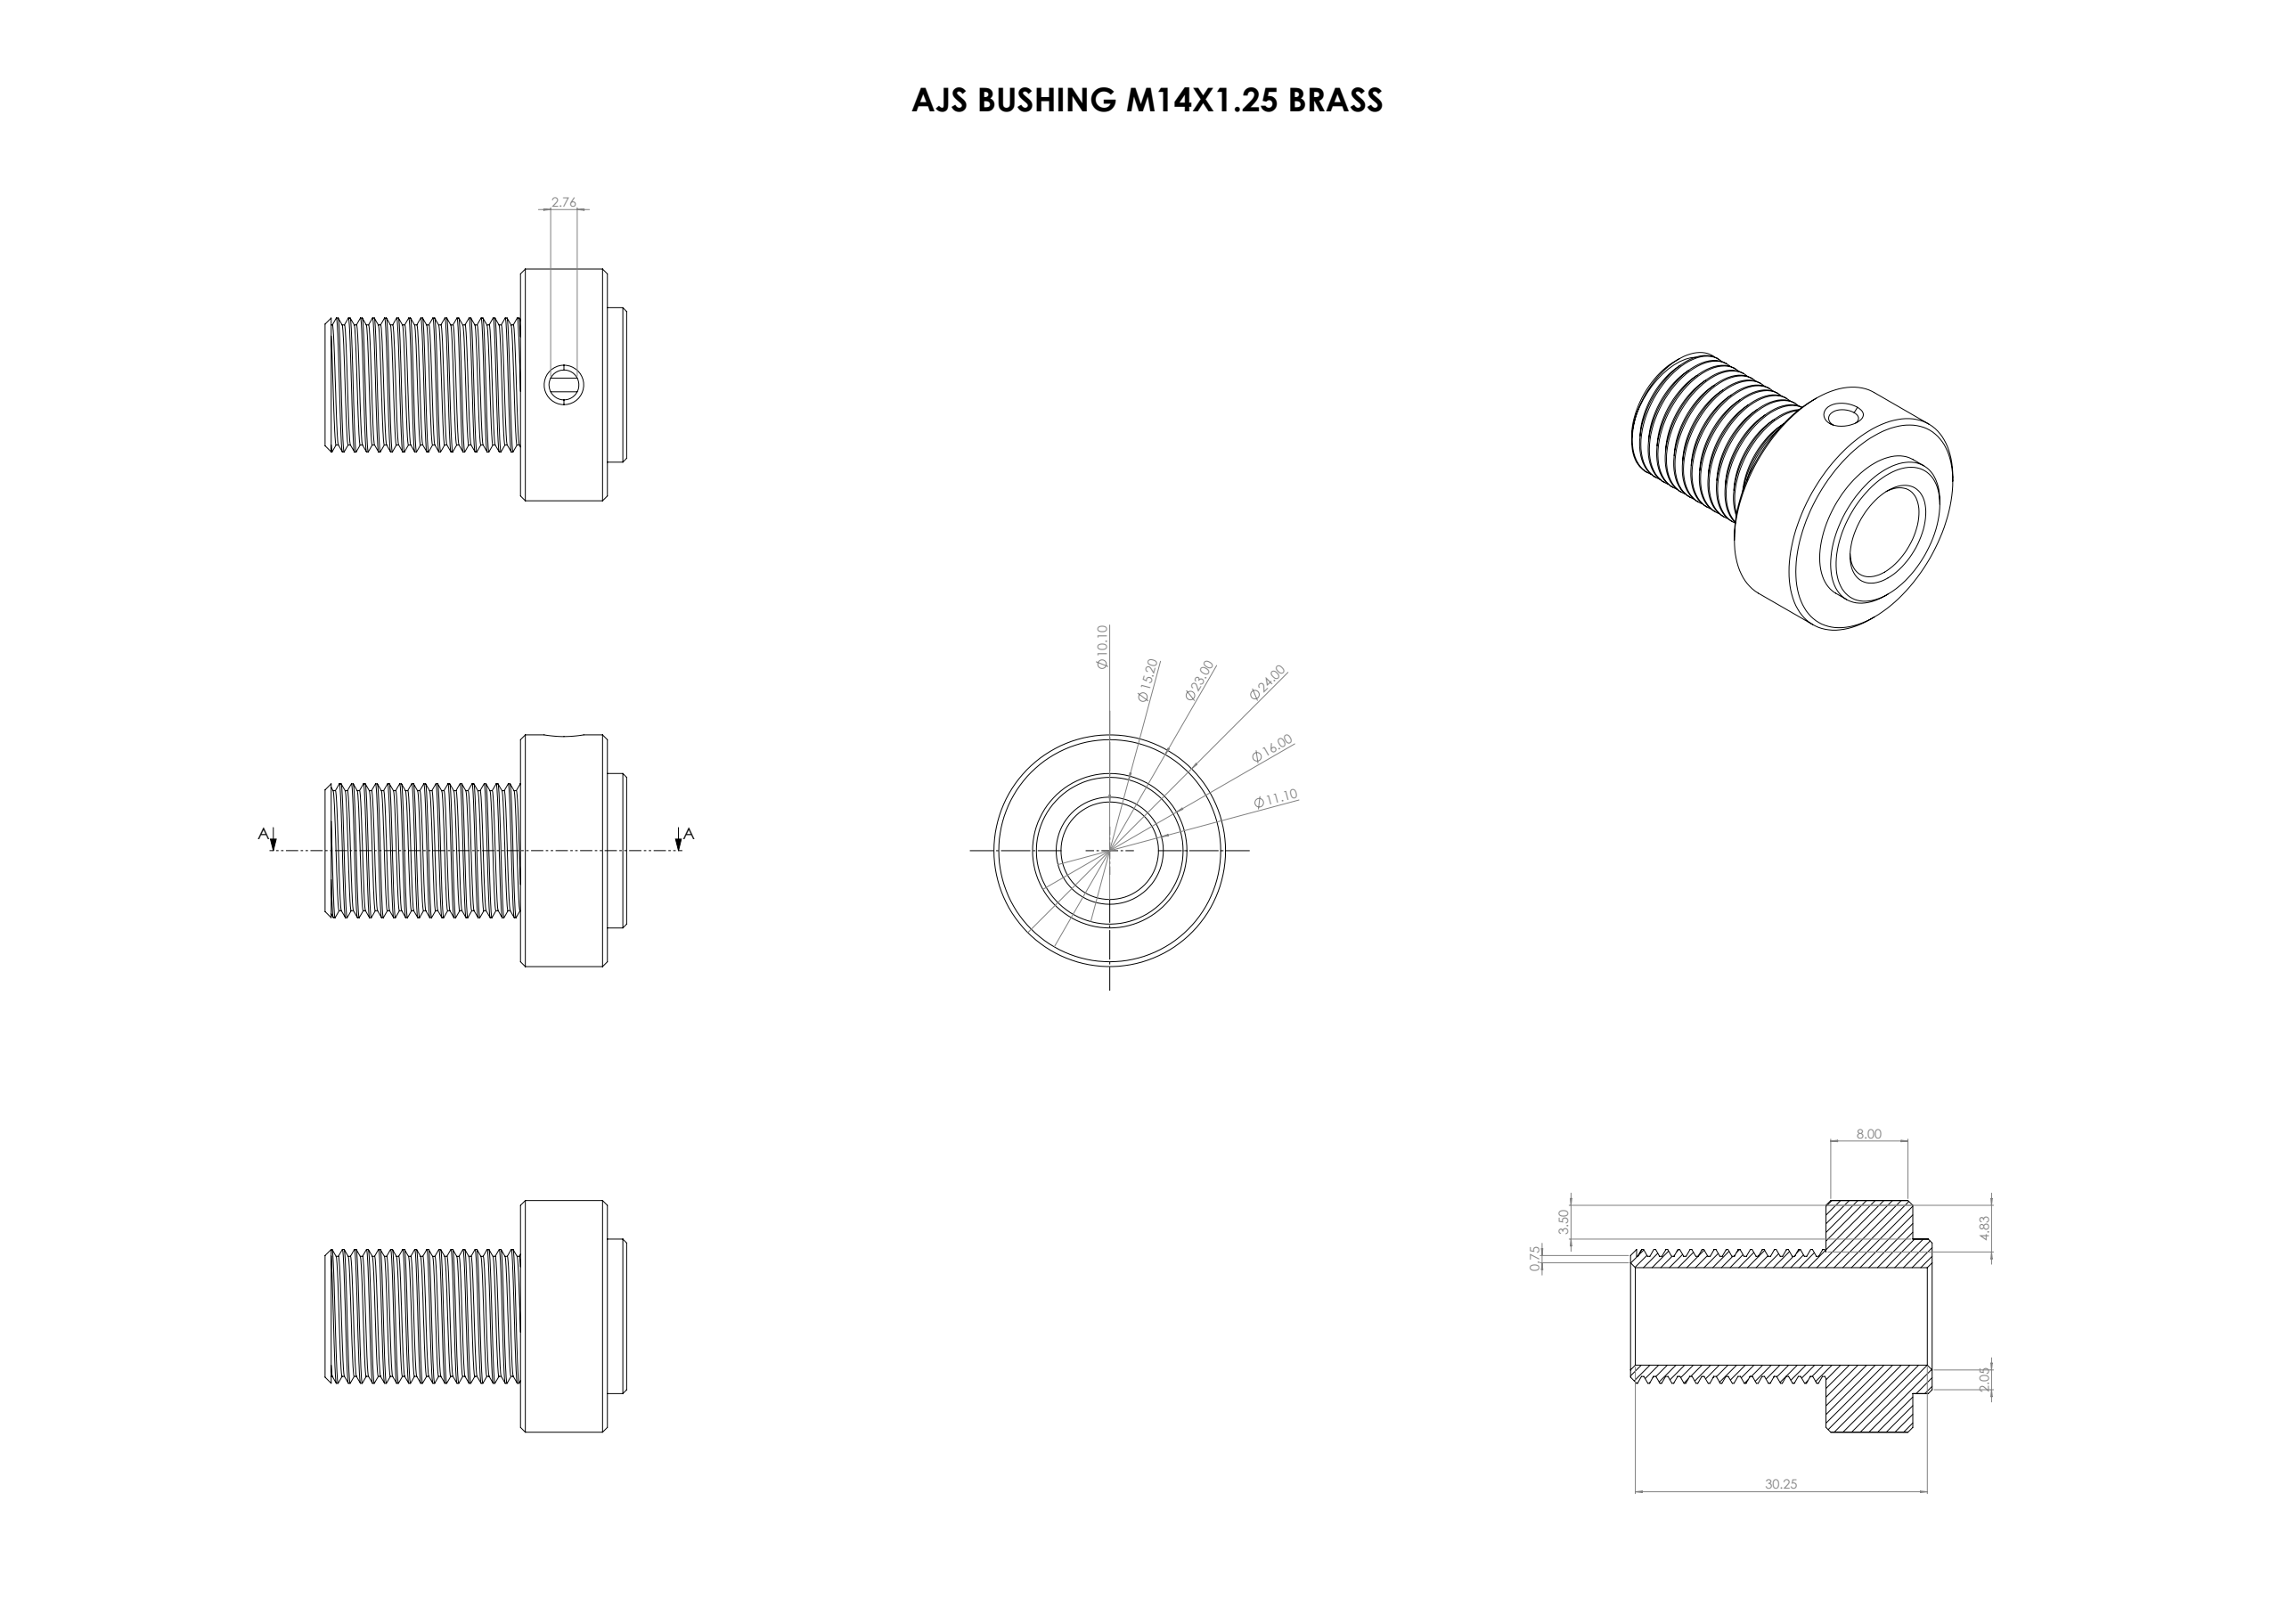
ISO-10303-21;
HEADER;
/* Generated by software containing ST-Developer
 * from STEP Tools, Inc. (www.steptools.com) 
 */

FILE_DESCRIPTION(
/* description */ (''),
/* implementation_level */ '2;1');

FILE_NAME(
/* name */ '07_AJS_Bushing_M14x1.25_Brass.step',
/* time_stamp */ '2026-10-21T01:56:51-07:00',
/* author */ (''),
/* organization */ (''),
/* preprocessor_version */ 'ST-DEVELOPER v20.2',
/* originating_system */ 'Autodesk Translation Framework v15.15.0.0',
/* authorisation */ '');

FILE_SCHEMA (('AUTOMOTIVE_DESIGN { 1 0 10303 214 3 1 1 }'));
ENDSEC;

DATA;
#10=MECHANICAL_DESIGN_GEOMETRIC_PRESENTATION_REPRESENTATION('',(#285),#82384);
#247=SHAPE_REPRESENTATION_RELATIONSHIP('SRR','None',#82481,#266);
#266=ADVANCED_BREP_SHAPE_REPRESENTATION('',(#304),#82380);
#285=STYLED_ITEM('',(#82645),#304);
#304=MANIFOLD_SOLID_BREP('Body1',#30676);
#426=B_SPLINE_SURFACE_WITH_KNOTS('',3,3,((#68020,#68021,#68022,#68023,#68024,
#68025,#68026,#68027,#68028,#68029,#68030,#68031,#68032,#68033,#68034,#68035,
#68036,#68037,#68038,#68039,#68040,#68041,#68042,#68043,#68044,#68045,#68046),
(#68047,#68048,#68049,#68050,#68051,#68052,#68053,#68054,#68055,#68056,
#68057,#68058,#68059,#68060,#68061,#68062,#68063,#68064,#68065,#68066,#68067,
#68068,#68069,#68070,#68071,#68072,#68073),(#68074,#68075,#68076,#68077,
#68078,#68079,#68080,#68081,#68082,#68083,#68084,#68085,#68086,#68087,#68088,
#68089,#68090,#68091,#68092,#68093,#68094,#68095,#68096,#68097,#68098,#68099,
#68100),(#68101,#68102,#68103,#68104,#68105,#68106,#68107,#68108,#68109,
#68110,#68111,#68112,#68113,#68114,#68115,#68116,#68117,#68118,#68119,#68120,
#68121,#68122,#68123,#68124,#68125,#68126,#68127)),.UNSPECIFIED.,.F.,.T.,
 .F.,(4,4),(4,1,2,1,1,1,2,2,2,1,1,1,1,1,1,1,1,1,1,1,4),(0.,1.),(0.,0.0584568917522064,
0.116913783504413,0.175370117903373,0.233826452302333,0.263054619501813,
0.350739121100252,0.409196012852459,0.467652904604665,0.526109517680248,
0.569951977486936,0.584566130755832,0.672251050369206,0.686865203638102,
0.69417228027255,0.701479356906998,0.774550123251477,0.818392583058164,
0.847620889595956,0.876849196133747,0.93530580920933),.UNSPECIFIED.);
#427=B_SPLINE_SURFACE_WITH_KNOTS('',3,3,((#68199,#68200,#68201,#68202,#68203,
#68204,#68205,#68206,#68207,#68208,#68209,#68210,#68211,#68212,#68213,#68214,
#68215,#68216,#68217,#68218,#68219,#68220,#68221,#68222,#68223,#68224,#68225,
#68226,#68227,#68228,#68229,#68230,#68231,#68232,#68233,#68234,#68235,#68236,
#68237,#68238,#68239,#68240,#68241,#68242,#68243,#68244,#68245,#68246,#68247,
#68248,#68249,#68250,#68251,#68252,#68253,#68254,#68255,#68256,#68257,#68258,
#68259,#68260,#68261,#68262,#68263,#68264,#68265,#68266,#68267,#68268,#68269,
#68270,#68271,#68272,#68273,#68274,#68275,#68276,#68277,#68278,#68279,#68280,
#68281,#68282,#68283,#68284,#68285,#68286,#68287,#68288,#68289,#68290,#68291,
#68292,#68293,#68294,#68295,#68296,#68297,#68298,#68299,#68300,#68301,#68302,
#68303,#68304,#68305,#68306,#68307,#68308,#68309,#68310,#68311,#68312,#68313,
#68314,#68315,#68316,#68317,#68318,#68319,#68320,#68321,#68322,#68323,#68324,
#68325,#68326,#68327,#68328,#68329,#68330,#68331,#68332,#68333,#68334,#68335,
#68336,#68337,#68338,#68339,#68340,#68341,#68342,#68343,#68344,#68345,#68346,
#68347,#68348,#68349,#68350,#68351,#68352,#68353,#68354,#68355,#68356,#68357,
#68358,#68359,#68360,#68361,#68362,#68363,#68364,#68365,#68366,#68367,#68368,
#68369,#68370,#68371,#68372,#68373,#68374,#68375,#68376,#68377,#68378,#68379,
#68380,#68381,#68382,#68383,#68384,#68385,#68386,#68387,#68388,#68389,#68390,
#68391,#68392,#68393,#68394,#68395,#68396,#68397,#68398,#68399,#68400,#68401,
#68402,#68403),(#68404,#68405,#68406,#68407,#68408,#68409,#68410,#68411,
#68412,#68413,#68414,#68415,#68416,#68417,#68418,#68419,#68420,#68421,#68422,
#68423,#68424,#68425,#68426,#68427,#68428,#68429,#68430,#68431,#68432,#68433,
#68434,#68435,#68436,#68437,#68438,#68439,#68440,#68441,#68442,#68443,#68444,
#68445,#68446,#68447,#68448,#68449,#68450,#68451,#68452,#68453,#68454,#68455,
#68456,#68457,#68458,#68459,#68460,#68461,#68462,#68463,#68464,#68465,#68466,
#68467,#68468,#68469,#68470,#68471,#68472,#68473,#68474,#68475,#68476,#68477,
#68478,#68479,#68480,#68481,#68482,#68483,#68484,#68485,#68486,#68487,#68488,
#68489,#68490,#68491,#68492,#68493,#68494,#68495,#68496,#68497,#68498,#68499,
#68500,#68501,#68502,#68503,#68504,#68505,#68506,#68507,#68508,#68509,#68510,
#68511,#68512,#68513,#68514,#68515,#68516,#68517,#68518,#68519,#68520,#68521,
#68522,#68523,#68524,#68525,#68526,#68527,#68528,#68529,#68530,#68531,#68532,
#68533,#68534,#68535,#68536,#68537,#68538,#68539,#68540,#68541,#68542,#68543,
#68544,#68545,#68546,#68547,#68548,#68549,#68550,#68551,#68552,#68553,#68554,
#68555,#68556,#68557,#68558,#68559,#68560,#68561,#68562,#68563,#68564,#68565,
#68566,#68567,#68568,#68569,#68570,#68571,#68572,#68573,#68574,#68575,#68576,
#68577,#68578,#68579,#68580,#68581,#68582,#68583,#68584,#68585,#68586,#68587,
#68588,#68589,#68590,#68591,#68592,#68593,#68594,#68595,#68596,#68597,#68598,
#68599,#68600,#68601,#68602,#68603,#68604,#68605,#68606,#68607,#68608),
(#68609,#68610,#68611,#68612,#68613,#68614,#68615,#68616,#68617,#68618,
#68619,#68620,#68621,#68622,#68623,#68624,#68625,#68626,#68627,#68628,#68629,
#68630,#68631,#68632,#68633,#68634,#68635,#68636,#68637,#68638,#68639,#68640,
#68641,#68642,#68643,#68644,#68645,#68646,#68647,#68648,#68649,#68650,#68651,
#68652,#68653,#68654,#68655,#68656,#68657,#68658,#68659,#68660,#68661,#68662,
#68663,#68664,#68665,#68666,#68667,#68668,#68669,#68670,#68671,#68672,#68673,
#68674,#68675,#68676,#68677,#68678,#68679,#68680,#68681,#68682,#68683,#68684,
#68685,#68686,#68687,#68688,#68689,#68690,#68691,#68692,#68693,#68694,#68695,
#68696,#68697,#68698,#68699,#68700,#68701,#68702,#68703,#68704,#68705,#68706,
#68707,#68708,#68709,#68710,#68711,#68712,#68713,#68714,#68715,#68716,#68717,
#68718,#68719,#68720,#68721,#68722,#68723,#68724,#68725,#68726,#68727,#68728,
#68729,#68730,#68731,#68732,#68733,#68734,#68735,#68736,#68737,#68738,#68739,
#68740,#68741,#68742,#68743,#68744,#68745,#68746,#68747,#68748,#68749,#68750,
#68751,#68752,#68753,#68754,#68755,#68756,#68757,#68758,#68759,#68760,#68761,
#68762,#68763,#68764,#68765,#68766,#68767,#68768,#68769,#68770,#68771,#68772,
#68773,#68774,#68775,#68776,#68777,#68778,#68779,#68780,#68781,#68782,#68783,
#68784,#68785,#68786,#68787,#68788,#68789,#68790,#68791,#68792,#68793,#68794,
#68795,#68796,#68797,#68798,#68799,#68800,#68801,#68802,#68803,#68804,#68805,
#68806,#68807,#68808,#68809,#68810,#68811,#68812,#68813),(#68814,#68815,
#68816,#68817,#68818,#68819,#68820,#68821,#68822,#68823,#68824,#68825,#68826,
#68827,#68828,#68829,#68830,#68831,#68832,#68833,#68834,#68835,#68836,#68837,
#68838,#68839,#68840,#68841,#68842,#68843,#68844,#68845,#68846,#68847,#68848,
#68849,#68850,#68851,#68852,#68853,#68854,#68855,#68856,#68857,#68858,#68859,
#68860,#68861,#68862,#68863,#68864,#68865,#68866,#68867,#68868,#68869,#68870,
#68871,#68872,#68873,#68874,#68875,#68876,#68877,#68878,#68879,#68880,#68881,
#68882,#68883,#68884,#68885,#68886,#68887,#68888,#68889,#68890,#68891,#68892,
#68893,#68894,#68895,#68896,#68897,#68898,#68899,#68900,#68901,#68902,#68903,
#68904,#68905,#68906,#68907,#68908,#68909,#68910,#68911,#68912,#68913,#68914,
#68915,#68916,#68917,#68918,#68919,#68920,#68921,#68922,#68923,#68924,#68925,
#68926,#68927,#68928,#68929,#68930,#68931,#68932,#68933,#68934,#68935,#68936,
#68937,#68938,#68939,#68940,#68941,#68942,#68943,#68944,#68945,#68946,#68947,
#68948,#68949,#68950,#68951,#68952,#68953,#68954,#68955,#68956,#68957,#68958,
#68959,#68960,#68961,#68962,#68963,#68964,#68965,#68966,#68967,#68968,#68969,
#68970,#68971,#68972,#68973,#68974,#68975,#68976,#68977,#68978,#68979,#68980,
#68981,#68982,#68983,#68984,#68985,#68986,#68987,#68988,#68989,#68990,#68991,
#68992,#68993,#68994,#68995,#68996,#68997,#68998,#68999,#69000,#69001,#69002,
#69003,#69004,#69005,#69006,#69007,#69008,#69009,#69010,#69011,#69012,#69013,
#69014,#69015,#69016,#69017,#69018)),.UNSPECIFIED.,.F.,.F.,.F.,(4,4),(4,
1,1,1,1,1,1,1,1,1,1,1,1,1,1,1,1,1,1,1,1,1,1,1,1,1,1,1,1,1,1,1,1,1,1,1,1,
1,1,1,1,1,1,1,1,1,1,1,1,1,1,1,1,1,1,1,1,1,1,1,1,1,1,1,1,1,1,1,1,1,1,1,1,
1,1,1,1,1,1,1,1,1,1,1,1,1,1,1,1,1,1,1,1,1,1,1,1,1,1,1,1,1,1,1,1,1,1,1,1,
1,1,1,1,1,1,1,1,1,1,1,1,1,1,1,1,1,1,1,1,1,1,1,1,1,1,1,1,1,1,1,1,1,1,1,1,
1,1,1,1,1,1,1,1,1,1,1,1,1,1,1,1,1,1,1,1,1,1,1,1,1,1,1,1,1,1,1,1,1,1,1,1,
1,1,1,1,1,1,1,1,1,1,1,1,1,1,1,1,1,1,1,1,1,4),(0.,0.0824167509268191),(8.30472057736738,
8.80312233880653,9.30152410024569,9.79992586168484,10.298327623124,10.7967293845631,
11.2951311460023,11.7935329074415,12.2919346688806,12.7903364303198,13.2887381917589,
13.7871399531981,14.2855417146372,14.7839434760764,15.2823452375155,15.7807469989547,
16.2791487603938,16.777550521833,17.2759522832721,17.7743540447113,18.2727558061505,
18.7711575675896,19.2695593290288,19.7679610904679,20.2663628519071,20.7647646133462,
21.2631663747854,21.7615681362245,22.2599698976637,22.7583716591028,23.256773420542,
23.7551751819811,24.2535769434203,24.7519787048595,25.2503804662986,25.7487822277378,
26.2471839891769,26.7455857506161,27.2439875120552,27.7423892734944,28.2407910349335,
28.7391927963727,29.2375945578118,29.735996319251,30.2343980806901,30.7327998421293,
31.2312016035684,31.7296033650076,32.2280051264468,32.7264068878859,33.2248086493251,
33.7232104107642,34.2216121722034,34.7200139336425,35.2184156950817,35.7168174565208,
36.21521921796,36.7136209793991,37.2120227408383,37.7104245022774,38.2088262637166,
38.7072280251558,39.2056297865949,39.7040315480341,40.2024333094732,40.7008350709124,
41.1992368323515,41.6976385937907,42.1960403552298,42.694442116669,43.1928438781081,
43.6912456395473,44.1896474009864,44.6880491624256,45.1864509238648,45.6848526853039,
46.1832544467431,46.6816562081822,47.1800579696214,47.6784597310605,48.1768614924997,
48.6752632539388,49.173665015378,49.6720667768171,50.1704685382563,50.6688702996954,
51.1672720611346,51.6656738225738,52.1640755840129,52.6624773454521,53.1608791068912,
53.6592808683304,54.1576826297695,54.6560843912087,55.1544861526478,55.652887914087,
56.1512896755261,56.6496914369653,57.1480931984044,57.6464949598436,58.1448967212827,
58.6432984827219,59.1417002441611,59.6401020056002,60.1385037670394,60.6369055284785,
61.1353072899177,61.6337090513568,62.132110812796,62.6305125742351,63.1289143356743,
63.6273160971134,64.1257178585526,64.6241196199917,65.1225213814309,65.6209231428701,
66.1193249043092,66.6177266657484,67.1161284271875,67.6145301886267,68.1129319500658,
68.611333711505,69.1097354729441,69.6081372343833,70.1065389958224,70.6049407572616,
71.1033425187007,71.6017442801399,72.1001460415791,72.5985478030182,73.0969495644573,
73.5953513258965,74.0937530873357,74.5921548487748,75.090556610214,75.5889583716531,
76.0873601330923,76.5857618945314,77.0841636559706,77.5825654174097,78.0809671788489,
78.579368940288,79.0777707017272,79.5761724631663,80.0745742246055,80.5729759860447,
81.0713777474838,81.569779508923,82.0681812703621,82.5665830318013,83.0649847932404,
83.5633865546796,84.0617883161187,84.5601900775579,85.058591838997,85.5569936004362,
86.0553953618753,86.5537971233145,87.0521988847537,87.5506006461928,88.049002407632,
88.5474041690711,89.0458059305103,89.5442076919494,90.0426094533886,90.5410112148277,
91.0394129762669,91.537814737706,92.0362164991452,92.5346182605844,93.0330200220235,
93.5314217834626,94.0298235449018,94.528225306341,95.0266270677801,95.5250288292193,
96.0234305906584,96.5218323520976,97.0202341135367,97.5186358749759,98.017037636415,
98.5154393978542,99.0138411592933,99.5122429207325,100.010644682172,100.509046443611,
101.00744820505,101.505849966489,102.004251727928,102.502653489367,103.001055250807,
103.499457012246,103.997858773685,104.496260535124,104.994662296563,105.493064058002,
105.991465819441,106.489867580881,106.98826934232,107.486671103759,107.985072865198,
108.483474626637,108.981876388076),.UNSPECIFIED.);
#428=B_SPLINE_SURFACE_WITH_KNOTS('',3,3,((#69418,#69419,#69420,#69421,#69422,
#69423,#69424,#69425,#69426,#69427,#69428,#69429,#69430,#69431,#69432,#69433,
#69434,#69435,#69436,#69437,#69438,#69439,#69440,#69441,#69442,#69443,#69444,
#69445,#69446,#69447,#69448,#69449,#69450,#69451,#69452,#69453,#69454,#69455,
#69456,#69457,#69458,#69459,#69460,#69461,#69462,#69463,#69464,#69465,#69466,
#69467,#69468,#69469,#69470,#69471,#69472,#69473,#69474,#69475,#69476,#69477,
#69478,#69479,#69480,#69481,#69482,#69483,#69484,#69485,#69486,#69487,#69488,
#69489,#69490,#69491,#69492,#69493,#69494,#69495,#69496,#69497,#69498,#69499,
#69500,#69501,#69502,#69503,#69504,#69505,#69506,#69507,#69508,#69509,#69510,
#69511,#69512,#69513,#69514,#69515,#69516,#69517,#69518,#69519,#69520,#69521,
#69522,#69523,#69524,#69525,#69526,#69527,#69528,#69529,#69530,#69531,#69532,
#69533,#69534,#69535,#69536,#69537,#69538,#69539,#69540,#69541,#69542,#69543,
#69544,#69545,#69546,#69547,#69548,#69549,#69550,#69551,#69552,#69553,#69554,
#69555,#69556,#69557,#69558,#69559,#69560,#69561,#69562,#69563,#69564,#69565,
#69566,#69567,#69568,#69569,#69570,#69571,#69572,#69573,#69574,#69575,#69576,
#69577,#69578,#69579,#69580,#69581,#69582,#69583,#69584,#69585,#69586,#69587,
#69588,#69589,#69590,#69591,#69592,#69593,#69594,#69595,#69596,#69597,#69598,
#69599,#69600,#69601,#69602,#69603,#69604,#69605,#69606,#69607,#69608,#69609,
#69610,#69611,#69612,#69613,#69614,#69615,#69616,#69617,#69618,#69619,#69620,
#69621,#69622),(#69623,#69624,#69625,#69626,#69627,#69628,#69629,#69630,
#69631,#69632,#69633,#69634,#69635,#69636,#69637,#69638,#69639,#69640,#69641,
#69642,#69643,#69644,#69645,#69646,#69647,#69648,#69649,#69650,#69651,#69652,
#69653,#69654,#69655,#69656,#69657,#69658,#69659,#69660,#69661,#69662,#69663,
#69664,#69665,#69666,#69667,#69668,#69669,#69670,#69671,#69672,#69673,#69674,
#69675,#69676,#69677,#69678,#69679,#69680,#69681,#69682,#69683,#69684,#69685,
#69686,#69687,#69688,#69689,#69690,#69691,#69692,#69693,#69694,#69695,#69696,
#69697,#69698,#69699,#69700,#69701,#69702,#69703,#69704,#69705,#69706,#69707,
#69708,#69709,#69710,#69711,#69712,#69713,#69714,#69715,#69716,#69717,#69718,
#69719,#69720,#69721,#69722,#69723,#69724,#69725,#69726,#69727,#69728,#69729,
#69730,#69731,#69732,#69733,#69734,#69735,#69736,#69737,#69738,#69739,#69740,
#69741,#69742,#69743,#69744,#69745,#69746,#69747,#69748,#69749,#69750,#69751,
#69752,#69753,#69754,#69755,#69756,#69757,#69758,#69759,#69760,#69761,#69762,
#69763,#69764,#69765,#69766,#69767,#69768,#69769,#69770,#69771,#69772,#69773,
#69774,#69775,#69776,#69777,#69778,#69779,#69780,#69781,#69782,#69783,#69784,
#69785,#69786,#69787,#69788,#69789,#69790,#69791,#69792,#69793,#69794,#69795,
#69796,#69797,#69798,#69799,#69800,#69801,#69802,#69803,#69804,#69805,#69806,
#69807,#69808,#69809,#69810,#69811,#69812,#69813,#69814,#69815,#69816,#69817,
#69818,#69819,#69820,#69821,#69822,#69823,#69824,#69825,#69826,#69827),
(#69828,#69829,#69830,#69831,#69832,#69833,#69834,#69835,#69836,#69837,
#69838,#69839,#69840,#69841,#69842,#69843,#69844,#69845,#69846,#69847,#69848,
#69849,#69850,#69851,#69852,#69853,#69854,#69855,#69856,#69857,#69858,#69859,
#69860,#69861,#69862,#69863,#69864,#69865,#69866,#69867,#69868,#69869,#69870,
#69871,#69872,#69873,#69874,#69875,#69876,#69877,#69878,#69879,#69880,#69881,
#69882,#69883,#69884,#69885,#69886,#69887,#69888,#69889,#69890,#69891,#69892,
#69893,#69894,#69895,#69896,#69897,#69898,#69899,#69900,#69901,#69902,#69903,
#69904,#69905,#69906,#69907,#69908,#69909,#69910,#69911,#69912,#69913,#69914,
#69915,#69916,#69917,#69918,#69919,#69920,#69921,#69922,#69923,#69924,#69925,
#69926,#69927,#69928,#69929,#69930,#69931,#69932,#69933,#69934,#69935,#69936,
#69937,#69938,#69939,#69940,#69941,#69942,#69943,#69944,#69945,#69946,#69947,
#69948,#69949,#69950,#69951,#69952,#69953,#69954,#69955,#69956,#69957,#69958,
#69959,#69960,#69961,#69962,#69963,#69964,#69965,#69966,#69967,#69968,#69969,
#69970,#69971,#69972,#69973,#69974,#69975,#69976,#69977,#69978,#69979,#69980,
#69981,#69982,#69983,#69984,#69985,#69986,#69987,#69988,#69989,#69990,#69991,
#69992,#69993,#69994,#69995,#69996,#69997,#69998,#69999,#70000,#70001,#70002,
#70003,#70004,#70005,#70006,#70007,#70008,#70009,#70010,#70011,#70012,#70013,
#70014,#70015,#70016,#70017,#70018,#70019,#70020,#70021,#70022,#70023,#70024,
#70025,#70026,#70027,#70028,#70029,#70030,#70031,#70032),(#70033,#70034,
#70035,#70036,#70037,#70038,#70039,#70040,#70041,#70042,#70043,#70044,#70045,
#70046,#70047,#70048,#70049,#70050,#70051,#70052,#70053,#70054,#70055,#70056,
#70057,#70058,#70059,#70060,#70061,#70062,#70063,#70064,#70065,#70066,#70067,
#70068,#70069,#70070,#70071,#70072,#70073,#70074,#70075,#70076,#70077,#70078,
#70079,#70080,#70081,#70082,#70083,#70084,#70085,#70086,#70087,#70088,#70089,
#70090,#70091,#70092,#70093,#70094,#70095,#70096,#70097,#70098,#70099,#70100,
#70101,#70102,#70103,#70104,#70105,#70106,#70107,#70108,#70109,#70110,#70111,
#70112,#70113,#70114,#70115,#70116,#70117,#70118,#70119,#70120,#70121,#70122,
#70123,#70124,#70125,#70126,#70127,#70128,#70129,#70130,#70131,#70132,#70133,
#70134,#70135,#70136,#70137,#70138,#70139,#70140,#70141,#70142,#70143,#70144,
#70145,#70146,#70147,#70148,#70149,#70150,#70151,#70152,#70153,#70154,#70155,
#70156,#70157,#70158,#70159,#70160,#70161,#70162,#70163,#70164,#70165,#70166,
#70167,#70168,#70169,#70170,#70171,#70172,#70173,#70174,#70175,#70176,#70177,
#70178,#70179,#70180,#70181,#70182,#70183,#70184,#70185,#70186,#70187,#70188,
#70189,#70190,#70191,#70192,#70193,#70194,#70195,#70196,#70197,#70198,#70199,
#70200,#70201,#70202,#70203,#70204,#70205,#70206,#70207,#70208,#70209,#70210,
#70211,#70212,#70213,#70214,#70215,#70216,#70217,#70218,#70219,#70220,#70221,
#70222,#70223,#70224,#70225,#70226,#70227,#70228,#70229,#70230,#70231,#70232,
#70233,#70234,#70235,#70236,#70237)),.UNSPECIFIED.,.F.,.F.,.F.,(4,4),(4,
1,1,1,1,1,1,1,1,1,1,1,1,1,1,1,1,1,1,1,1,1,1,1,1,1,1,1,1,1,1,1,1,1,1,1,1,
1,1,1,1,1,1,1,1,1,1,1,1,1,1,1,1,1,1,1,1,1,1,1,1,1,1,1,1,1,1,1,1,1,1,1,1,
1,1,1,1,1,1,1,1,1,1,1,1,1,1,1,1,1,1,1,1,1,1,1,1,1,1,1,1,1,1,1,1,1,1,1,1,
1,1,1,1,1,1,1,1,1,1,1,1,1,1,1,1,1,1,1,1,1,1,1,1,1,1,1,1,1,1,1,1,1,1,1,1,
1,1,1,1,1,1,1,1,1,1,1,1,1,1,1,1,1,1,1,1,1,1,1,1,1,1,1,1,1,1,1,1,1,1,1,1,
1,1,1,1,1,1,1,1,1,1,1,1,1,1,1,1,1,1,1,1,1,4),(0.,0.0824167509268191),(11.6150691238055,
12.1134708852447,12.6118726466838,13.110274408123,13.6086761695621,14.1070779310013,
14.6054796924404,15.1038814538796,15.6022832153187,16.1006849767579,16.5990867381971,
17.0974884996362,17.5958902610754,18.0942920225145,18.5926937839537,19.0910955453928,
19.589497306832,20.0878990682711,20.5863008297103,21.0847025911494,21.5831043525886,
22.0815061140277,22.5799078754669,23.0783096369061,23.5767113983452,24.0751131597844,
24.5735149212235,25.0719166826627,25.5703184441018,26.068720205541,26.5671219669801,
27.0655237284193,27.5639254898584,28.0623272512976,28.5607290127367,29.0591307741759,
29.5575325356151,30.0559342970542,30.5543360584934,31.0527378199325,31.5511395813717,
32.0495413428108,32.54794310425,33.0463448656891,33.5447466271283,34.0431483885674,
34.5415501500066,35.0399519114457,35.5383536728849,36.036755434324,36.5351571957632,
37.0335589572024,37.5319607186415,38.0303624800807,38.5287642415198,39.027166002959,
39.5255677643981,40.0239695258373,40.5223712872764,41.0207730487156,41.5191748101547,
42.0175765715939,42.515978333033,43.0143800944722,43.5127818559113,44.0111836173505,
44.5095853787897,45.0079871402288,45.506388901668,46.0047906631071,46.5031924245463,
47.0015941859854,47.4999959474246,47.9983977088637,48.4967994703029,48.995201231742,
49.4936029931812,49.9920047546203,50.4904065160595,50.9888082774987,51.4872100389378,
51.985611800377,52.4840135618161,52.9824153232553,53.4808170846944,53.9792188461336,
54.4776206075727,54.9760223690119,55.474424130451,55.9728258918902,56.4712276533293,
56.9696294147685,57.4680311762077,57.9664329376468,58.464834699086,58.9632364605251,
59.4616382219643,59.9600399834034,60.4584417448426,60.9568435062817,61.4552452677209,
61.95364702916,62.4520487905992,62.9504505520383,63.4488523134775,63.9472540749166,
64.4456558363558,64.944057597795,65.4424593592341,65.9408611206733,66.4392628821124,
66.9376646435516,67.4360664049907,67.9344681664299,68.432869927869,68.9312716893082,
69.4296734507473,69.9280752121865,70.4264769736257,70.9248787350648,71.4232804965039,
71.9216822579431,72.4200840193823,72.9184857808214,73.4168875422606,73.9152893036997,
74.4136910651389,74.912092826578,75.4104945880172,75.9088963494563,76.4072981108955,
76.9056998723347,77.4041016337738,77.902503395213,78.4009051566521,78.8993069180913,
79.3977086795304,79.8961104409696,80.3945122024087,80.8929139638479,81.391315725287,
81.8897174867262,82.3881192481653,82.8865210096045,83.3849227710436,83.8833245324828,
84.381726293922,84.8801280553611,85.3785298168003,85.8769315782394,86.3753333396786,
86.8737351011177,87.3721368625569,87.870538623996,88.3689403854352,88.8673421468743,
89.3657439083135,89.8641456697526,90.3625474311918,90.860949192631,91.3593509540701,
91.8577527155093,92.3561544769484,92.8545562383876,93.3529579998267,93.8513597612659,
94.349761522705,94.8481632841442,95.3465650455833,95.8449668070225,96.3433685684616,
96.8417703299008,97.34017209134,97.8385738527791,98.3369756142182,98.8353773756574,
99.3337791370966,99.8321808985357,100.330582659975,100.828984421414,101.327386182853,
101.825787944292,102.324189705731,102.822591467171,103.32099322861,103.819394990049,
104.317796751488,104.816198512927,105.314600274366,105.813002035806,106.311403797245,
106.809805558684,107.308207320123,107.806609081562,108.305010843001,108.80341260444,
109.30181436588,109.800216127319,110.298617888758,110.797019650197,111.295421411636,
111.793823173075,112.292224934515),.UNSPECIFIED.);
#812=CYLINDRICAL_SURFACE('',#32908,6.933);
#813=CYLINDRICAL_SURFACE('',#32910,6.933);
#814=CYLINDRICAL_SURFACE('',#32911,6.933);
#815=CYLINDRICAL_SURFACE('',#32912,6.933);
#816=CYLINDRICAL_SURFACE('',#32913,6.933);
#817=CYLINDRICAL_SURFACE('',#32914,6.933);
#818=CYLINDRICAL_SURFACE('',#32915,6.933);
#819=CYLINDRICAL_SURFACE('',#32916,6.933);
#820=CYLINDRICAL_SURFACE('',#32917,6.933);
#821=CYLINDRICAL_SURFACE('',#32918,6.933);
#822=CYLINDRICAL_SURFACE('',#32919,6.933);
#823=CYLINDRICAL_SURFACE('',#32920,6.933);
#824=CYLINDRICAL_SURFACE('',#32921,6.933);
#825=CYLINDRICAL_SURFACE('',#32922,6.933);
#826=CYLINDRICAL_SURFACE('',#32923,6.933);
#827=CYLINDRICAL_SURFACE('',#32924,6.933);
#828=CYLINDRICAL_SURFACE('',#32925,6.21925);
#829=CYLINDRICAL_SURFACE('',#32927,6.21925);
#830=CYLINDRICAL_SURFACE('',#32929,6.21925);
#831=CYLINDRICAL_SURFACE('',#32930,6.21925);
#832=CYLINDRICAL_SURFACE('',#32931,6.21925);
#833=CYLINDRICAL_SURFACE('',#32932,6.21925);
#834=CYLINDRICAL_SURFACE('',#32933,6.21925);
#835=CYLINDRICAL_SURFACE('',#32934,6.21925);
#836=CYLINDRICAL_SURFACE('',#32935,6.21925);
#837=CYLINDRICAL_SURFACE('',#32936,6.21925);
#838=CYLINDRICAL_SURFACE('',#32937,6.21925);
#839=CYLINDRICAL_SURFACE('',#32938,6.21925);
#840=CYLINDRICAL_SURFACE('',#32939,6.21925);
#841=CYLINDRICAL_SURFACE('',#32940,6.21925);
#842=CYLINDRICAL_SURFACE('',#32941,6.21925);
#843=CYLINDRICAL_SURFACE('',#32942,6.21925);
#844=CYLINDRICAL_SURFACE('',#32947,5.05);
#845=CYLINDRICAL_SURFACE('',#32956,1.55);
#846=CYLINDRICAL_SURFACE('',#32959,12.);
#847=CYLINDRICAL_SURFACE('',#32966,6.21925);
#848=CYLINDRICAL_SURFACE('',#32970,6.933);
#849=CYLINDRICAL_SURFACE('',#32979,8.);
#1742=CIRCLE('',#32909,6.933);
#1743=CIRCLE('',#32926,6.21925);
#1744=CIRCLE('',#32928,6.21925);
#1745=CIRCLE('',#32944,5.55);
#1746=CIRCLE('',#32945,5.05);
#1747=CIRCLE('',#32946,5.05);
#1748=CIRCLE('',#32948,5.05);
#1749=CIRCLE('',#32949,5.05);
#1750=CIRCLE('',#32951,6.3);
#1751=CIRCLE('',#32953,5.55);
#1752=CIRCLE('',#32955,7.6);
#1753=CIRCLE('',#32957,1.55);
#1754=CIRCLE('',#32958,1.55);
#1755=CIRCLE('',#32960,12.);
#1756=CIRCLE('',#32961,12.);
#1757=CIRCLE('',#32963,6.933);
#1758=CIRCLE('',#32964,6.933);
#1759=CIRCLE('',#32965,6.21925);
#1760=CIRCLE('',#32971,6.933);
#1761=CIRCLE('',#32973,11.5);
#1762=CIRCLE('',#32976,11.5);
#1763=CIRCLE('',#32978,8.);
#1764=CIRCLE('',#32980,8.);
#2055=CONICAL_SURFACE('',#32943,5.3,0.785398163397448);
#2056=CONICAL_SURFACE('',#32952,5.3,0.785398163397448);
#2057=CONICAL_SURFACE('',#32969,6.65,0.785398163397447);
#2058=CONICAL_SURFACE('',#32974,11.75,0.785398163397448);
#2059=CONICAL_SURFACE('',#32975,11.75,0.785398163397448);
#2060=CONICAL_SURFACE('',#32981,7.8,0.785398163397451);
#2835=B_SPLINE_CURVE_WITH_KNOTS('',3,(#66057,#66058,#66059,#66060,#66061,
#66062,#66063,#66064,#66065,#66066,#66067,#66068,#66069,#66070,#66071,#66072),
 .UNSPECIFIED.,.F.,.F.,(4,3,3,3,3,4),(-4.09289414414337,-3.98721409151323,
-3.48881233007407,-2.99041056863492,-2.49200880719577,-2.07135887395549),
 .UNSPECIFIED.);
#2836=B_SPLINE_CURVE_WITH_KNOTS('',3,(#66075,#66076,#66077,#66078,#66079,
#66080,#66081,#66082,#66083,#66084),.UNSPECIFIED.,.F.,.F.,(4,3,3,4),(0.,
0.498401761439146,0.996803522878299,1.12005738340184),.UNSPECIFIED.);
#2837=B_SPLINE_CURVE_WITH_KNOTS('',3,(#66089,#66090,#66091,#66092,#66093,
#66094,#66095,#66096,#66097,#66098,#66099,#66100,#66101,#66102,#66103,#66104,
#66105,#66106,#66107,#66108,#66109,#66110,#66111,#66112,#66113,#66114,#66115,
#66116,#66117,#66118,#66119,#66120,#66121,#66122,#66123,#66124,#66125,#66126,
#66127,#66128),.UNSPECIFIED.,.F.,.F.,(4,3,3,3,3,3,3,3,3,3,3,3,3,4),(-10.376079451323,
-9.96803522878307,-9.46963346734392,-8.97123170590477,-8.47282994446562,
-7.97442818302646,-7.47602642158731,-6.97762466014815,-6.479222898709,-5.98082113726984,
-5.48241937583069,-4.98401761439154,-4.48561585295238,-4.09289414414337),
 .UNSPECIFIED.);
#2838=B_SPLINE_CURVE_WITH_KNOTS('',3,(#66129,#66130,#66131,#66132,#66133,
#66134,#66135,#66136,#66137,#66138,#66139,#66140,#66141,#66142,#66143,#66144,
#66145,#66146,#66147,#66148,#66149,#66150,#66151,#66152,#66153,#66154,#66155,
#66156,#66157,#66158,#66159,#66160,#66161,#66162,#66163,#66164,#66165,#66166,
#66167,#66168),.UNSPECIFIED.,.F.,.F.,(4,3,3,3,3,3,3,3,3,3,3,3,3,4),(1.12005738340184,
1.49520528431745,1.99360704575661,2.49200880719576,2.99041056863492,3.48881233007407,
3.98721409151323,4.48561585295238,4.98401761439154,5.48241937583069,5.98082113726985,
6.479222898709,6.97762466014816,7.40324269058142),.UNSPECIFIED.);
#2839=B_SPLINE_CURVE_WITH_KNOTS('',3,(#66173,#66174,#66175,#66176,#66177,
#66178,#66179,#66180,#66181,#66182,#66183,#66184,#66185,#66186,#66187,#66188,
#66189,#66190,#66191,#66192,#66193,#66194,#66195,#66196,#66197,#66198,#66199,
#66200,#66201,#66202,#66203,#66204,#66205,#66206,#66207,#66208,#66209,#66210,
#66211,#66212,#66213,#66214,#66215),.UNSPECIFIED.,.F.,.F.,(4,3,3,3,3,3,
3,3,3,3,3,3,3,3,4),(-16.6592647585025,-16.4472581274921,-15.9488563660529,
-15.4504546046138,-14.9520528431746,-14.4536510817355,-13.9552493202963,
-13.4568475588571,-12.958445797418,-12.4600440359788,-11.9616422745397,
-11.4632405131005,-10.9648387516614,-10.4664369902222,-10.376079451323),
 .UNSPECIFIED.);
#2840=B_SPLINE_CURVE_WITH_KNOTS('',3,(#66216,#66217,#66218,#66219,#66220,
#66221,#66222,#66223,#66224,#66225,#66226,#66227,#66228,#66229,#66230,#66231,
#66232,#66233,#66234,#66235,#66236,#66237,#66238,#66239,#66240,#66241,#66242,
#66243,#66244,#66245,#66246,#66247,#66248,#66249,#66250,#66251,#66252,#66253,
#66254,#66255,#66256,#66257,#66258),.UNSPECIFIED.,.F.,.F.,(4,3,3,3,3,3,
3,3,3,3,3,3,3,3,4),(7.40324269058142,7.47602642158731,7.97442818302646,
8.47282994446562,8.97123170590477,9.46963346734393,9.96803522878308,10.4664369902222,
10.9648387516614,11.4632405131005,11.9616422745397,12.4600440359788,12.958445797418,
13.4568475588571,13.686427997761),.UNSPECIFIED.);
#2841=B_SPLINE_CURVE_WITH_KNOTS('',3,(#66263,#66264,#66265,#66266,#66267,
#66268,#66269,#66270,#66271,#66272,#66273,#66274,#66275,#66276,#66277,#66278,
#66279,#66280,#66281,#66282,#66283,#66284,#66285,#66286,#66287,#66288,#66289,
#66290,#66291,#66292,#66293,#66294,#66295,#66296,#66297,#66298,#66299,#66300,
#66301,#66302,#66303,#66304,#66305),.UNSPECIFIED.,.F.,.F.,(4,3,3,3,3,3,
3,3,3,3,3,3,3,3,4),(-22.9424500656821,-22.9264810262011,-22.4280792647619,
-21.9296775033228,-21.4312757418836,-20.9328739804445,-20.4344722190053,
-19.9360704575661,-19.437668696127,-18.9392669346878,-18.4408651732487,
-17.9424634118095,-17.4440616503704,-16.9456598889312,-16.6592647585025),
 .UNSPECIFIED.);
#2842=B_SPLINE_CURVE_WITH_KNOTS('',3,(#66306,#66307,#66308,#66309,#66310,
#66311,#66312,#66313,#66314,#66315,#66316,#66317,#66318,#66319,#66320,#66321,
#66322,#66323,#66324,#66325,#66326,#66327,#66328,#66329,#66330,#66331,#66332,
#66333,#66334,#66335,#66336,#66337,#66338,#66339,#66340,#66341,#66342,#66343,
#66344,#66345,#66346,#66347,#66348),.UNSPECIFIED.,.F.,.F.,(4,3,3,3,3,3,
3,3,3,3,3,3,3,3,4),(13.686427997761,13.9552493202963,14.4536510817355,14.9520528431746,
15.4504546046138,15.9488563660529,16.4472581274921,16.9456598889312,17.4440616503704,
17.9424634118095,18.4408651732487,18.9392669346878,19.437668696127,19.9360704575661,
19.9696133049406),.UNSPECIFIED.);
#2843=B_SPLINE_CURVE_WITH_KNOTS('',3,(#66353,#66354,#66355,#66356,#66357,
#66358,#66359,#66360,#66361,#66362,#66363,#66364,#66365,#66366,#66367,#66368,
#66369,#66370,#66371,#66372,#66373,#66374,#66375,#66376,#66377,#66378,#66379,
#66380,#66381,#66382,#66383,#66384,#66385,#66386,#66387,#66388,#66389,#66390,
#66391,#66392),.UNSPECIFIED.,.F.,.F.,(4,3,3,3,3,3,3,3,3,3,3,3,3,4),(-29.2256353728617,
-28.9073021634709,-28.4089004020318,-27.9104986405926,-27.4120968791534,
-26.9136951177143,-26.4152933562751,-25.916891594836,-25.4184898333968,
-24.9200880719577,-24.4216863105185,-23.9232845490794,-23.4248827876402,
-22.9424500656821),.UNSPECIFIED.);
#2844=B_SPLINE_CURVE_WITH_KNOTS('',3,(#66393,#66394,#66395,#66396,#66397,
#66398,#66399,#66400,#66401,#66402,#66403,#66404,#66405,#66406,#66407,#66408,
#66409,#66410,#66411,#66412,#66413,#66414,#66415,#66416,#66417,#66418,#66419,
#66420,#66421,#66422,#66423,#66424,#66425,#66426,#66427,#66428,#66429,#66430,
#66431,#66432),.UNSPECIFIED.,.F.,.F.,(4,3,3,3,3,3,3,3,3,3,3,3,3,4),(19.9696133049406,
20.4344722190053,20.9328739804445,21.4312757418836,21.9296775033228,22.4280792647619,
22.9264810262011,23.4248827876402,23.9232845490794,24.4216863105185,24.9200880719577,
25.4184898333968,25.916891594836,26.2527986121202),.UNSPECIFIED.);
#2845=B_SPLINE_CURVE_WITH_KNOTS('',3,(#66437,#66438,#66439,#66440,#66441,
#66442,#66443,#66444,#66445,#66446,#66447,#66448,#66449,#66450,#66451,#66452,
#66453,#66454,#66455,#66456,#66457,#66458,#66459,#66460,#66461,#66462,#66463,
#66464,#66465,#66466,#66467,#66468,#66469,#66470,#66471,#66472,#66473,#66474,
#66475,#66476,#66477,#66478,#66479),.UNSPECIFIED.,.F.,.F.,(4,3,3,3,3,3,
3,3,3,3,3,3,3,3,4),(-35.5088206800413,-35.3865250621799,-34.8881233007408,
-34.3897215393016,-33.8913197778624,-33.3929180164233,-32.8945162549841,
-32.396114493545,-31.8977127321058,-31.3993109706667,-30.9009092092275,
-30.4025074477884,-29.9041056863492,-29.4057039249101,-29.2256353728617),
 .UNSPECIFIED.);
#2846=B_SPLINE_CURVE_WITH_KNOTS('',3,(#66480,#66481,#66482,#66483,#66484,
#66485,#66486,#66487,#66488,#66489,#66490,#66491,#66492,#66493,#66494,#66495,
#66496,#66497,#66498,#66499,#66500,#66501,#66502,#66503,#66504,#66505,#66506,
#66507,#66508,#66509,#66510,#66511,#66512,#66513,#66514,#66515,#66516,#66517,
#66518,#66519,#66520,#66521,#66522),.UNSPECIFIED.,.F.,.F.,(4,3,3,3,3,3,
3,3,3,3,3,3,3,3,4),(26.2527986121202,26.4152933562751,26.9136951177143,
27.4120968791534,27.9104986405926,28.4089004020318,28.9073021634709,29.4057039249101,
29.9041056863492,30.4025074477884,30.9009092092275,31.3993109706667,31.8977127321058,
32.396114493545,32.5359839192998),.UNSPECIFIED.);
#2847=B_SPLINE_CURVE_WITH_KNOTS('',3,(#66527,#66528,#66529,#66530,#66531,
#66532,#66533,#66534,#66535,#66536,#66537,#66538,#66539,#66540,#66541,#66542,
#66543,#66544,#66545,#66546,#66547,#66548,#66549,#66550,#66551,#66552,#66553,
#66554,#66555,#66556,#66557,#66558,#66559,#66560,#66561,#66562,#66563,#66564,
#66565,#66566),.UNSPECIFIED.,.F.,.F.,(4,3,3,3,3,3,3,3,3,3,3,3,3,4),(-41.7920059872209,
-41.3673461994497,-40.8689444380106,-40.3705426765714,-39.8721409151323,
-39.3737391536931,-38.875337392254,-38.3769356308148,-37.8785338693757,
-37.3801321079365,-36.8817303464974,-36.3833285850582,-35.8849268236191,
-35.5088206800413),.UNSPECIFIED.);
#2848=B_SPLINE_CURVE_WITH_KNOTS('',3,(#66567,#66568,#66569,#66570,#66571,
#66572,#66573,#66574,#66575,#66576,#66577,#66578,#66579,#66580,#66581,#66582,
#66583,#66584,#66585,#66586,#66587,#66588,#66589,#66590,#66591,#66592,#66593,
#66594,#66595,#66596,#66597,#66598,#66599,#66600,#66601,#66602,#66603,#66604,
#66605,#66606),.UNSPECIFIED.,.F.,.F.,(4,3,3,3,3,3,3,3,3,3,3,3,3,4),(32.5359839192998,
32.8945162549841,33.3929180164233,33.8913197778625,34.3897215393016,34.8881233007408,
35.3865250621799,35.8849268236191,36.3833285850582,36.8817303464974,37.3801321079365,
37.8785338693757,38.3769356308148,38.8191692264794),.UNSPECIFIED.);
#2849=B_SPLINE_CURVE_WITH_KNOTS('',3,(#66611,#66612,#66613,#66614,#66615,
#66616,#66617,#66618,#66619,#66620,#66621,#66622,#66623,#66624,#66625,#66626,
#66627,#66628,#66629,#66630,#66631,#66632,#66633,#66634,#66635,#66636,#66637,
#66638,#66639,#66640,#66641,#66642,#66643,#66644,#66645,#66646,#66647,#66648,
#66649,#66650,#66651,#66652,#66653),.UNSPECIFIED.,.F.,.F.,(4,3,3,3,3,3,
3,3,3,3,3,3,3,3,4),(-48.0751912944005,-47.8465690981587,-47.3481673367196,
-46.8497655752804,-46.3513638138413,-45.8529620524021,-45.354560290963,
-44.8561585295238,-44.3577567680847,-43.8593550066455,-43.3609532452064,
-42.8625514837672,-42.3641497223281,-41.8657479608889,-41.7920059872209),
 .UNSPECIFIED.);
#2850=B_SPLINE_CURVE_WITH_KNOTS('',3,(#66654,#66655,#66656,#66657,#66658,
#66659,#66660,#66661,#66662,#66663,#66664,#66665,#66666,#66667,#66668,#66669,
#66670,#66671,#66672,#66673,#66674,#66675,#66676,#66677,#66678,#66679,#66680,
#66681,#66682,#66683,#66684,#66685,#66686,#66687,#66688,#66689,#66690,#66691,
#66692,#66693,#66694,#66695,#66696),.UNSPECIFIED.,.F.,.F.,(4,3,3,3,3,3,
3,3,3,3,3,3,3,3,4),(38.8191692264794,38.875337392254,39.3737391536931,39.8721409151323,
40.3705426765714,40.8689444380106,41.3673461994498,41.8657479608889,42.3641497223281,
42.8625514837672,43.3609532452064,43.8593550066455,44.3577567680847,44.8561585295238,
45.102354533659),.UNSPECIFIED.);
#2851=B_SPLINE_CURVE_WITH_KNOTS('',3,(#66701,#66702,#66703,#66704,#66705,
#66706,#66707,#66708,#66709,#66710,#66711,#66712,#66713,#66714,#66715,#66716,
#66717,#66718,#66719,#66720,#66721,#66722,#66723,#66724,#66725,#66726,#66727,
#66728,#66729,#66730,#66731,#66732,#66733,#66734,#66735,#66736,#66737,#66738,
#66739,#66740,#66741,#66742,#66743),.UNSPECIFIED.,.F.,.F.,(4,3,3,3,3,3,
3,3,3,3,3,3,3,3,4),(-54.3583766015801,-54.3257919968678,-53.8273902354286,
-53.3289884739894,-52.8305867125503,-52.3321849511111,-51.833783189672,
-51.3353814282328,-50.8369796667937,-50.3385779053545,-49.8401761439154,
-49.3417743824762,-48.8433726210371,-48.3449708595979,-48.0751912944005),
 .UNSPECIFIED.);
#2852=B_SPLINE_CURVE_WITH_KNOTS('',3,(#66744,#66745,#66746,#66747,#66748,
#66749,#66750,#66751,#66752,#66753,#66754,#66755,#66756,#66757,#66758,#66759,
#66760,#66761,#66762,#66763,#66764,#66765,#66766,#66767,#66768,#66769,#66770,
#66771,#66772,#66773,#66774,#66775,#66776,#66777,#66778,#66779,#66780,#66781,
#66782,#66783,#66784,#66785,#66786),.UNSPECIFIED.,.F.,.F.,(4,3,3,3,3,3,
3,3,3,3,3,3,3,3,4),(45.102354533659,45.354560290963,45.8529620524021,46.3513638138413,
46.8497655752804,47.3481673367196,47.8465690981588,48.3449708595979,48.8433726210371,
49.3417743824762,49.8401761439154,50.3385779053545,50.8369796667937,51.3353814282328,
51.3855398408386),.UNSPECIFIED.);
#2853=B_SPLINE_CURVE_WITH_KNOTS('',3,(#66791,#66792,#66793,#66794,#66795,
#66796,#66797,#66798,#66799,#66800,#66801,#66802,#66803,#66804,#66805,#66806,
#66807,#66808,#66809,#66810,#66811,#66812,#66813,#66814,#66815,#66816,#66817,
#66818,#66819,#66820,#66821,#66822,#66823,#66824,#66825,#66826,#66827,#66828,
#66829,#66830),.UNSPECIFIED.,.F.,.F.,(4,3,3,3,3,3,3,3,3,3,3,3,3,4),(-60.6415619087597,
-60.3066131341376,-59.8082113726984,-59.3098096112593,-58.8114078498201,
-58.313006088381,-57.8146043269418,-57.3162025655027,-56.8178008040635,
-56.3193990426244,-55.8209972811852,-55.3225955197461,-54.8241937583069,
-54.3583766015801),.UNSPECIFIED.);
#2854=B_SPLINE_CURVE_WITH_KNOTS('',3,(#66831,#66832,#66833,#66834,#66835,
#66836,#66837,#66838,#66839,#66840,#66841,#66842,#66843,#66844,#66845,#66846,
#66847,#66848,#66849,#66850,#66851,#66852,#66853,#66854,#66855,#66856,#66857,
#66858,#66859,#66860,#66861,#66862,#66863,#66864,#66865,#66866,#66867,#66868,
#66869,#66870),.UNSPECIFIED.,.F.,.F.,(4,3,3,3,3,3,3,3,3,3,3,3,3,4),(51.3855398408386,
51.833783189672,52.3321849511111,52.8305867125503,53.3289884739894,53.8273902354286,
54.3257919968677,54.8241937583069,55.3225955197461,55.8209972811852,56.3193990426244,
56.8178008040635,57.3162025655027,57.6687251480181),.UNSPECIFIED.);
#2855=B_SPLINE_CURVE_WITH_KNOTS('',3,(#66875,#66876,#66877,#66878,#66879,
#66880,#66881,#66882,#66883,#66884,#66885,#66886,#66887,#66888,#66889,#66890,
#66891,#66892,#66893,#66894,#66895,#66896,#66897,#66898,#66899,#66900,#66901,
#66902,#66903,#66904,#66905,#66906,#66907,#66908,#66909,#66910,#66911,#66912,
#66913,#66914,#66915,#66916,#66917),.UNSPECIFIED.,.F.,.F.,(4,3,3,3,3,3,
3,3,3,3,3,3,3,3,4),(-66.9247472159393,-66.7858360328466,-66.2874342714074,
-65.7890325099683,-65.2906307485291,-64.79222898709,-64.2938272256508,-63.7954254642117,
-63.2970237027725,-62.7986219413334,-62.3002201798942,-61.8018184184551,
-61.3034166570159,-60.8050148955767,-60.6415619087597),.UNSPECIFIED.);
#2856=B_SPLINE_CURVE_WITH_KNOTS('',3,(#66918,#66919,#66920,#66921,#66922,
#66923,#66924,#66925,#66926,#66927,#66928,#66929,#66930,#66931,#66932,#66933,
#66934,#66935,#66936,#66937,#66938,#66939,#66940,#66941,#66942,#66943,#66944,
#66945,#66946,#66947,#66948,#66949,#66950,#66951,#66952,#66953,#66954,#66955,
#66956,#66957,#66958,#66959,#66960),.UNSPECIFIED.,.F.,.F.,(4,3,3,3,3,3,
3,3,3,3,3,3,3,3,4),(57.6687251480181,57.8146043269418,58.313006088381,58.8114078498201,
59.3098096112593,59.8082113726984,60.3066131341376,60.8050148955767,61.3034166570159,
61.801818418455,62.3002201798942,62.7986219413334,63.2970237027725,63.7954254642117,
63.9519104551977),.UNSPECIFIED.);
#2857=B_SPLINE_CURVE_WITH_KNOTS('',3,(#66965,#66966,#66967,#66968,#66969,
#66970,#66971,#66972,#66973,#66974,#66975,#66976,#66977,#66978,#66979,#66980,
#66981,#66982,#66983,#66984,#66985,#66986,#66987,#66988,#66989,#66990,#66991,
#66992,#66993,#66994,#66995,#66996,#66997,#66998,#66999,#67000,#67001,#67002,
#67003,#67004),.UNSPECIFIED.,.F.,.F.,(4,3,3,3,3,3,3,3,3,3,3,3,3,4),(-73.2079325231189,
-72.7666571701164,-72.2682554086773,-71.7698536472381,-71.271451885799,
-70.7730501243598,-70.2746483629207,-69.7762466014815,-69.2778448400424,
-68.7794430786032,-68.2810413171641,-67.7826395557249,-67.2842377942858,
-66.9247472159393),.UNSPECIFIED.);
#2858=B_SPLINE_CURVE_WITH_KNOTS('',3,(#67005,#67006,#67007,#67008,#67009,
#67010,#67011,#67012,#67013,#67014,#67015,#67016,#67017,#67018,#67019,#67020,
#67021,#67022,#67023,#67024,#67025,#67026,#67027,#67028,#67029,#67030,#67031,
#67032,#67033,#67034,#67035,#67036,#67037,#67038,#67039,#67040,#67041,#67042,
#67043,#67044),.UNSPECIFIED.,.F.,.F.,(4,3,3,3,3,3,3,3,3,3,3,3,3,4),(63.9519104551977,
64.2938272256508,64.79222898709,65.2906307485291,65.7890325099683,66.2874342714074,
66.7858360328466,67.2842377942857,67.7826395557249,68.2810413171641,68.7794430786032,
69.2778448400424,69.7762466014815,70.2350957623773),.UNSPECIFIED.);
#2859=B_SPLINE_CURVE_WITH_KNOTS('',3,(#67049,#67050,#67051,#67052,#67053,
#67054,#67055,#67056,#67057,#67058,#67059,#67060,#67061,#67062,#67063,#67064,
#67065,#67066,#67067,#67068,#67069,#67070,#67071,#67072,#67073,#67074,#67075,
#67076,#67077,#67078,#67079,#67080,#67081,#67082,#67083,#67084,#67085,#67086,
#67087,#67088,#67089,#67090,#67091),.UNSPECIFIED.,.F.,.F.,(4,3,3,3,3,3,
3,3,3,3,3,3,3,3,4),(-79.4911178302985,-79.2458800688254,-78.7474783073863,
-78.2490765459471,-77.750674784508,-77.2522730230688,-76.7538712616297,
-76.2554695001905,-75.7570677387514,-75.2586659773122,-74.760264215873,
-74.2618624544339,-73.7634606929947,-73.2650589315556,-73.2079325231189),
 .UNSPECIFIED.);
#2860=B_SPLINE_CURVE_WITH_KNOTS('',3,(#67092,#67093,#67094,#67095,#67096,
#67097,#67098,#67099,#67100,#67101,#67102,#67103,#67104,#67105,#67106,#67107,
#67108,#67109,#67110,#67111,#67112,#67113,#67114,#67115,#67116,#67117,#67118,
#67119,#67120,#67121,#67122,#67123,#67124,#67125,#67126,#67127,#67128,#67129,
#67130,#67131,#67132,#67133,#67134),.UNSPECIFIED.,.F.,.F.,(4,3,3,3,3,3,
3,3,3,3,3,3,3,3,4),(70.2350957623773,70.2746483629207,70.7730501243598,
71.271451885799,71.7698536472381,72.2682554086773,72.7666571701164,73.2650589315556,
73.7634606929947,74.2618624544339,74.760264215873,75.2586659773122,75.7570677387513,
76.2554695001905,76.5182810695569),.UNSPECIFIED.);
#2861=B_SPLINE_CURVE_WITH_KNOTS('',3,(#67139,#67140,#67141,#67142,#67143,
#67144,#67145,#67146,#67147,#67148,#67149,#67150,#67151,#67152,#67153,#67154,
#67155,#67156,#67157,#67158,#67159,#67160,#67161,#67162,#67163,#67164,#67165,
#67166,#67167,#67168,#67169,#67170,#67171,#67172,#67173,#67174,#67175,#67176,
#67177,#67178,#67179,#67180,#67181),.UNSPECIFIED.,.F.,.F.,(4,3,3,3,3,3,
3,3,3,3,3,3,3,3,4),(-85.774303137478,-85.7251029675344,-85.2267012060953,
-84.7282994446561,-84.229897683217,-83.7314959217778,-83.2330941603387,
-82.7346923988995,-82.2362906374604,-81.7378888760212,-81.239487114582,
-80.7410853531429,-80.2426835917038,-79.7442818302646,-79.4911178302985),
 .UNSPECIFIED.);
#2862=B_SPLINE_CURVE_WITH_KNOTS('',3,(#67182,#67183,#67184,#67185,#67186,
#67187,#67188,#67189,#67190,#67191,#67192,#67193,#67194,#67195,#67196,#67197,
#67198,#67199,#67200,#67201,#67202,#67203,#67204,#67205,#67206,#67207,#67208,
#67209,#67210,#67211,#67212,#67213,#67214,#67215,#67216,#67217,#67218,#67219,
#67220,#67221,#67222,#67223,#67224),.UNSPECIFIED.,.F.,.F.,(4,3,3,3,3,3,
3,3,3,3,3,3,3,3,4),(76.5182810695569,76.7538712616297,77.2522730230688,
77.750674784508,78.2490765459471,78.7474783073863,79.2458800688254,79.7442818302646,
80.2426835917037,80.7410853531429,81.239487114582,81.7378888760212,82.2362906374604,
82.7346923988995,82.8014663767365),.UNSPECIFIED.);
#2863=B_SPLINE_CURVE_WITH_KNOTS('',3,(#67229,#67230,#67231,#67232,#67233,
#67234,#67235,#67236,#67237,#67238,#67239,#67240,#67241,#67242,#67243,#67244,
#67245,#67246,#67247,#67248,#67249,#67250,#67251,#67252,#67253,#67254,#67255,
#67256,#67257,#67258,#67259,#67260,#67261,#67262,#67263,#67264,#67265,#67266,
#67267,#67268),.UNSPECIFIED.,.F.,.F.,(4,3,3,3,3,3,3,3,3,3,3,3,3,4),(-92.0574884446577,
-91.7059241048043,-91.2075223433651,-90.709120581926,-90.2107188204868,
-89.7123170590477,-89.2139152976085,-88.7155135361694,-88.2171117747302,
-87.718710013291,-87.2203082518519,-86.7219064904127,-86.2235047289736,
-85.774303137478),.UNSPECIFIED.);
#2864=B_SPLINE_CURVE_WITH_KNOTS('',3,(#67269,#67270,#67271,#67272,#67273,
#67274,#67275,#67276,#67277,#67278,#67279,#67280,#67281,#67282,#67283,#67284,
#67285,#67286,#67287,#67288,#67289,#67290,#67291,#67292,#67293,#67294,#67295,
#67296,#67297,#67298,#67299,#67300,#67301,#67302,#67303,#67304,#67305,#67306,
#67307,#67308),.UNSPECIFIED.,.F.,.F.,(4,3,3,3,3,3,3,3,3,3,3,3,3,4),(82.8014663767365,
83.2330941603387,83.7314959217778,84.229897683217,84.7282994446561,85.2267012060953,
85.7251029675344,86.2235047289736,86.7219064904127,87.2203082518519,87.718710013291,
88.2171117747302,88.7155135361694,89.0846516839161),.UNSPECIFIED.);
#2865=B_SPLINE_CURVE_WITH_KNOTS('',3,(#67313,#67314,#67315,#67316,#67317,
#67318,#67319,#67320,#67321,#67322,#67323,#67324,#67325,#67326,#67327,#67328,
#67329,#67330,#67331,#67332,#67333,#67334,#67335,#67336,#67337,#67338,#67339,
#67340,#67341,#67342,#67343,#67344,#67345,#67346,#67347,#67348,#67349,#67350,
#67351,#67352,#67353,#67354,#67355),.UNSPECIFIED.,.F.,.F.,(4,3,3,3,3,3,
3,3,3,3,3,3,3,3,4),(-98.3406737518372,-98.1851470035133,-97.6867452420741,
-97.188343480635,-96.6899417191958,-96.1915399577567,-95.6931381963175,
-95.1947364348784,-94.6963346734392,-94.197932912,-93.6995311505609,-93.2011293891217,
-92.7027276276826,-92.2043258662434,-92.0574884446577),.UNSPECIFIED.);
#2866=B_SPLINE_CURVE_WITH_KNOTS('',3,(#67356,#67357,#67358,#67359,#67360,
#67361,#67362,#67363,#67364,#67365,#67366,#67367,#67368,#67369,#67370,#67371,
#67372,#67373,#67374,#67375,#67376,#67377,#67378,#67379,#67380,#67381,#67382,
#67383,#67384,#67385,#67386,#67387,#67388,#67389,#67390,#67391,#67392,#67393,
#67394,#67395,#67396,#67397,#67398),.UNSPECIFIED.,.F.,.F.,(4,3,3,3,3,3,
3,3,3,3,3,3,3,3,4),(89.0846516839161,89.2139152976085,89.7123170590477,
90.2107188204868,90.709120581926,91.2075223433651,91.7059241048043,92.2043258662434,
92.7027276276826,93.2011293891217,93.6995311505609,94.197932912,94.6963346734392,
95.1947364348784,95.3678369910957),.UNSPECIFIED.);
#2867=B_SPLINE_CURVE_WITH_KNOTS('',3,(#67404,#67405,#67406,#67407),
 .UNSPECIFIED.,.F.,.F.,(4,4),(109.955742875643,110.220866060559),
 .UNSPECIFIED.);
#2868=B_SPLINE_CURVE_WITH_KNOTS('',3,(#67413,#67414,#67415,#67416,#67417,
#67418,#67419,#67420,#67421,#67422,#67423,#67424,#67425,#67426,#67427,#67428,
#67429),.UNSPECIFIED.,.F.,.F.,(4,1,1,1,1,1,1,1,1,1,1,1,1,1,4),(103.672557568463,
103.819394990049,104.317796751488,104.816198512927,105.314600274366,105.813002035806,
106.311403797245,106.809805558684,107.308207320123,107.806609081562,108.305010843001,
108.80341260444,109.30181436588,109.800216127319,109.955742875643),
 .UNSPECIFIED.);
#2869=B_SPLINE_CURVE_WITH_KNOTS('',3,(#67432,#67433,#67434,#67435,#67436,
#67437,#67438,#67439,#67440,#67441,#67442,#67443,#67444,#67445),
 .UNSPECIFIED.,.F.,.F.,(4,1,1,1,1,1,1,1,1,1,1,4),(103.672557568463,103.997858773685,
104.496260535124,104.994662296563,105.493064058002,105.991465819441,106.489867580881,
106.98826934232,107.486671103759,107.985072865198,108.483474626637,108.981876388076),
 .UNSPECIFIED.);
#2870=B_SPLINE_CURVE_WITH_KNOTS('',3,(#67450,#67451,#67452,#67453,#67454,
#67455,#67456,#67457,#67458,#67459,#67460,#67461,#67462,#67463,#67464,#67465),
 .UNSPECIFIED.,.F.,.F.,(4,1,1,1,1,1,1,1,1,1,1,1,1,4),(97.3893722612836,
97.8385738527791,98.3369756142182,98.8353773756574,99.3337791370966,99.8321808985357,
100.330582659975,100.828984421414,101.327386182853,101.825787944292,102.324189705731,
102.822591467171,103.32099322861,103.672557568463),.UNSPECIFIED.);
#2871=B_SPLINE_CURVE_WITH_KNOTS('',3,(#67466,#67467,#67468,#67469,#67470,
#67471,#67472,#67473,#67474,#67475,#67476,#67477,#67478,#67479,#67480,#67481,
#67482),.UNSPECIFIED.,.F.,.F.,(4,1,1,1,1,1,1,1,1,1,1,1,1,1,4),(97.3893722612836,
97.5186358749759,98.017037636415,98.5154393978542,99.0138411592933,99.5122429207325,
100.010644682172,100.509046443611,101.00744820505,101.505849966489,102.004251727928,
102.502653489367,103.001055250807,103.499457012246,103.672557568463),
 .UNSPECIFIED.);
#2872=B_SPLINE_CURVE_WITH_KNOTS('',3,(#67487,#67488,#67489,#67490,#67491,
#67492,#67493,#67494,#67495,#67496,#67497,#67498,#67499,#67500,#67501,#67502,
#67503),.UNSPECIFIED.,.F.,.F.,(4,1,1,1,1,1,1,1,1,1,1,1,1,1,4),(91.106186954104,
91.3593509540701,91.8577527155093,92.3561544769484,92.8545562383876,93.3529579998267,
93.8513597612659,94.349761522705,94.8481632841442,95.3465650455833,95.8449668070225,
96.3433685684616,96.8417703299008,97.34017209134,97.3893722612836),
 .UNSPECIFIED.);
#2873=B_SPLINE_CURVE_WITH_KNOTS('',3,(#67504,#67505,#67506,#67507,#67508,
#67509,#67510,#67511,#67512,#67513,#67514,#67515,#67516,#67517,#67518,#67519),
 .UNSPECIFIED.,.F.,.F.,(4,1,1,1,1,1,1,1,1,1,1,1,1,4),(91.106186954104,91.537814737706,
92.0362164991452,92.5346182605844,93.0330200220235,93.5314217834626,94.0298235449018,
94.528225306341,95.0266270677801,95.5250288292193,96.0234305906584,96.5218323520976,
97.0202341135367,97.3893722612836),.UNSPECIFIED.);
#2874=B_SPLINE_CURVE_WITH_KNOTS('',3,(#67524,#67525,#67526,#67527,#67528,
#67529,#67530,#67531,#67532,#67533,#67534,#67535,#67536,#67537,#67538,#67539,
#67540),.UNSPECIFIED.,.F.,.F.,(4,1,1,1,1,1,1,1,1,1,1,1,1,1,4),(84.8230016469244,
84.8801280553611,85.3785298168003,85.8769315782394,86.3753333396786,86.8737351011177,
87.3721368625569,87.870538623996,88.3689403854352,88.8673421468743,89.3657439083135,
89.8641456697526,90.3625474311918,90.860949192631,91.106186954104),
 .UNSPECIFIED.);
#2875=B_SPLINE_CURVE_WITH_KNOTS('',3,(#67541,#67542,#67543,#67544,#67545,
#67546,#67547,#67548,#67549,#67550,#67551,#67552,#67553,#67554,#67555,#67556,
#67557),.UNSPECIFIED.,.F.,.F.,(4,1,1,1,1,1,1,1,1,1,1,1,1,1,4),(84.8230016469244,
85.058591838997,85.5569936004362,86.0553953618753,86.5537971233145,87.0521988847537,
87.5506006461928,88.049002407632,88.5474041690711,89.0458059305103,89.5442076919494,
90.0426094533886,90.5410112148277,91.0394129762669,91.106186954104),
 .UNSPECIFIED.);
#2876=B_SPLINE_CURVE_WITH_KNOTS('',3,(#67562,#67563,#67564,#67565,#67566,
#67567,#67568,#67569,#67570,#67571,#67572,#67573,#67574,#67575,#67576,#67577),
 .UNSPECIFIED.,.F.,.F.,(4,1,1,1,1,1,1,1,1,1,1,1,1,4),(78.5398163397448,
78.8993069180913,79.3977086795304,79.8961104409696,80.3945122024087,80.8929139638479,
81.391315725287,81.8897174867262,82.3881192481653,82.8865210096045,83.3849227710436,
83.8833245324828,84.381726293922,84.8230016469244),.UNSPECIFIED.);
#2877=B_SPLINE_CURVE_WITH_KNOTS('',3,(#67578,#67579,#67580,#67581,#67582,
#67583,#67584,#67585,#67586,#67587,#67588,#67589,#67590,#67591,#67592,#67593,
#67594),.UNSPECIFIED.,.F.,.F.,(4,1,1,1,1,1,1,1,1,1,1,1,1,1,4),(78.5398163397448,
78.579368940288,79.0777707017272,79.5761724631663,80.0745742246055,80.5729759860447,
81.0713777474838,81.569779508923,82.0681812703621,82.5665830318013,83.0649847932404,
83.5633865546796,84.0617883161187,84.5601900775579,84.8230016469244),
 .UNSPECIFIED.);
#2878=B_SPLINE_CURVE_WITH_KNOTS('',3,(#67599,#67600,#67601,#67602,#67603,
#67604,#67605,#67606,#67607,#67608,#67609,#67610,#67611,#67612,#67613,#67614,
#67615),.UNSPECIFIED.,.F.,.F.,(4,1,1,1,1,1,1,1,1,1,1,1,1,1,4),(72.2566310325652,
72.4200840193823,72.9184857808214,73.4168875422606,73.9152893036997,74.4136910651389,
74.912092826578,75.4104945880172,75.9088963494563,76.4072981108955,76.9056998723347,
77.4041016337738,77.902503395213,78.4009051566521,78.5398163397448),
 .UNSPECIFIED.);
#2879=B_SPLINE_CURVE_WITH_KNOTS('',3,(#67616,#67617,#67618,#67619,#67620,
#67621,#67622,#67623,#67624,#67625,#67626,#67627,#67628,#67629,#67630,#67631),
 .UNSPECIFIED.,.F.,.F.,(4,1,1,1,1,1,1,1,1,1,1,1,1,4),(72.2566310325652,
72.5985478030182,73.0969495644573,73.5953513258965,74.0937530873357,74.5921548487748,
75.090556610214,75.5889583716531,76.0873601330923,76.5857618945314,77.0841636559706,
77.5825654174097,78.0809671788489,78.5398163397448),.UNSPECIFIED.);
#2880=B_SPLINE_CURVE_WITH_KNOTS('',3,(#67636,#67637,#67638,#67639,#67640,
#67641,#67642,#67643,#67644,#67645,#67646,#67647,#67648,#67649,#67650,#67651),
 .UNSPECIFIED.,.F.,.F.,(4,1,1,1,1,1,1,1,1,1,1,1,1,4),(65.9734457253856,
66.4392628821124,66.9376646435516,67.4360664049907,67.9344681664299,68.432869927869,
68.9312716893082,69.4296734507473,69.9280752121865,70.4264769736257,70.9248787350648,
71.4232804965039,71.9216822579431,72.2566310325652),.UNSPECIFIED.);
#2881=B_SPLINE_CURVE_WITH_KNOTS('',3,(#67652,#67653,#67654,#67655,#67656,
#67657,#67658,#67659,#67660,#67661,#67662,#67663,#67664,#67665,#67666,#67667,
#67668),.UNSPECIFIED.,.F.,.F.,(4,1,1,1,1,1,1,1,1,1,1,1,1,1,4),(65.9734457253856,
66.1193249043092,66.6177266657484,67.1161284271875,67.6145301886267,68.1129319500658,
68.611333711505,69.1097354729441,69.6081372343833,70.1065389958224,70.6049407572616,
71.1033425187007,71.6017442801399,72.1001460415791,72.2566310325652),
 .UNSPECIFIED.);
#2882=B_SPLINE_CURVE_WITH_KNOTS('',3,(#67673,#67674,#67675,#67676,#67677,
#67678,#67679,#67680,#67681,#67682,#67683,#67684,#67685,#67686,#67687,#67688,
#67689),.UNSPECIFIED.,.F.,.F.,(4,1,1,1,1,1,1,1,1,1,1,1,1,1,4),(59.690260418206,
59.9600399834034,60.4584417448426,60.9568435062817,61.4552452677209,61.95364702916,
62.4520487905992,62.9504505520383,63.4488523134775,63.9472540749166,64.4456558363558,
64.944057597795,65.4424593592341,65.9408611206733,65.9734457253856),
 .UNSPECIFIED.);
#2883=B_SPLINE_CURVE_WITH_KNOTS('',3,(#67690,#67691,#67692,#67693,#67694,
#67695,#67696,#67697,#67698,#67699,#67700,#67701,#67702,#67703,#67704,#67705),
 .UNSPECIFIED.,.F.,.F.,(4,1,1,1,1,1,1,1,1,1,1,1,1,4),(59.690260418206,60.1385037670394,
60.6369055284785,61.1353072899177,61.6337090513568,62.132110812796,62.6305125742351,
63.1289143356743,63.6273160971134,64.1257178585526,64.6241196199917,65.1225213814309,
65.6209231428701,65.9734457253856),.UNSPECIFIED.);
#2884=B_SPLINE_CURVE_WITH_KNOTS('',3,(#67710,#67711,#67712,#67713,#67714,
#67715,#67716,#67717,#67718,#67719,#67720,#67721,#67722,#67723,#67724,#67725,
#67726),.UNSPECIFIED.,.F.,.F.,(4,1,1,1,1,1,1,1,1,1,1,1,1,1,4),(53.4070751110264,
53.4808170846944,53.9792188461336,54.4776206075727,54.9760223690119,55.474424130451,
55.9728258918902,56.4712276533293,56.9696294147685,57.4680311762077,57.9664329376468,
58.464834699086,58.9632364605251,59.4616382219643,59.690260418206),
 .UNSPECIFIED.);
#2885=B_SPLINE_CURVE_WITH_KNOTS('',3,(#67727,#67728,#67729,#67730,#67731,
#67732,#67733,#67734,#67735,#67736,#67737,#67738,#67739,#67740,#67741,#67742,
#67743),.UNSPECIFIED.,.F.,.F.,(4,1,1,1,1,1,1,1,1,1,1,1,1,1,4),(53.4070751110264,
53.6592808683304,54.1576826297695,54.6560843912087,55.1544861526478,55.652887914087,
56.1512896755261,56.6496914369653,57.1480931984044,57.6464949598436,58.1448967212827,
58.6432984827219,59.1417002441611,59.6401020056002,59.690260418206),
 .UNSPECIFIED.);
#2886=B_SPLINE_CURVE_WITH_KNOTS('',3,(#67748,#67749,#67750,#67751,#67752,
#67753,#67754,#67755,#67756,#67757,#67758,#67759,#67760,#67761,#67762,#67763),
 .UNSPECIFIED.,.F.,.F.,(4,1,1,1,1,1,1,1,1,1,1,1,1,4),(47.1238898038469,
47.4999959474246,47.9983977088637,48.4967994703029,48.995201231742,49.4936029931812,
49.9920047546203,50.4904065160595,50.9888082774987,51.4872100389378,51.985611800377,
52.4840135618161,52.9824153232553,53.4070751110264),.UNSPECIFIED.);
#2887=B_SPLINE_CURVE_WITH_KNOTS('',3,(#67764,#67765,#67766,#67767,#67768,
#67769,#67770,#67771,#67772,#67773,#67774,#67775,#67776,#67777,#67778,#67779,
#67780),.UNSPECIFIED.,.F.,.F.,(4,1,1,1,1,1,1,1,1,1,1,1,1,1,4),(47.1238898038468,
47.1800579696214,47.6784597310605,48.1768614924997,48.6752632539388,49.173665015378,
49.6720667768171,50.1704685382563,50.6688702996954,51.1672720611346,51.6656738225738,
52.1640755840129,52.6624773454521,53.1608791068912,53.4070751110264),
 .UNSPECIFIED.);
#2888=B_SPLINE_CURVE_WITH_KNOTS('',3,(#67785,#67786,#67787,#67788,#67789,
#67790,#67791,#67792,#67793,#67794,#67795,#67796,#67797,#67798,#67799,#67800,
#67801),.UNSPECIFIED.,.F.,.F.,(4,1,1,1,1,1,1,1,1,1,1,1,1,1,4),(40.8407044966672,
41.0207730487156,41.5191748101547,42.0175765715939,42.515978333033,43.0143800944722,
43.5127818559113,44.0111836173505,44.5095853787897,45.0079871402288,45.506388901668,
46.0047906631071,46.5031924245463,47.0015941859854,47.1238898038469),
 .UNSPECIFIED.);
#2889=B_SPLINE_CURVE_WITH_KNOTS('',3,(#67802,#67803,#67804,#67805,#67806,
#67807,#67808,#67809,#67810,#67811,#67812,#67813,#67814,#67815,#67816,#67817),
 .UNSPECIFIED.,.F.,.F.,(4,1,1,1,1,1,1,1,1,1,1,1,1,4),(40.8407044966672,
41.1992368323515,41.6976385937907,42.1960403552298,42.694442116669,43.1928438781081,
43.6912456395473,44.1896474009864,44.6880491624256,45.1864509238648,45.6848526853039,
46.1832544467431,46.6816562081822,47.1238898038468),.UNSPECIFIED.);
#2890=B_SPLINE_CURVE_WITH_KNOTS('',3,(#67822,#67823,#67824,#67825,#67826,
#67827,#67828,#67829,#67830,#67831,#67832,#67833,#67834,#67835,#67836,#67837),
 .UNSPECIFIED.,.F.,.F.,(4,1,1,1,1,1,1,1,1,1,1,1,1,4),(34.5575191894876,
35.0399519114457,35.5383536728849,36.036755434324,36.5351571957632,37.0335589572024,
37.5319607186415,38.0303624800807,38.5287642415198,39.027166002959,39.5255677643981,
40.0239695258373,40.5223712872764,40.8407044966672),.UNSPECIFIED.);
#2891=B_SPLINE_CURVE_WITH_KNOTS('',3,(#67838,#67839,#67840,#67841,#67842,
#67843,#67844,#67845,#67846,#67847,#67848,#67849,#67850,#67851,#67852,#67853,
#67854),.UNSPECIFIED.,.F.,.F.,(4,1,1,1,1,1,1,1,1,1,1,1,1,1,4),(34.5575191894876,
34.7200139336425,35.2184156950817,35.7168174565208,36.21521921796,36.7136209793991,
37.2120227408383,37.7104245022774,38.2088262637166,38.7072280251558,39.2056297865949,
39.7040315480341,40.2024333094732,40.7008350709124,40.8407044966672),
 .UNSPECIFIED.);
#2892=B_SPLINE_CURVE_WITH_KNOTS('',3,(#67859,#67860,#67861,#67862,#67863,
#67864,#67865,#67866,#67867,#67868,#67869,#67870,#67871,#67872,#67873,#67874,
#67875),.UNSPECIFIED.,.F.,.F.,(4,1,1,1,1,1,1,1,1,1,1,1,1,1,4),(28.2743338823081,
28.5607290127367,29.0591307741759,29.5575325356151,30.0559342970542,30.5543360584934,
31.0527378199325,31.5511395813717,32.0495413428108,32.54794310425,33.0463448656891,
33.5447466271283,34.0431483885674,34.5415501500066,34.5575191894876),
 .UNSPECIFIED.);
#2893=B_SPLINE_CURVE_WITH_KNOTS('',3,(#67876,#67877,#67878,#67879,#67880,
#67881,#67882,#67883,#67884,#67885,#67886,#67887,#67888,#67889,#67890,#67891),
 .UNSPECIFIED.,.F.,.F.,(4,1,1,1,1,1,1,1,1,1,1,1,1,4),(28.2743338823081,
28.7391927963727,29.2375945578118,29.735996319251,30.2343980806901,30.7327998421293,
31.2312016035684,31.7296033650076,32.2280051264468,32.7264068878859,33.2248086493251,
33.7232104107642,34.2216121722034,34.5575191894876),.UNSPECIFIED.);
#2894=B_SPLINE_CURVE_WITH_KNOTS('',3,(#67896,#67897,#67898,#67899,#67900,
#67901,#67902,#67903,#67904,#67905,#67906,#67907,#67908,#67909,#67910,#67911,
#67912),.UNSPECIFIED.,.F.,.F.,(4,1,1,1,1,1,1,1,1,1,1,1,1,1,4),(21.9911485751285,
22.0815061140277,22.5799078754669,23.0783096369061,23.5767113983452,24.0751131597844,
24.5735149212235,25.0719166826627,25.5703184441018,26.068720205541,26.5671219669801,
27.0655237284193,27.5639254898584,28.0623272512976,28.2743338823081),
 .UNSPECIFIED.);
#2895=B_SPLINE_CURVE_WITH_KNOTS('',3,(#67913,#67914,#67915,#67916,#67917,
#67918,#67919,#67920,#67921,#67922,#67923,#67924,#67925,#67926,#67927,#67928,
#67929),.UNSPECIFIED.,.F.,.F.,(4,1,1,1,1,1,1,1,1,1,1,1,1,1,4),(21.9911485751285,
22.2599698976637,22.7583716591028,23.256773420542,23.7551751819811,24.2535769434203,
24.7519787048595,25.2503804662986,25.7487822277378,26.2471839891769,26.7455857506161,
27.2439875120552,27.7423892734944,28.2407910349335,28.2743338823081),
 .UNSPECIFIED.);
#2896=B_SPLINE_CURVE_WITH_KNOTS('',3,(#67934,#67935,#67936,#67937,#67938,
#67939,#67940,#67941,#67942,#67943,#67944,#67945,#67946,#67947,#67948,#67949),
 .UNSPECIFIED.,.F.,.F.,(4,1,1,1,1,1,1,1,1,1,1,1,1,4),(15.7079632679489,
16.1006849767579,16.5990867381971,17.0974884996362,17.5958902610754,18.0942920225145,
18.5926937839537,19.0910955453928,19.589497306832,20.0878990682711,20.5863008297103,
21.0847025911494,21.5831043525886,21.9911485751285),.UNSPECIFIED.);
#2897=B_SPLINE_CURVE_WITH_KNOTS('',3,(#67950,#67951,#67952,#67953,#67954,
#67955,#67956,#67957,#67958,#67959,#67960,#67961,#67962,#67963,#67964,#67965,
#67966),.UNSPECIFIED.,.F.,.F.,(4,1,1,1,1,1,1,1,1,1,1,1,1,1,4),(15.7079632679489,
15.7807469989547,16.2791487603938,16.777550521833,17.2759522832721,17.7743540447113,
18.2727558061505,18.7711575675896,19.2695593290288,19.7679610904679,20.2663628519071,
20.7647646133462,21.2631663747854,21.7615681362245,21.9911485751285),
 .UNSPECIFIED.);
#2898=B_SPLINE_CURVE_WITH_KNOTS('',3,(#67983,#67984,#67985,#67986,#67987,
#67988),.UNSPECIFIED.,.F.,.F.,(4,2,4),(0.164470082438344,0.176405072826056,
0.235193913087612),.UNSPECIFIED.);
#2899=B_SPLINE_CURVE_WITH_KNOTS('',3,(#67990,#67991,#67992,#67993,#67994,
#67995),.UNSPECIFIED.,.F.,.F.,(4,2,4),(0.235193913087612,0.293982753349168,
0.30591774373688),.UNSPECIFIED.);
#2900=B_SPLINE_CURVE_WITH_KNOTS('',3,(#67999,#68000,#68001,#68002,#68003,
#68004,#68005,#68006,#68007,#68008),.UNSPECIFIED.,.F.,.F.,(4,2,2,2,4),(0.634857908613568,
0.64679289900128,0.705581739262836,0.764370579524392,0.776305569912104),
 .UNSPECIFIED.);
#2901=B_SPLINE_CURVE_WITH_KNOTS('',3,(#68132,#68133,#68134,#68135,#68136,
#68137,#68138,#68139,#68140,#68141,#68142,#68143,#68144,#68145,#68146,#68147,
#68148,#68149,#68150,#68151,#68152,#68153),.UNSPECIFIED.,.F.,.F.,(4,1,2,
1,1,1,2,2,2,1,1,1,1,1,1,4),(0.,0.0584568917522064,0.116913783504413,0.175370117903373,
0.233826452302333,0.263054619501813,0.350739121100252,0.409196012852459,
0.467652904604665,0.526109517680248,0.569951977486936,0.584566130755832,
0.672251050369206,0.686865203638102,0.69417228027255,0.701479356906998),
 .UNSPECIFIED.);
#2902=B_SPLINE_CURVE_WITH_KNOTS('',3,(#68154,#68155,#68156,#68157,#68158,
#68159,#68160,#68161),.UNSPECIFIED.,.F.,.F.,(4,1,1,1,1,4),(0.701479356906998,
0.774550123251477,0.818392583058164,0.847620889595956,0.876849196133747,
0.93530580920933),.UNSPECIFIED.);
#2903=B_SPLINE_CURVE_WITH_KNOTS('',3,(#68162,#68163,#68164,#68165,#68166,
#68167,#68168,#68169,#68170,#68171,#68172,#68173,#68174,#68175,#68176,#68177,
#68178,#68179,#68180,#68181,#68182,#68183,#68184,#68185,#68186,#68187,#68188),
 .UNSPECIFIED.,.T.,.F.,(4,1,1,1,1,1,1,1,1,1,1,1,2,2,2,1,1,1,2,1,4),(-0.93530580920933,
-0.876849196133747,-0.847620889595956,-0.818392583058164,-0.774550123251477,
-0.701479356906998,-0.69417228027255,-0.686865203638102,-0.672251050369206,
-0.584566130755832,-0.569951977486936,-0.526109517680248,-0.467652904604665,
-0.409196012852459,-0.350739121100252,-0.263054619501813,-0.233826452302333,
-0.175370117903373,-0.116913783504413,-0.0584568917522064,0.),
 .UNSPECIFIED.);
#2904=B_SPLINE_CURVE_WITH_KNOTS('',3,(#69020,#69021,#69022,#69023,#69024,
#69025,#69026,#69027,#69028,#69029,#69030,#69031,#69032,#69033,#69034,#69035,
#69036,#69037,#69038,#69039,#69040,#69041,#69042,#69043,#69044,#69045,#69046,
#69047,#69048,#69049,#69050,#69051,#69052,#69053,#69054,#69055,#69056,#69057,
#69058,#69059,#69060,#69061,#69062,#69063,#69064,#69065,#69066,#69067,#69068,
#69069,#69070,#69071,#69072,#69073,#69074,#69075,#69076,#69077,#69078,#69079,
#69080,#69081,#69082,#69083,#69084,#69085,#69086,#69087,#69088,#69089,#69090,
#69091,#69092,#69093,#69094,#69095,#69096,#69097,#69098,#69099,#69100,#69101,
#69102,#69103,#69104,#69105,#69106,#69107,#69108,#69109,#69110,#69111,#69112,
#69113,#69114,#69115,#69116,#69117,#69118,#69119,#69120,#69121,#69122,#69123,
#69124,#69125,#69126,#69127,#69128,#69129,#69130,#69131,#69132,#69133,#69134),
 .UNSPECIFIED.,.F.,.F.,(4,3,3,3,3,3,3,3,3,3,3,3,3,3,3,3,3,3,3,3,3,3,3,3,
3,3,3,3,3,3,3,3,3,3,3,3,3,3,4),(-1.36616069392046,-1.31234511237088,-1.25590688369221,
-1.22043336320159,-1.19978988322529,-1.18977195970498,-1.18171686644571,
-1.12581307785687,-1.07017593161874,-1.02114732569299,-1.0124506254895,
-1.00557445843696,-0.972118719767242,-0.917136617675091,-0.861845521301615,
-0.806301914613285,-0.764644209597037,-0.752957249475711,-0.746332111135441,
-0.691988100457753,-0.639671094548295,-0.585206903159839,-0.530950162134808,
-0.504026220241107,-0.496690883172722,-0.490851144198066,-0.437265553293869,
-0.383730648991155,-0.330847439887809,-0.315558626985201,-0.276113798612051,
-0.258856686198798,-0.248596553131286,-0.240631547682685,-0.188137041660069,
-0.135346646621427,-0.0828734739367624,-0.0314201096525192,0.),
 .UNSPECIFIED.);
#2905=B_SPLINE_CURVE_WITH_KNOTS('',3,(#69135,#69136,#69137,#69138,#69139,
#69140,#69141,#69142,#69143,#69144,#69145,#69146,#69147,#69148,#69149,#69150,
#69151,#69152,#69153,#69154,#69155,#69156),.UNSPECIFIED.,.F.,.F.,(4,3,3,
3,3,3,3,4),(95.3678369910957,95.6931381963175,96.1915399577567,96.6899417191958,
97.188343480635,97.6867452420741,98.1851470035133,98.6057969367535),
 .UNSPECIFIED.);
#2906=B_SPLINE_CURVE_WITH_KNOTS('',3,(#69158,#69159,#69160,#69161,#69162,
#69163,#69164,#69165,#69166,#69167,#69168,#69169,#69170,#69171,#69172,#69173,
#69174,#69175,#69176,#69177,#69178,#69179,#69180,#69181,#69182,#69183,#69184,
#69185,#69186,#69187,#69188,#69189,#69190,#69191,#69192,#69193,#69194,#69195,
#69196,#69197,#69198,#69199,#69200,#69201,#69202,#69203,#69204,#69205,#69206,
#69207,#69208,#69209,#69210,#69211,#69212,#69213,#69214,#69215,#69216,#69217,
#69218,#69219,#69220,#69221,#69222,#69223,#69224,#69225,#69226,#69227,#69228,
#69229,#69230,#69231,#69232,#69233,#69234,#69235,#69236,#69237,#69238,#69239,
#69240,#69241,#69242,#69243,#69244,#69245,#69246,#69247,#69248,#69249,#69250,
#69251,#69252,#69253,#69254,#69255,#69256,#69257,#69258,#69259,#69260,#69261,
#69262,#69263,#69264,#69265,#69266,#69267,#69268,#69269),.UNSPECIFIED.,
 .F.,.F.,(4,3,3,3,3,3,3,3,3,3,3,3,3,3,3,3,3,3,3,3,3,3,3,3,3,3,3,3,3,3,3,
3,3,3,3,3,3,4),(-1.3692760959275,-1.32059746496365,-1.26831585127865,-1.23521527309061,
-1.21194803095155,-1.20083137328431,-1.14767293878112,-1.09434061971044,
-1.04892592274238,-1.04156502142363,-1.0342810920432,-1.00351122577432,
-0.950462707727008,-0.896724595787321,-0.841890453382919,-0.800764846579617,
-0.789580710740268,-0.783394562059837,-0.728633107476855,-0.677388026169712,
-0.622874329736254,-0.568068343407881,-0.53991042266811,-0.531693285272613,
-0.524470610547756,-0.469207417019949,-0.413568213634201,-0.358037807451751,
-0.342804977489712,-0.299954355303498,-0.281207208097029,-0.270867643373009,
-0.263531854817724,-0.208138358731652,-0.151751170205445,-0.0952554154038859,
-0.0393377089155784,0.),.UNSPECIFIED.);
#2907=B_SPLINE_CURVE_WITH_KNOTS('',3,(#69270,#69271,#69272,#69273,#69274,
#69275,#69276,#69277,#69278,#69279,#69280,#69281,#69282,#69283),
 .UNSPECIFIED.,.F.,.F.,(4,1,1,1,1,1,1,1,1,1,1,4),(10.3760794513229,10.7967293845631,
11.2951311460023,11.7935329074415,12.2919346688806,12.7903364303198,13.2887381917589,
13.7871399531981,14.2855417146372,14.7839434760764,15.2823452375155,15.7079632679489),
 .UNSPECIFIED.);
#2908=B_SPLINE_CURVE_WITH_KNOTS('',3,(#69289,#69290,#69291,#69292,#69293,
#69294,#69295,#69296,#69297,#69298,#69299,#69300,#69301,#69302,#69303,#69304,
#69305,#69306,#69307,#69308,#69309,#69310,#69311,#69312,#69313,#69314,#69315,
#69316,#69317,#69318,#69319,#69320,#69321,#69322,#69323,#69324,#69325,#69326,
#69327,#69328,#69329,#69330,#69331,#69332,#69333,#69334,#69335,#69336,#69337,
#69338,#69339,#69340,#69341,#69342,#69343,#69344,#69345,#69346,#69347,#69348,
#69349,#69350,#69351,#69352,#69353,#69354,#69355,#69356,#69357,#69358,#69359,
#69360,#69361,#69362,#69363,#69364,#69365,#69366,#69367,#69368,#69369,#69370,
#69371,#69372,#69373,#69374,#69375,#69376,#69377,#69378,#69379,#69380,#69381,
#69382,#69383,#69384,#69385,#69386,#69387,#69388,#69389,#69390,#69391,#69392,
#69393,#69394,#69395,#69396,#69397,#69398,#69399,#69400,#69401,#69402,#69403),
 .UNSPECIFIED.,.F.,.F.,(4,3,3,3,3,3,3,3,3,3,3,3,3,3,3,3,3,3,3,3,3,3,3,3,
3,3,3,3,3,3,3,3,3,3,3,3,3,3,4),(-1.36616069392045,-1.31234511237089,-1.25590688348171,
-1.2204333630174,-1.19978988220562,-1.18977196024391,-1.18171686684243,
-1.12581307864118,-1.0701759321844,-1.02114732597582,-1.01245062620987,
-1.00557445941498,-0.972118719767232,-0.917136616953618,-0.861845521732145,
-0.806301914936184,-0.764644209839213,-0.752957251104887,-0.74633211206392,
-0.691988105836551,-0.6396710945483,-0.58520690320579,-0.530950150202216,
-0.504026209800091,-0.49669074307685,-0.490850922101458,-0.437265330746164,
-0.383730417642567,-0.330847185660873,-0.315558626985216,-0.276113798612064,
-0.25885668619881,-0.248596553277842,-0.240631547783679,-0.188137027104224,
-0.135346638809626,-0.0828734852353619,-0.031420154055552,0.),
 .UNSPECIFIED.);
#2909=B_SPLINE_CURVE_WITH_KNOTS('',3,(#69406,#69407,#69408,#69409,#69410,
#69411,#69412,#69413,#69414,#69415,#69416,#69417),.UNSPECIFIED.,.F.,.F.,
(4,1,1,1,1,1,1,1,1,4),(11.6150691238055,12.1134708852447,12.6118726466838,
13.110274408123,13.6086761695621,14.1070779310013,14.6054796924404,15.1038814538796,
15.6022832153187,15.7079632679489),.UNSPECIFIED.);
#2910=B_SPLINE_CURVE_WITH_KNOTS('',3,(#70239,#70240,#70241,#70242,#70243,
#70244,#70245,#70246,#70247,#70248,#70249,#70250,#70251,#70252,#70253,#70254,
#70255,#70256,#70257,#70258,#70259,#70260,#70261,#70262,#70263,#70264,#70265,
#70266,#70267,#70268,#70269,#70270,#70271,#70272,#70273,#70274,#70275,#70276,
#70277,#70278,#70279,#70280,#70281,#70282,#70283,#70284,#70285,#70286,#70287,
#70288,#70289,#70290,#70291,#70292,#70293,#70294,#70295,#70296,#70297,#70298,
#70299,#70300,#70301,#70302,#70303,#70304,#70305,#70306,#70307,#70308,#70309,
#70310,#70311,#70312,#70313,#70314,#70315,#70316,#70317,#70318,#70319,#70320,
#70321,#70322,#70323,#70324,#70325,#70326,#70327,#70328,#70329,#70330,#70331,
#70332,#70333,#70334,#70335,#70336,#70337,#70338,#70339,#70340,#70341,#70342,
#70343,#70344,#70345,#70346,#70347,#70348,#70349,#70350),.UNSPECIFIED.,
 .F.,.F.,(4,3,3,3,3,3,3,3,3,3,3,3,3,3,3,3,3,3,3,3,3,3,3,3,3,3,3,3,3,3,3,
3,3,3,3,3,3,4),(-1.36927609592744,-1.32059746496358,-1.26831584736848,-1.2352152696692,
-1.21194802431441,-1.20083137389322,-1.14767293782772,-1.09434061945375,
-1.04892592261401,-1.0415650212466,-1.03428109205196,-1.00351122577428,
-0.950462711904765,-0.896724600945316,-0.841890457251413,-0.800764849480985,
-0.789580715694322,-0.78339457205448,-0.728633117749904,-0.677388026169701,
-0.622874336103501,-0.568068350793894,-0.539910429130868,-0.53169331053965,
-0.524470612233283,-0.469207425202408,-0.413568223926661,-0.358037807603194,
-0.342804977489683,-0.299954355303473,-0.281207208097006,-0.270867643816207,
-0.263531854461882,-0.208138335712682,-0.151751137623188,-0.0952553853759454,
-0.0393377021735775,0.),.UNSPECIFIED.);
#2911=B_SPLINE_CURVE_WITH_KNOTS('',3,(#70351,#70352,#70353,#70354,#70355,
#70356,#70357,#70358,#70359,#70360,#70361,#70362,#70363,#70364,#70365,#70366),
 .UNSPECIFIED.,.F.,.F.,(4,3,3,3,3,4),(-100.677155810709,-100.17875404927,
-99.6803522878307,-99.1819505263916,-98.6835487649524,-98.3406737518372),
 .UNSPECIFIED.);
#3566=FACE_BOUND('',#7062,.T.);
#3567=FACE_BOUND('',#7064,.T.);
#3568=FACE_BOUND('',#7067,.T.);
#3569=FACE_BOUND('',#7071,.T.);
#3570=FACE_BOUND('',#7081,.T.);
#3571=FACE_BOUND('',#7085,.T.);
#4990=FACE_OUTER_BOUND('',#7028,.T.);
#4991=FACE_OUTER_BOUND('',#7029,.T.);
#4992=FACE_OUTER_BOUND('',#7030,.T.);
#4993=FACE_OUTER_BOUND('',#7031,.T.);
#4994=FACE_OUTER_BOUND('',#7032,.T.);
#4995=FACE_OUTER_BOUND('',#7033,.T.);
#4996=FACE_OUTER_BOUND('',#7034,.T.);
#4997=FACE_OUTER_BOUND('',#7035,.T.);
#4998=FACE_OUTER_BOUND('',#7036,.T.);
#4999=FACE_OUTER_BOUND('',#7037,.T.);
#5000=FACE_OUTER_BOUND('',#7038,.T.);
#5001=FACE_OUTER_BOUND('',#7039,.T.);
#5002=FACE_OUTER_BOUND('',#7040,.T.);
#5003=FACE_OUTER_BOUND('',#7041,.T.);
#5004=FACE_OUTER_BOUND('',#7042,.T.);
#5005=FACE_OUTER_BOUND('',#7043,.T.);
#5006=FACE_OUTER_BOUND('',#7044,.T.);
#5007=FACE_OUTER_BOUND('',#7045,.T.);
#5008=FACE_OUTER_BOUND('',#7046,.T.);
#5009=FACE_OUTER_BOUND('',#7047,.T.);
#5010=FACE_OUTER_BOUND('',#7048,.T.);
#5011=FACE_OUTER_BOUND('',#7049,.T.);
#5012=FACE_OUTER_BOUND('',#7050,.T.);
#5013=FACE_OUTER_BOUND('',#7051,.T.);
#5014=FACE_OUTER_BOUND('',#7052,.T.);
#5015=FACE_OUTER_BOUND('',#7053,.T.);
#5016=FACE_OUTER_BOUND('',#7054,.T.);
#5017=FACE_OUTER_BOUND('',#7055,.T.);
#5018=FACE_OUTER_BOUND('',#7056,.T.);
#5019=FACE_OUTER_BOUND('',#7057,.T.);
#5020=FACE_OUTER_BOUND('',#7058,.T.);
#5021=FACE_OUTER_BOUND('',#7059,.T.);
#5022=FACE_OUTER_BOUND('',#7060,.T.);
#5023=FACE_OUTER_BOUND('',#7061,.T.);
#5024=FACE_OUTER_BOUND('',#7063,.T.);
#5025=FACE_OUTER_BOUND('',#7065,.T.);
#5026=FACE_OUTER_BOUND('',#7066,.T.);
#5027=FACE_OUTER_BOUND('',#7068,.T.);
#5028=FACE_OUTER_BOUND('',#7069,.T.);
#5029=FACE_OUTER_BOUND('',#7070,.T.);
#5030=FACE_OUTER_BOUND('',#7072,.T.);
#5031=FACE_OUTER_BOUND('',#7073,.T.);
#5032=FACE_OUTER_BOUND('',#7074,.T.);
#5033=FACE_OUTER_BOUND('',#7075,.T.);
#5034=FACE_OUTER_BOUND('',#7076,.T.);
#5035=FACE_OUTER_BOUND('',#7077,.T.);
#5036=FACE_OUTER_BOUND('',#7078,.T.);
#5037=FACE_OUTER_BOUND('',#7079,.T.);
#5038=FACE_OUTER_BOUND('',#7080,.T.);
#5039=FACE_OUTER_BOUND('',#7082,.T.);
#5040=FACE_OUTER_BOUND('',#7083,.T.);
#5041=FACE_OUTER_BOUND('',#7084,.T.);
#5042=FACE_OUTER_BOUND('',#7086,.T.);
#5043=FACE_OUTER_BOUND('',#7087,.T.);
#7028=EDGE_LOOP('',(#26163,#26164,#26165,#26166));
#7029=EDGE_LOOP('',(#26167,#26168,#26169,#26170));
#7030=EDGE_LOOP('',(#26171,#26172,#26173,#26174));
#7031=EDGE_LOOP('',(#26175,#26176,#26177,#26178));
#7032=EDGE_LOOP('',(#26179,#26180,#26181,#26182));
#7033=EDGE_LOOP('',(#26183,#26184,#26185,#26186));
#7034=EDGE_LOOP('',(#26187,#26188,#26189,#26190));
#7035=EDGE_LOOP('',(#26191,#26192,#26193,#26194));
#7036=EDGE_LOOP('',(#26195,#26196,#26197,#26198));
#7037=EDGE_LOOP('',(#26199,#26200,#26201,#26202));
#7038=EDGE_LOOP('',(#26203,#26204,#26205,#26206));
#7039=EDGE_LOOP('',(#26207,#26208,#26209,#26210));
#7040=EDGE_LOOP('',(#26211,#26212,#26213,#26214));
#7041=EDGE_LOOP('',(#26215,#26216,#26217,#26218));
#7042=EDGE_LOOP('',(#26219,#26220,#26221,#26222));
#7043=EDGE_LOOP('',(#26223,#26224,#26225,#26226));
#7044=EDGE_LOOP('',(#26227,#26228,#26229));
#7045=EDGE_LOOP('',(#26230,#26231,#26232,#26233,#26234));
#7046=EDGE_LOOP('',(#26235,#26236,#26237,#26238));
#7047=EDGE_LOOP('',(#26239,#26240,#26241,#26242));
#7048=EDGE_LOOP('',(#26243,#26244,#26245,#26246));
#7049=EDGE_LOOP('',(#26247,#26248,#26249,#26250));
#7050=EDGE_LOOP('',(#26251,#26252,#26253,#26254));
#7051=EDGE_LOOP('',(#26255,#26256,#26257,#26258));
#7052=EDGE_LOOP('',(#26259,#26260,#26261,#26262));
#7053=EDGE_LOOP('',(#26263,#26264,#26265,#26266));
#7054=EDGE_LOOP('',(#26267,#26268,#26269,#26270));
#7055=EDGE_LOOP('',(#26271,#26272,#26273,#26274));
#7056=EDGE_LOOP('',(#26275,#26276,#26277,#26278));
#7057=EDGE_LOOP('',(#26279,#26280,#26281,#26282));
#7058=EDGE_LOOP('',(#26283,#26284,#26285,#26286));
#7059=EDGE_LOOP('',(#26287,#26288,#26289,#26290));
#7060=EDGE_LOOP('',(#26291,#26292,#26293,#26294,#26295));
#7061=EDGE_LOOP('',(#26296,#26297,#26298,#26299,#26300,#26301));
#7062=EDGE_LOOP('',(#26302,#26303,#26304,#26305,#26306));
#7063=EDGE_LOOP('',(#26307));
#7064=EDGE_LOOP('',(#26308));
#7065=EDGE_LOOP('',(#26309,#26310,#26311,#26312,#26313));
#7066=EDGE_LOOP('',(#26314));
#7067=EDGE_LOOP('',(#26315));
#7068=EDGE_LOOP('',(#26316,#26317,#26318,#26319,#26320));
#7069=EDGE_LOOP('',(#26321,#26322,#26323,#26324,#26325,#26326,#26327,#26328,
#26329));
#7070=EDGE_LOOP('',(#26330,#26331,#26332,#26333));
#7071=EDGE_LOOP('',(#26334));
#7072=EDGE_LOOP('',(#26335,#26336,#26337,#26338,#26339,#26340,#26341,#26342,
#26343,#26344,#26345,#26346,#26347,#26348,#26349,#26350,#26351,#26352,#26353,
#26354,#26355,#26356,#26357,#26358,#26359,#26360,#26361,#26362,#26363,#26364,
#26365,#26366,#26367,#26368,#26369));
#7073=EDGE_LOOP('',(#26370,#26371,#26372,#26373,#26374));
#7074=EDGE_LOOP('',(#26375,#26376,#26377,#26378));
#7075=EDGE_LOOP('',(#26379,#26380,#26381,#26382,#26383,#26384,#26385,#26386,
#26387,#26388,#26389,#26390,#26391,#26392,#26393,#26394,#26395,#26396,#26397,
#26398,#26399,#26400,#26401,#26402,#26403,#26404,#26405,#26406,#26407,#26408,
#26409,#26410,#26411,#26412,#26413,#26414));
#7076=EDGE_LOOP('',(#26415,#26416));
#7077=EDGE_LOOP('',(#26417,#26418));
#7078=EDGE_LOOP('',(#26419,#26420,#26421,#26422,#26423,#26424));
#7079=EDGE_LOOP('',(#26425,#26426,#26427,#26428));
#7080=EDGE_LOOP('',(#26429));
#7081=EDGE_LOOP('',(#26430,#26431,#26432,#26433,#26434));
#7082=EDGE_LOOP('',(#26435,#26436,#26437,#26438));
#7083=EDGE_LOOP('',(#26439,#26440,#26441,#26442));
#7084=EDGE_LOOP('',(#26443));
#7085=EDGE_LOOP('',(#26444));
#7086=EDGE_LOOP('',(#26445,#26446,#26447,#26448));
#7087=EDGE_LOOP('',(#26449,#26450,#26451,#26452));
#9331=LINE('',#66055,#11637);
#9332=LINE('',#66088,#11638);
#9333=LINE('',#66172,#11639);
#9334=LINE('',#66262,#11640);
#9335=LINE('',#66352,#11641);
#9336=LINE('',#66436,#11642);
#9337=LINE('',#66526,#11643);
#9338=LINE('',#66610,#11644);
#9339=LINE('',#66700,#11645);
#9340=LINE('',#66790,#11646);
#9341=LINE('',#66874,#11647);
#9342=LINE('',#66964,#11648);
#9343=LINE('',#67048,#11649);
#9344=LINE('',#67138,#11650);
#9345=LINE('',#67228,#11651);
#9346=LINE('',#67312,#11652);
#9347=LINE('',#67402,#11653);
#9348=LINE('',#67412,#11654);
#9349=LINE('',#67449,#11655);
#9350=LINE('',#67486,#11656);
#9351=LINE('',#67523,#11657);
#9352=LINE('',#67561,#11658);
#9353=LINE('',#67598,#11659);
#9354=LINE('',#67635,#11660);
#9355=LINE('',#67672,#11661);
#9356=LINE('',#67709,#11662);
#9357=LINE('',#67747,#11663);
#9358=LINE('',#67784,#11664);
#9359=LINE('',#67821,#11665);
#9360=LINE('',#67858,#11666);
#9361=LINE('',#67895,#11667);
#9362=LINE('',#67933,#11668);
#9363=LINE('',#67971,#11669);
#9364=LINE('',#67980,#11670);
#9365=LINE('',#67997,#11671);
#9366=LINE('',#68009,#11672);
#9367=LINE('',#68015,#11673);
#9368=LINE('',#68130,#11674);
#9369=LINE('',#68190,#11675);
#9370=LINE('',#68197,#11676);
#9371=LINE('',#70370,#11677);
#9372=LINE('',#70377,#11678);
#9373=LINE('',#70381,#11679);
#9374=LINE('',#70388,#11680);
#9375=LINE('',#70390,#11681);
#11637=VECTOR('',#39400,7.);
#11638=VECTOR('',#39405,7.);
#11639=VECTOR('',#39408,7.);
#11640=VECTOR('',#39411,7.);
#11641=VECTOR('',#39414,7.);
#11642=VECTOR('',#39417,7.);
#11643=VECTOR('',#39420,7.);
#11644=VECTOR('',#39423,7.);
#11645=VECTOR('',#39426,7.);
#11646=VECTOR('',#39429,7.);
#11647=VECTOR('',#39432,7.);
#11648=VECTOR('',#39435,7.);
#11649=VECTOR('',#39438,7.);
#11650=VECTOR('',#39441,7.);
#11651=VECTOR('',#39444,7.);
#11652=VECTOR('',#39447,7.);
#11653=VECTOR('',#39450,6.21925);
#11654=VECTOR('',#39455,6.21925);
#11655=VECTOR('',#39460,6.21925);
#11656=VECTOR('',#39463,6.21925);
#11657=VECTOR('',#39466,6.21925);
#11658=VECTOR('',#39469,6.21925);
#11659=VECTOR('',#39472,6.21925);
#11660=VECTOR('',#39475,6.21925);
#11661=VECTOR('',#39478,6.21925);
#11662=VECTOR('',#39481,6.21925);
#11663=VECTOR('',#39484,6.21925);
#11664=VECTOR('',#39487,6.21925);
#11665=VECTOR('',#39490,6.21925);
#11666=VECTOR('',#39493,6.21925);
#11667=VECTOR('',#39496,6.21925);
#11668=VECTOR('',#39499,6.21925);
#11669=VECTOR('',#39504,5.3);
#11670=VECTOR('',#39515,5.05);
#11671=VECTOR('',#39516,10.);
#11672=VECTOR('',#39517,10.);
#11673=VECTOR('',#39524,5.3);
#11674=VECTOR('',#39531,10.);
#11675=VECTOR('',#39534,1.55);
#11676=VECTOR('',#39543,12.);
#11677=VECTOR('',#39562,6.65);
#11678=VECTOR('',#39573,11.75);
#11679=VECTOR('',#39578,11.75);
#11680=VECTOR('',#39587,8.);
#11681=VECTOR('',#39590,7.8);
#14218=VERTEX_POINT('',#66053);
#14219=VERTEX_POINT('',#66054);
#14220=VERTEX_POINT('',#66056);
#14221=VERTEX_POINT('',#66073);
#14222=VERTEX_POINT('',#66086);
#14223=VERTEX_POINT('',#66087);
#14224=VERTEX_POINT('',#66170);
#14225=VERTEX_POINT('',#66171);
#14226=VERTEX_POINT('',#66260);
#14227=VERTEX_POINT('',#66261);
#14228=VERTEX_POINT('',#66350);
#14229=VERTEX_POINT('',#66351);
#14230=VERTEX_POINT('',#66434);
#14231=VERTEX_POINT('',#66435);
#14232=VERTEX_POINT('',#66524);
#14233=VERTEX_POINT('',#66525);
#14234=VERTEX_POINT('',#66608);
#14235=VERTEX_POINT('',#66609);
#14236=VERTEX_POINT('',#66698);
#14237=VERTEX_POINT('',#66699);
#14238=VERTEX_POINT('',#66788);
#14239=VERTEX_POINT('',#66789);
#14240=VERTEX_POINT('',#66872);
#14241=VERTEX_POINT('',#66873);
#14242=VERTEX_POINT('',#66962);
#14243=VERTEX_POINT('',#66963);
#14244=VERTEX_POINT('',#67046);
#14245=VERTEX_POINT('',#67047);
#14246=VERTEX_POINT('',#67136);
#14247=VERTEX_POINT('',#67137);
#14248=VERTEX_POINT('',#67226);
#14249=VERTEX_POINT('',#67227);
#14250=VERTEX_POINT('',#67310);
#14251=VERTEX_POINT('',#67311);
#14252=VERTEX_POINT('',#67400);
#14253=VERTEX_POINT('',#67401);
#14254=VERTEX_POINT('',#67403);
#14255=VERTEX_POINT('',#67410);
#14256=VERTEX_POINT('',#67411);
#14257=VERTEX_POINT('',#67430);
#14258=VERTEX_POINT('',#67447);
#14259=VERTEX_POINT('',#67448);
#14260=VERTEX_POINT('',#67484);
#14261=VERTEX_POINT('',#67485);
#14262=VERTEX_POINT('',#67521);
#14263=VERTEX_POINT('',#67522);
#14264=VERTEX_POINT('',#67559);
#14265=VERTEX_POINT('',#67560);
#14266=VERTEX_POINT('',#67596);
#14267=VERTEX_POINT('',#67597);
#14268=VERTEX_POINT('',#67633);
#14269=VERTEX_POINT('',#67634);
#14270=VERTEX_POINT('',#67670);
#14271=VERTEX_POINT('',#67671);
#14272=VERTEX_POINT('',#67707);
#14273=VERTEX_POINT('',#67708);
#14274=VERTEX_POINT('',#67745);
#14275=VERTEX_POINT('',#67746);
#14276=VERTEX_POINT('',#67782);
#14277=VERTEX_POINT('',#67783);
#14278=VERTEX_POINT('',#67819);
#14279=VERTEX_POINT('',#67820);
#14280=VERTEX_POINT('',#67856);
#14281=VERTEX_POINT('',#67857);
#14282=VERTEX_POINT('',#67893);
#14283=VERTEX_POINT('',#67894);
#14284=VERTEX_POINT('',#67931);
#14285=VERTEX_POINT('',#67932);
#14286=VERTEX_POINT('',#67968);
#14287=VERTEX_POINT('',#67970);
#14288=VERTEX_POINT('',#67972);
#14289=VERTEX_POINT('',#67976);
#14290=VERTEX_POINT('',#67977);
#14291=VERTEX_POINT('',#67981);
#14292=VERTEX_POINT('',#67982);
#14293=VERTEX_POINT('',#67989);
#14294=VERTEX_POINT('',#67996);
#14295=VERTEX_POINT('',#67998);
#14296=VERTEX_POINT('',#68011);
#14297=VERTEX_POINT('',#68014);
#14298=VERTEX_POINT('',#68018);
#14299=VERTEX_POINT('',#68128);
#14300=VERTEX_POINT('',#68129);
#14301=VERTEX_POINT('',#68131);
#14302=VERTEX_POINT('',#68194);
#14303=VERTEX_POINT('',#68196);
#14304=VERTEX_POINT('',#69019);
#14305=VERTEX_POINT('',#69157);
#14306=VERTEX_POINT('',#69285);
#14307=VERTEX_POINT('',#69288);
#14308=VERTEX_POINT('',#70238);
#14309=VERTEX_POINT('',#70374);
#14310=VERTEX_POINT('',#70379);
#14311=VERTEX_POINT('',#70383);
#14312=VERTEX_POINT('',#70386);
#18303=EDGE_CURVE('',#14218,#14219,#9331,.T.);
#18304=EDGE_CURVE('',#14218,#14220,#2835,.T.);
#18305=EDGE_CURVE('',#14220,#14221,#1742,.T.);
#18306=EDGE_CURVE('',#14221,#14219,#2836,.T.);
#18307=EDGE_CURVE('',#14222,#14223,#9332,.T.);
#18308=EDGE_CURVE('',#14222,#14218,#2837,.T.);
#18309=EDGE_CURVE('',#14219,#14223,#2838,.T.);
#18310=EDGE_CURVE('',#14224,#14225,#9333,.T.);
#18311=EDGE_CURVE('',#14224,#14222,#2839,.T.);
#18312=EDGE_CURVE('',#14223,#14225,#2840,.T.);
#18313=EDGE_CURVE('',#14226,#14227,#9334,.T.);
#18314=EDGE_CURVE('',#14226,#14224,#2841,.T.);
#18315=EDGE_CURVE('',#14225,#14227,#2842,.T.);
#18316=EDGE_CURVE('',#14228,#14229,#9335,.T.);
#18317=EDGE_CURVE('',#14228,#14226,#2843,.T.);
#18318=EDGE_CURVE('',#14227,#14229,#2844,.T.);
#18319=EDGE_CURVE('',#14230,#14231,#9336,.T.);
#18320=EDGE_CURVE('',#14230,#14228,#2845,.T.);
#18321=EDGE_CURVE('',#14229,#14231,#2846,.T.);
#18322=EDGE_CURVE('',#14232,#14233,#9337,.T.);
#18323=EDGE_CURVE('',#14232,#14230,#2847,.T.);
#18324=EDGE_CURVE('',#14231,#14233,#2848,.T.);
#18325=EDGE_CURVE('',#14234,#14235,#9338,.T.);
#18326=EDGE_CURVE('',#14234,#14232,#2849,.T.);
#18327=EDGE_CURVE('',#14233,#14235,#2850,.T.);
#18328=EDGE_CURVE('',#14236,#14237,#9339,.T.);
#18329=EDGE_CURVE('',#14236,#14234,#2851,.T.);
#18330=EDGE_CURVE('',#14235,#14237,#2852,.T.);
#18331=EDGE_CURVE('',#14238,#14239,#9340,.T.);
#18332=EDGE_CURVE('',#14238,#14236,#2853,.T.);
#18333=EDGE_CURVE('',#14237,#14239,#2854,.T.);
#18334=EDGE_CURVE('',#14240,#14241,#9341,.T.);
#18335=EDGE_CURVE('',#14240,#14238,#2855,.T.);
#18336=EDGE_CURVE('',#14239,#14241,#2856,.T.);
#18337=EDGE_CURVE('',#14242,#14243,#9342,.T.);
#18338=EDGE_CURVE('',#14242,#14240,#2857,.T.);
#18339=EDGE_CURVE('',#14241,#14243,#2858,.T.);
#18340=EDGE_CURVE('',#14244,#14245,#9343,.T.);
#18341=EDGE_CURVE('',#14244,#14242,#2859,.T.);
#18342=EDGE_CURVE('',#14243,#14245,#2860,.T.);
#18343=EDGE_CURVE('',#14246,#14247,#9344,.T.);
#18344=EDGE_CURVE('',#14246,#14244,#2861,.T.);
#18345=EDGE_CURVE('',#14245,#14247,#2862,.T.);
#18346=EDGE_CURVE('',#14248,#14249,#9345,.T.);
#18347=EDGE_CURVE('',#14248,#14246,#2863,.T.);
#18348=EDGE_CURVE('',#14247,#14249,#2864,.T.);
#18349=EDGE_CURVE('',#14250,#14251,#9346,.T.);
#18350=EDGE_CURVE('',#14250,#14248,#2865,.T.);
#18351=EDGE_CURVE('',#14249,#14251,#2866,.T.);
#18352=EDGE_CURVE('',#14252,#14253,#9347,.T.);
#18353=EDGE_CURVE('',#14252,#14254,#2867,.T.);
#18354=EDGE_CURVE('',#14253,#14254,#1743,.T.);
#18355=EDGE_CURVE('',#14255,#14256,#9348,.T.);
#18356=EDGE_CURVE('',#14255,#14252,#2868,.T.);
#18357=EDGE_CURVE('',#14257,#14253,#1744,.T.);
#18358=EDGE_CURVE('',#14256,#14257,#2869,.T.);
#18359=EDGE_CURVE('',#14258,#14259,#9349,.T.);
#18360=EDGE_CURVE('',#14258,#14255,#2870,.T.);
#18361=EDGE_CURVE('',#14259,#14256,#2871,.T.);
#18362=EDGE_CURVE('',#14260,#14261,#9350,.T.);
#18363=EDGE_CURVE('',#14260,#14258,#2872,.T.);
#18364=EDGE_CURVE('',#14261,#14259,#2873,.T.);
#18365=EDGE_CURVE('',#14262,#14263,#9351,.T.);
#18366=EDGE_CURVE('',#14262,#14260,#2874,.T.);
#18367=EDGE_CURVE('',#14263,#14261,#2875,.T.);
#18368=EDGE_CURVE('',#14264,#14265,#9352,.T.);
#18369=EDGE_CURVE('',#14264,#14262,#2876,.T.);
#18370=EDGE_CURVE('',#14265,#14263,#2877,.T.);
#18371=EDGE_CURVE('',#14266,#14267,#9353,.T.);
#18372=EDGE_CURVE('',#14266,#14264,#2878,.T.);
#18373=EDGE_CURVE('',#14267,#14265,#2879,.T.);
#18374=EDGE_CURVE('',#14268,#14269,#9354,.T.);
#18375=EDGE_CURVE('',#14268,#14266,#2880,.T.);
#18376=EDGE_CURVE('',#14269,#14267,#2881,.T.);
#18377=EDGE_CURVE('',#14270,#14271,#9355,.T.);
#18378=EDGE_CURVE('',#14270,#14268,#2882,.T.);
#18379=EDGE_CURVE('',#14271,#14269,#2883,.T.);
#18380=EDGE_CURVE('',#14272,#14273,#9356,.T.);
#18381=EDGE_CURVE('',#14272,#14270,#2884,.T.);
#18382=EDGE_CURVE('',#14273,#14271,#2885,.T.);
#18383=EDGE_CURVE('',#14274,#14275,#9357,.T.);
#18384=EDGE_CURVE('',#14274,#14272,#2886,.T.);
#18385=EDGE_CURVE('',#14275,#14273,#2887,.T.);
#18386=EDGE_CURVE('',#14276,#14277,#9358,.T.);
#18387=EDGE_CURVE('',#14276,#14274,#2888,.T.);
#18388=EDGE_CURVE('',#14277,#14275,#2889,.T.);
#18389=EDGE_CURVE('',#14278,#14279,#9359,.T.);
#18390=EDGE_CURVE('',#14278,#14276,#2890,.T.);
#18391=EDGE_CURVE('',#14279,#14277,#2891,.T.);
#18392=EDGE_CURVE('',#14280,#14281,#9360,.T.);
#18393=EDGE_CURVE('',#14280,#14278,#2892,.T.);
#18394=EDGE_CURVE('',#14281,#14279,#2893,.T.);
#18395=EDGE_CURVE('',#14282,#14283,#9361,.T.);
#18396=EDGE_CURVE('',#14282,#14280,#2894,.T.);
#18397=EDGE_CURVE('',#14283,#14281,#2895,.T.);
#18398=EDGE_CURVE('',#14284,#14285,#9362,.T.);
#18399=EDGE_CURVE('',#14284,#14282,#2896,.T.);
#18400=EDGE_CURVE('',#14285,#14283,#2897,.T.);
#18401=EDGE_CURVE('',#14286,#14286,#1745,.T.);
#18402=EDGE_CURVE('',#14286,#14287,#9363,.T.);
#18403=EDGE_CURVE('',#14287,#14288,#1746,.T.);
#18404=EDGE_CURVE('',#14288,#14287,#1747,.T.);
#18405=EDGE_CURVE('',#14289,#14290,#1748,.T.);
#18406=EDGE_CURVE('',#14290,#14289,#1749,.T.);
#18407=EDGE_CURVE('',#14290,#14288,#9364,.T.);
#18408=EDGE_CURVE('',#14291,#14292,#2898,.T.);
#18409=EDGE_CURVE('',#14292,#14293,#2899,.T.);
#18410=EDGE_CURVE('',#14293,#14294,#9365,.T.);
#18411=EDGE_CURVE('',#14294,#14295,#2900,.T.);
#18412=EDGE_CURVE('',#14295,#14291,#9366,.T.);
#18413=EDGE_CURVE('',#14296,#14296,#1750,.T.);
#18414=EDGE_CURVE('',#14289,#14297,#9367,.T.);
#18415=EDGE_CURVE('',#14297,#14297,#1751,.T.);
#18416=EDGE_CURVE('',#14298,#14298,#1752,.T.);
#18417=EDGE_CURVE('',#14299,#14300,#9368,.T.);
#18418=EDGE_CURVE('',#14300,#14301,#2901,.T.);
#18419=EDGE_CURVE('',#14301,#14300,#2902,.T.);
#18420=EDGE_CURVE('',#14299,#14299,#2903,.T.);
#18421=EDGE_CURVE('',#14301,#14292,#9369,.T.);
#18422=EDGE_CURVE('',#14291,#14295,#1753,.T.);
#18423=EDGE_CURVE('',#14294,#14293,#1754,.T.);
#18424=EDGE_CURVE('',#14302,#14302,#1755,.T.);
#18425=EDGE_CURVE('',#14302,#14303,#9370,.T.);
#18426=EDGE_CURVE('',#14303,#14303,#1756,.T.);
#18427=EDGE_CURVE('',#14304,#14257,#2904,.T.);
#18428=EDGE_CURVE('',#14251,#14304,#2905,.T.);
#18429=EDGE_CURVE('',#14305,#14221,#2906,.T.);
#18430=EDGE_CURVE('',#14305,#14285,#2907,.T.);
#18431=EDGE_CURVE('',#14221,#14306,#1757,.T.);
#18432=EDGE_CURVE('',#14306,#14220,#1758,.T.);
#18433=EDGE_CURVE('',#14220,#14307,#2908,.T.);
#18434=EDGE_CURVE('',#14307,#14305,#1759,.T.);
#18435=EDGE_CURVE('',#14307,#14284,#2909,.T.);
#18436=EDGE_CURVE('',#14254,#14308,#2910,.T.);
#18437=EDGE_CURVE('',#14308,#14250,#2911,.T.);
#18438=EDGE_CURVE('',#14306,#14296,#9371,.T.);
#18439=EDGE_CURVE('',#14308,#14304,#1760,.T.);
#18440=EDGE_CURVE('',#14309,#14309,#1761,.T.);
#18441=EDGE_CURVE('',#14303,#14309,#9372,.T.);
#18442=EDGE_CURVE('',#14310,#14310,#1762,.T.);
#18443=EDGE_CURVE('',#14310,#14302,#9373,.T.);
#18444=EDGE_CURVE('',#14311,#14311,#1763,.T.);
#18445=EDGE_CURVE('',#14312,#14312,#1764,.T.);
#18446=EDGE_CURVE('',#14312,#14311,#9374,.T.);
#18447=EDGE_CURVE('',#14298,#14312,#9375,.T.);
#26163=ORIENTED_EDGE('',*,*,#18303,.F.);
#26164=ORIENTED_EDGE('',*,*,#18304,.T.);
#26165=ORIENTED_EDGE('',*,*,#18305,.T.);
#26166=ORIENTED_EDGE('',*,*,#18306,.T.);
#26167=ORIENTED_EDGE('',*,*,#18307,.F.);
#26168=ORIENTED_EDGE('',*,*,#18308,.T.);
#26169=ORIENTED_EDGE('',*,*,#18303,.T.);
#26170=ORIENTED_EDGE('',*,*,#18309,.T.);
#26171=ORIENTED_EDGE('',*,*,#18310,.F.);
#26172=ORIENTED_EDGE('',*,*,#18311,.T.);
#26173=ORIENTED_EDGE('',*,*,#18307,.T.);
#26174=ORIENTED_EDGE('',*,*,#18312,.T.);
#26175=ORIENTED_EDGE('',*,*,#18313,.F.);
#26176=ORIENTED_EDGE('',*,*,#18314,.T.);
#26177=ORIENTED_EDGE('',*,*,#18310,.T.);
#26178=ORIENTED_EDGE('',*,*,#18315,.T.);
#26179=ORIENTED_EDGE('',*,*,#18316,.F.);
#26180=ORIENTED_EDGE('',*,*,#18317,.T.);
#26181=ORIENTED_EDGE('',*,*,#18313,.T.);
#26182=ORIENTED_EDGE('',*,*,#18318,.T.);
#26183=ORIENTED_EDGE('',*,*,#18319,.F.);
#26184=ORIENTED_EDGE('',*,*,#18320,.T.);
#26185=ORIENTED_EDGE('',*,*,#18316,.T.);
#26186=ORIENTED_EDGE('',*,*,#18321,.T.);
#26187=ORIENTED_EDGE('',*,*,#18322,.F.);
#26188=ORIENTED_EDGE('',*,*,#18323,.T.);
#26189=ORIENTED_EDGE('',*,*,#18319,.T.);
#26190=ORIENTED_EDGE('',*,*,#18324,.T.);
#26191=ORIENTED_EDGE('',*,*,#18325,.F.);
#26192=ORIENTED_EDGE('',*,*,#18326,.T.);
#26193=ORIENTED_EDGE('',*,*,#18322,.T.);
#26194=ORIENTED_EDGE('',*,*,#18327,.T.);
#26195=ORIENTED_EDGE('',*,*,#18328,.F.);
#26196=ORIENTED_EDGE('',*,*,#18329,.T.);
#26197=ORIENTED_EDGE('',*,*,#18325,.T.);
#26198=ORIENTED_EDGE('',*,*,#18330,.T.);
#26199=ORIENTED_EDGE('',*,*,#18331,.F.);
#26200=ORIENTED_EDGE('',*,*,#18332,.T.);
#26201=ORIENTED_EDGE('',*,*,#18328,.T.);
#26202=ORIENTED_EDGE('',*,*,#18333,.T.);
#26203=ORIENTED_EDGE('',*,*,#18334,.F.);
#26204=ORIENTED_EDGE('',*,*,#18335,.T.);
#26205=ORIENTED_EDGE('',*,*,#18331,.T.);
#26206=ORIENTED_EDGE('',*,*,#18336,.T.);
#26207=ORIENTED_EDGE('',*,*,#18337,.F.);
#26208=ORIENTED_EDGE('',*,*,#18338,.T.);
#26209=ORIENTED_EDGE('',*,*,#18334,.T.);
#26210=ORIENTED_EDGE('',*,*,#18339,.T.);
#26211=ORIENTED_EDGE('',*,*,#18340,.F.);
#26212=ORIENTED_EDGE('',*,*,#18341,.T.);
#26213=ORIENTED_EDGE('',*,*,#18337,.T.);
#26214=ORIENTED_EDGE('',*,*,#18342,.T.);
#26215=ORIENTED_EDGE('',*,*,#18343,.F.);
#26216=ORIENTED_EDGE('',*,*,#18344,.T.);
#26217=ORIENTED_EDGE('',*,*,#18340,.T.);
#26218=ORIENTED_EDGE('',*,*,#18345,.T.);
#26219=ORIENTED_EDGE('',*,*,#18346,.F.);
#26220=ORIENTED_EDGE('',*,*,#18347,.T.);
#26221=ORIENTED_EDGE('',*,*,#18343,.T.);
#26222=ORIENTED_EDGE('',*,*,#18348,.T.);
#26223=ORIENTED_EDGE('',*,*,#18349,.F.);
#26224=ORIENTED_EDGE('',*,*,#18350,.T.);
#26225=ORIENTED_EDGE('',*,*,#18346,.T.);
#26226=ORIENTED_EDGE('',*,*,#18351,.T.);
#26227=ORIENTED_EDGE('',*,*,#18352,.F.);
#26228=ORIENTED_EDGE('',*,*,#18353,.T.);
#26229=ORIENTED_EDGE('',*,*,#18354,.F.);
#26230=ORIENTED_EDGE('',*,*,#18355,.F.);
#26231=ORIENTED_EDGE('',*,*,#18356,.T.);
#26232=ORIENTED_EDGE('',*,*,#18352,.T.);
#26233=ORIENTED_EDGE('',*,*,#18357,.F.);
#26234=ORIENTED_EDGE('',*,*,#18358,.F.);
#26235=ORIENTED_EDGE('',*,*,#18359,.F.);
#26236=ORIENTED_EDGE('',*,*,#18360,.T.);
#26237=ORIENTED_EDGE('',*,*,#18355,.T.);
#26238=ORIENTED_EDGE('',*,*,#18361,.F.);
#26239=ORIENTED_EDGE('',*,*,#18362,.F.);
#26240=ORIENTED_EDGE('',*,*,#18363,.T.);
#26241=ORIENTED_EDGE('',*,*,#18359,.T.);
#26242=ORIENTED_EDGE('',*,*,#18364,.F.);
#26243=ORIENTED_EDGE('',*,*,#18365,.F.);
#26244=ORIENTED_EDGE('',*,*,#18366,.T.);
#26245=ORIENTED_EDGE('',*,*,#18362,.T.);
#26246=ORIENTED_EDGE('',*,*,#18367,.F.);
#26247=ORIENTED_EDGE('',*,*,#18368,.F.);
#26248=ORIENTED_EDGE('',*,*,#18369,.T.);
#26249=ORIENTED_EDGE('',*,*,#18365,.T.);
#26250=ORIENTED_EDGE('',*,*,#18370,.F.);
#26251=ORIENTED_EDGE('',*,*,#18371,.F.);
#26252=ORIENTED_EDGE('',*,*,#18372,.T.);
#26253=ORIENTED_EDGE('',*,*,#18368,.T.);
#26254=ORIENTED_EDGE('',*,*,#18373,.F.);
#26255=ORIENTED_EDGE('',*,*,#18374,.F.);
#26256=ORIENTED_EDGE('',*,*,#18375,.T.);
#26257=ORIENTED_EDGE('',*,*,#18371,.T.);
#26258=ORIENTED_EDGE('',*,*,#18376,.F.);
#26259=ORIENTED_EDGE('',*,*,#18377,.F.);
#26260=ORIENTED_EDGE('',*,*,#18378,.T.);
#26261=ORIENTED_EDGE('',*,*,#18374,.T.);
#26262=ORIENTED_EDGE('',*,*,#18379,.F.);
#26263=ORIENTED_EDGE('',*,*,#18380,.F.);
#26264=ORIENTED_EDGE('',*,*,#18381,.T.);
#26265=ORIENTED_EDGE('',*,*,#18377,.T.);
#26266=ORIENTED_EDGE('',*,*,#18382,.F.);
#26267=ORIENTED_EDGE('',*,*,#18383,.F.);
#26268=ORIENTED_EDGE('',*,*,#18384,.T.);
#26269=ORIENTED_EDGE('',*,*,#18380,.T.);
#26270=ORIENTED_EDGE('',*,*,#18385,.F.);
#26271=ORIENTED_EDGE('',*,*,#18386,.F.);
#26272=ORIENTED_EDGE('',*,*,#18387,.T.);
#26273=ORIENTED_EDGE('',*,*,#18383,.T.);
#26274=ORIENTED_EDGE('',*,*,#18388,.F.);
#26275=ORIENTED_EDGE('',*,*,#18389,.F.);
#26276=ORIENTED_EDGE('',*,*,#18390,.T.);
#26277=ORIENTED_EDGE('',*,*,#18386,.T.);
#26278=ORIENTED_EDGE('',*,*,#18391,.F.);
#26279=ORIENTED_EDGE('',*,*,#18392,.F.);
#26280=ORIENTED_EDGE('',*,*,#18393,.T.);
#26281=ORIENTED_EDGE('',*,*,#18389,.T.);
#26282=ORIENTED_EDGE('',*,*,#18394,.F.);
#26283=ORIENTED_EDGE('',*,*,#18395,.F.);
#26284=ORIENTED_EDGE('',*,*,#18396,.T.);
#26285=ORIENTED_EDGE('',*,*,#18392,.T.);
#26286=ORIENTED_EDGE('',*,*,#18397,.F.);
#26287=ORIENTED_EDGE('',*,*,#18398,.F.);
#26288=ORIENTED_EDGE('',*,*,#18399,.T.);
#26289=ORIENTED_EDGE('',*,*,#18395,.T.);
#26290=ORIENTED_EDGE('',*,*,#18400,.F.);
#26291=ORIENTED_EDGE('',*,*,#18401,.T.);
#26292=ORIENTED_EDGE('',*,*,#18402,.T.);
#26293=ORIENTED_EDGE('',*,*,#18403,.T.);
#26294=ORIENTED_EDGE('',*,*,#18404,.T.);
#26295=ORIENTED_EDGE('',*,*,#18402,.F.);
#26296=ORIENTED_EDGE('',*,*,#18405,.F.);
#26297=ORIENTED_EDGE('',*,*,#18406,.F.);
#26298=ORIENTED_EDGE('',*,*,#18407,.T.);
#26299=ORIENTED_EDGE('',*,*,#18403,.F.);
#26300=ORIENTED_EDGE('',*,*,#18404,.F.);
#26301=ORIENTED_EDGE('',*,*,#18407,.F.);
#26302=ORIENTED_EDGE('',*,*,#18408,.T.);
#26303=ORIENTED_EDGE('',*,*,#18409,.T.);
#26304=ORIENTED_EDGE('',*,*,#18410,.T.);
#26305=ORIENTED_EDGE('',*,*,#18411,.T.);
#26306=ORIENTED_EDGE('',*,*,#18412,.T.);
#26307=ORIENTED_EDGE('',*,*,#18413,.F.);
#26308=ORIENTED_EDGE('',*,*,#18401,.F.);
#26309=ORIENTED_EDGE('',*,*,#18405,.T.);
#26310=ORIENTED_EDGE('',*,*,#18406,.T.);
#26311=ORIENTED_EDGE('',*,*,#18414,.T.);
#26312=ORIENTED_EDGE('',*,*,#18415,.T.);
#26313=ORIENTED_EDGE('',*,*,#18414,.F.);
#26314=ORIENTED_EDGE('',*,*,#18416,.T.);
#26315=ORIENTED_EDGE('',*,*,#18415,.F.);
#26316=ORIENTED_EDGE('',*,*,#18417,.T.);
#26317=ORIENTED_EDGE('',*,*,#18418,.T.);
#26318=ORIENTED_EDGE('',*,*,#18419,.T.);
#26319=ORIENTED_EDGE('',*,*,#18417,.F.);
#26320=ORIENTED_EDGE('',*,*,#18420,.T.);
#26321=ORIENTED_EDGE('',*,*,#18418,.F.);
#26322=ORIENTED_EDGE('',*,*,#18419,.F.);
#26323=ORIENTED_EDGE('',*,*,#18421,.T.);
#26324=ORIENTED_EDGE('',*,*,#18408,.F.);
#26325=ORIENTED_EDGE('',*,*,#18422,.T.);
#26326=ORIENTED_EDGE('',*,*,#18411,.F.);
#26327=ORIENTED_EDGE('',*,*,#18423,.T.);
#26328=ORIENTED_EDGE('',*,*,#18409,.F.);
#26329=ORIENTED_EDGE('',*,*,#18421,.F.);
#26330=ORIENTED_EDGE('',*,*,#18424,.F.);
#26331=ORIENTED_EDGE('',*,*,#18425,.T.);
#26332=ORIENTED_EDGE('',*,*,#18426,.T.);
#26333=ORIENTED_EDGE('',*,*,#18425,.F.);
#26334=ORIENTED_EDGE('',*,*,#18420,.F.);
#26335=ORIENTED_EDGE('',*,*,#18427,.F.);
#26336=ORIENTED_EDGE('',*,*,#18428,.F.);
#26337=ORIENTED_EDGE('',*,*,#18351,.F.);
#26338=ORIENTED_EDGE('',*,*,#18348,.F.);
#26339=ORIENTED_EDGE('',*,*,#18345,.F.);
#26340=ORIENTED_EDGE('',*,*,#18342,.F.);
#26341=ORIENTED_EDGE('',*,*,#18339,.F.);
#26342=ORIENTED_EDGE('',*,*,#18336,.F.);
#26343=ORIENTED_EDGE('',*,*,#18333,.F.);
#26344=ORIENTED_EDGE('',*,*,#18330,.F.);
#26345=ORIENTED_EDGE('',*,*,#18327,.F.);
#26346=ORIENTED_EDGE('',*,*,#18324,.F.);
#26347=ORIENTED_EDGE('',*,*,#18321,.F.);
#26348=ORIENTED_EDGE('',*,*,#18318,.F.);
#26349=ORIENTED_EDGE('',*,*,#18315,.F.);
#26350=ORIENTED_EDGE('',*,*,#18312,.F.);
#26351=ORIENTED_EDGE('',*,*,#18309,.F.);
#26352=ORIENTED_EDGE('',*,*,#18306,.F.);
#26353=ORIENTED_EDGE('',*,*,#18429,.F.);
#26354=ORIENTED_EDGE('',*,*,#18430,.T.);
#26355=ORIENTED_EDGE('',*,*,#18400,.T.);
#26356=ORIENTED_EDGE('',*,*,#18397,.T.);
#26357=ORIENTED_EDGE('',*,*,#18394,.T.);
#26358=ORIENTED_EDGE('',*,*,#18391,.T.);
#26359=ORIENTED_EDGE('',*,*,#18388,.T.);
#26360=ORIENTED_EDGE('',*,*,#18385,.T.);
#26361=ORIENTED_EDGE('',*,*,#18382,.T.);
#26362=ORIENTED_EDGE('',*,*,#18379,.T.);
#26363=ORIENTED_EDGE('',*,*,#18376,.T.);
#26364=ORIENTED_EDGE('',*,*,#18373,.T.);
#26365=ORIENTED_EDGE('',*,*,#18370,.T.);
#26366=ORIENTED_EDGE('',*,*,#18367,.T.);
#26367=ORIENTED_EDGE('',*,*,#18364,.T.);
#26368=ORIENTED_EDGE('',*,*,#18361,.T.);
#26369=ORIENTED_EDGE('',*,*,#18358,.T.);
#26370=ORIENTED_EDGE('',*,*,#18431,.T.);
#26371=ORIENTED_EDGE('',*,*,#18432,.T.);
#26372=ORIENTED_EDGE('',*,*,#18433,.T.);
#26373=ORIENTED_EDGE('',*,*,#18434,.T.);
#26374=ORIENTED_EDGE('',*,*,#18429,.T.);
#26375=ORIENTED_EDGE('',*,*,#18398,.T.);
#26376=ORIENTED_EDGE('',*,*,#18430,.F.);
#26377=ORIENTED_EDGE('',*,*,#18434,.F.);
#26378=ORIENTED_EDGE('',*,*,#18435,.T.);
#26379=ORIENTED_EDGE('',*,*,#18436,.F.);
#26380=ORIENTED_EDGE('',*,*,#18353,.F.);
#26381=ORIENTED_EDGE('',*,*,#18356,.F.);
#26382=ORIENTED_EDGE('',*,*,#18360,.F.);
#26383=ORIENTED_EDGE('',*,*,#18363,.F.);
#26384=ORIENTED_EDGE('',*,*,#18366,.F.);
#26385=ORIENTED_EDGE('',*,*,#18369,.F.);
#26386=ORIENTED_EDGE('',*,*,#18372,.F.);
#26387=ORIENTED_EDGE('',*,*,#18375,.F.);
#26388=ORIENTED_EDGE('',*,*,#18378,.F.);
#26389=ORIENTED_EDGE('',*,*,#18381,.F.);
#26390=ORIENTED_EDGE('',*,*,#18384,.F.);
#26391=ORIENTED_EDGE('',*,*,#18387,.F.);
#26392=ORIENTED_EDGE('',*,*,#18390,.F.);
#26393=ORIENTED_EDGE('',*,*,#18393,.F.);
#26394=ORIENTED_EDGE('',*,*,#18396,.F.);
#26395=ORIENTED_EDGE('',*,*,#18399,.F.);
#26396=ORIENTED_EDGE('',*,*,#18435,.F.);
#26397=ORIENTED_EDGE('',*,*,#18433,.F.);
#26398=ORIENTED_EDGE('',*,*,#18304,.F.);
#26399=ORIENTED_EDGE('',*,*,#18308,.F.);
#26400=ORIENTED_EDGE('',*,*,#18311,.F.);
#26401=ORIENTED_EDGE('',*,*,#18314,.F.);
#26402=ORIENTED_EDGE('',*,*,#18317,.F.);
#26403=ORIENTED_EDGE('',*,*,#18320,.F.);
#26404=ORIENTED_EDGE('',*,*,#18323,.F.);
#26405=ORIENTED_EDGE('',*,*,#18326,.F.);
#26406=ORIENTED_EDGE('',*,*,#18329,.F.);
#26407=ORIENTED_EDGE('',*,*,#18332,.F.);
#26408=ORIENTED_EDGE('',*,*,#18335,.F.);
#26409=ORIENTED_EDGE('',*,*,#18338,.F.);
#26410=ORIENTED_EDGE('',*,*,#18341,.F.);
#26411=ORIENTED_EDGE('',*,*,#18344,.F.);
#26412=ORIENTED_EDGE('',*,*,#18347,.F.);
#26413=ORIENTED_EDGE('',*,*,#18350,.F.);
#26414=ORIENTED_EDGE('',*,*,#18437,.F.);
#26415=ORIENTED_EDGE('',*,*,#18412,.F.);
#26416=ORIENTED_EDGE('',*,*,#18422,.F.);
#26417=ORIENTED_EDGE('',*,*,#18410,.F.);
#26418=ORIENTED_EDGE('',*,*,#18423,.F.);
#26419=ORIENTED_EDGE('',*,*,#18431,.F.);
#26420=ORIENTED_EDGE('',*,*,#18305,.F.);
#26421=ORIENTED_EDGE('',*,*,#18432,.F.);
#26422=ORIENTED_EDGE('',*,*,#18438,.T.);
#26423=ORIENTED_EDGE('',*,*,#18413,.T.);
#26424=ORIENTED_EDGE('',*,*,#18438,.F.);
#26425=ORIENTED_EDGE('',*,*,#18349,.T.);
#26426=ORIENTED_EDGE('',*,*,#18428,.T.);
#26427=ORIENTED_EDGE('',*,*,#18439,.F.);
#26428=ORIENTED_EDGE('',*,*,#18437,.T.);
#26429=ORIENTED_EDGE('',*,*,#18440,.F.);
#26430=ORIENTED_EDGE('',*,*,#18439,.T.);
#26431=ORIENTED_EDGE('',*,*,#18427,.T.);
#26432=ORIENTED_EDGE('',*,*,#18357,.T.);
#26433=ORIENTED_EDGE('',*,*,#18354,.T.);
#26434=ORIENTED_EDGE('',*,*,#18436,.T.);
#26435=ORIENTED_EDGE('',*,*,#18426,.F.);
#26436=ORIENTED_EDGE('',*,*,#18441,.T.);
#26437=ORIENTED_EDGE('',*,*,#18440,.T.);
#26438=ORIENTED_EDGE('',*,*,#18441,.F.);
#26439=ORIENTED_EDGE('',*,*,#18442,.F.);
#26440=ORIENTED_EDGE('',*,*,#18443,.T.);
#26441=ORIENTED_EDGE('',*,*,#18424,.T.);
#26442=ORIENTED_EDGE('',*,*,#18443,.F.);
#26443=ORIENTED_EDGE('',*,*,#18442,.T.);
#26444=ORIENTED_EDGE('',*,*,#18444,.F.);
#26445=ORIENTED_EDGE('',*,*,#18445,.F.);
#26446=ORIENTED_EDGE('',*,*,#18446,.T.);
#26447=ORIENTED_EDGE('',*,*,#18444,.T.);
#26448=ORIENTED_EDGE('',*,*,#18446,.F.);
#26449=ORIENTED_EDGE('',*,*,#18416,.F.);
#26450=ORIENTED_EDGE('',*,*,#18447,.T.);
#26451=ORIENTED_EDGE('',*,*,#18445,.T.);
#26452=ORIENTED_EDGE('',*,*,#18447,.F.);
#28822=PLANE('',#32950);
#28823=PLANE('',#32954);
#28824=PLANE('',#32962);
#28825=PLANE('',#32967);
#28826=PLANE('',#32968);
#28827=PLANE('',#32972);
#28828=PLANE('',#32977);
#30318=ADVANCED_FACE('',(#4990),#812,.T.);
#30319=ADVANCED_FACE('',(#4991),#813,.T.);
#30320=ADVANCED_FACE('',(#4992),#814,.T.);
#30321=ADVANCED_FACE('',(#4993),#815,.T.);
#30322=ADVANCED_FACE('',(#4994),#816,.T.);
#30323=ADVANCED_FACE('',(#4995),#817,.T.);
#30324=ADVANCED_FACE('',(#4996),#818,.T.);
#30325=ADVANCED_FACE('',(#4997),#819,.T.);
#30326=ADVANCED_FACE('',(#4998),#820,.T.);
#30327=ADVANCED_FACE('',(#4999),#821,.T.);
#30328=ADVANCED_FACE('',(#5000),#822,.T.);
#30329=ADVANCED_FACE('',(#5001),#823,.T.);
#30330=ADVANCED_FACE('',(#5002),#824,.T.);
#30331=ADVANCED_FACE('',(#5003),#825,.T.);
#30332=ADVANCED_FACE('',(#5004),#826,.T.);
#30333=ADVANCED_FACE('',(#5005),#827,.T.);
#30334=ADVANCED_FACE('',(#5006),#828,.T.);
#30335=ADVANCED_FACE('',(#5007),#829,.T.);
#30336=ADVANCED_FACE('',(#5008),#830,.T.);
#30337=ADVANCED_FACE('',(#5009),#831,.T.);
#30338=ADVANCED_FACE('',(#5010),#832,.T.);
#30339=ADVANCED_FACE('',(#5011),#833,.T.);
#30340=ADVANCED_FACE('',(#5012),#834,.T.);
#30341=ADVANCED_FACE('',(#5013),#835,.T.);
#30342=ADVANCED_FACE('',(#5014),#836,.T.);
#30343=ADVANCED_FACE('',(#5015),#837,.T.);
#30344=ADVANCED_FACE('',(#5016),#838,.T.);
#30345=ADVANCED_FACE('',(#5017),#839,.T.);
#30346=ADVANCED_FACE('',(#5018),#840,.T.);
#30347=ADVANCED_FACE('',(#5019),#841,.T.);
#30348=ADVANCED_FACE('',(#5020),#842,.T.);
#30349=ADVANCED_FACE('',(#5021),#843,.T.);
#30350=ADVANCED_FACE('',(#5022),#2055,.F.);
#30351=ADVANCED_FACE('',(#5023,#3566),#844,.F.);
#30352=ADVANCED_FACE('',(#5024,#3567),#28822,.T.);
#30353=ADVANCED_FACE('',(#5025),#2056,.F.);
#30354=ADVANCED_FACE('',(#5026,#3568),#28823,.T.);
#30355=ADVANCED_FACE('',(#5027),#426,.T.);
#30356=ADVANCED_FACE('',(#5028),#845,.F.);
#30357=ADVANCED_FACE('',(#5029,#3569),#846,.T.);
#30358=ADVANCED_FACE('',(#5030),#427,.F.);
#30359=ADVANCED_FACE('',(#5031),#28824,.T.);
#30360=ADVANCED_FACE('',(#5032),#847,.T.);
#30361=ADVANCED_FACE('',(#5033),#428,.F.);
#30362=ADVANCED_FACE('',(#5034),#28825,.T.);
#30363=ADVANCED_FACE('',(#5035),#28826,.T.);
#30364=ADVANCED_FACE('',(#5036),#2057,.T.);
#30365=ADVANCED_FACE('',(#5037),#848,.T.);
#30366=ADVANCED_FACE('',(#5038,#3570),#28827,.T.);
#30367=ADVANCED_FACE('',(#5039),#2058,.T.);
#30368=ADVANCED_FACE('',(#5040),#2059,.T.);
#30369=ADVANCED_FACE('',(#5041,#3571),#28828,.T.);
#30370=ADVANCED_FACE('',(#5042),#849,.T.);
#30371=ADVANCED_FACE('',(#5043),#2060,.T.);
#30676=CLOSED_SHELL('',(#30318,#30319,#30320,#30321,#30322,#30323,#30324,
#30325,#30326,#30327,#30328,#30329,#30330,#30331,#30332,#30333,#30334,#30335,
#30336,#30337,#30338,#30339,#30340,#30341,#30342,#30343,#30344,#30345,#30346,
#30347,#30348,#30349,#30350,#30351,#30352,#30353,#30354,#30355,#30356,#30357,
#30358,#30359,#30360,#30361,#30362,#30363,#30364,#30365,#30366,#30367,#30368,
#30369,#30370,#30371));
#32907=AXIS2_PLACEMENT_3D('',#66051,#39396,#39397);
#32908=AXIS2_PLACEMENT_3D('',#66052,#39398,#39399);
#32909=AXIS2_PLACEMENT_3D('',#66074,#39401,#39402);
#32910=AXIS2_PLACEMENT_3D('',#66085,#39403,#39404);
#32911=AXIS2_PLACEMENT_3D('',#66169,#39406,#39407);
#32912=AXIS2_PLACEMENT_3D('',#66259,#39409,#39410);
#32913=AXIS2_PLACEMENT_3D('',#66349,#39412,#39413);
#32914=AXIS2_PLACEMENT_3D('',#66433,#39415,#39416);
#32915=AXIS2_PLACEMENT_3D('',#66523,#39418,#39419);
#32916=AXIS2_PLACEMENT_3D('',#66607,#39421,#39422);
#32917=AXIS2_PLACEMENT_3D('',#66697,#39424,#39425);
#32918=AXIS2_PLACEMENT_3D('',#66787,#39427,#39428);
#32919=AXIS2_PLACEMENT_3D('',#66871,#39430,#39431);
#32920=AXIS2_PLACEMENT_3D('',#66961,#39433,#39434);
#32921=AXIS2_PLACEMENT_3D('',#67045,#39436,#39437);
#32922=AXIS2_PLACEMENT_3D('',#67135,#39439,#39440);
#32923=AXIS2_PLACEMENT_3D('',#67225,#39442,#39443);
#32924=AXIS2_PLACEMENT_3D('',#67309,#39445,#39446);
#32925=AXIS2_PLACEMENT_3D('',#67399,#39448,#39449);
#32926=AXIS2_PLACEMENT_3D('',#67408,#39451,#39452);
#32927=AXIS2_PLACEMENT_3D('',#67409,#39453,#39454);
#32928=AXIS2_PLACEMENT_3D('',#67431,#39456,#39457);
#32929=AXIS2_PLACEMENT_3D('',#67446,#39458,#39459);
#32930=AXIS2_PLACEMENT_3D('',#67483,#39461,#39462);
#32931=AXIS2_PLACEMENT_3D('',#67520,#39464,#39465);
#32932=AXIS2_PLACEMENT_3D('',#67558,#39467,#39468);
#32933=AXIS2_PLACEMENT_3D('',#67595,#39470,#39471);
#32934=AXIS2_PLACEMENT_3D('',#67632,#39473,#39474);
#32935=AXIS2_PLACEMENT_3D('',#67669,#39476,#39477);
#32936=AXIS2_PLACEMENT_3D('',#67706,#39479,#39480);
#32937=AXIS2_PLACEMENT_3D('',#67744,#39482,#39483);
#32938=AXIS2_PLACEMENT_3D('',#67781,#39485,#39486);
#32939=AXIS2_PLACEMENT_3D('',#67818,#39488,#39489);
#32940=AXIS2_PLACEMENT_3D('',#67855,#39491,#39492);
#32941=AXIS2_PLACEMENT_3D('',#67892,#39494,#39495);
#32942=AXIS2_PLACEMENT_3D('',#67930,#39497,#39498);
#32943=AXIS2_PLACEMENT_3D('',#67967,#39500,#39501);
#32944=AXIS2_PLACEMENT_3D('',#67969,#39502,#39503);
#32945=AXIS2_PLACEMENT_3D('',#67973,#39505,#39506);
#32946=AXIS2_PLACEMENT_3D('',#67974,#39507,#39508);
#32947=AXIS2_PLACEMENT_3D('',#67975,#39509,#39510);
#32948=AXIS2_PLACEMENT_3D('',#67978,#39511,#39512);
#32949=AXIS2_PLACEMENT_3D('',#67979,#39513,#39514);
#32950=AXIS2_PLACEMENT_3D('',#68010,#39518,#39519);
#32951=AXIS2_PLACEMENT_3D('',#68012,#39520,#39521);
#32952=AXIS2_PLACEMENT_3D('',#68013,#39522,#39523);
#32953=AXIS2_PLACEMENT_3D('',#68016,#39525,#39526);
#32954=AXIS2_PLACEMENT_3D('',#68017,#39527,#39528);
#32955=AXIS2_PLACEMENT_3D('',#68019,#39529,#39530);
#32956=AXIS2_PLACEMENT_3D('',#68189,#39532,#39533);
#32957=AXIS2_PLACEMENT_3D('',#68191,#39535,#39536);
#32958=AXIS2_PLACEMENT_3D('',#68192,#39537,#39538);
#32959=AXIS2_PLACEMENT_3D('',#68193,#39539,#39540);
#32960=AXIS2_PLACEMENT_3D('',#68195,#39541,#39542);
#32961=AXIS2_PLACEMENT_3D('',#68198,#39544,#39545);
#32962=AXIS2_PLACEMENT_3D('',#69284,#39546,#39547);
#32963=AXIS2_PLACEMENT_3D('',#69286,#39548,#39549);
#32964=AXIS2_PLACEMENT_3D('',#69287,#39550,#39551);
#32965=AXIS2_PLACEMENT_3D('',#69404,#39552,#39553);
#32966=AXIS2_PLACEMENT_3D('',#69405,#39554,#39555);
#32967=AXIS2_PLACEMENT_3D('',#70367,#39556,#39557);
#32968=AXIS2_PLACEMENT_3D('',#70368,#39558,#39559);
#32969=AXIS2_PLACEMENT_3D('',#70369,#39560,#39561);
#32970=AXIS2_PLACEMENT_3D('',#70371,#39563,#39564);
#32971=AXIS2_PLACEMENT_3D('',#70372,#39565,#39566);
#32972=AXIS2_PLACEMENT_3D('',#70373,#39567,#39568);
#32973=AXIS2_PLACEMENT_3D('',#70375,#39569,#39570);
#32974=AXIS2_PLACEMENT_3D('',#70376,#39571,#39572);
#32975=AXIS2_PLACEMENT_3D('',#70378,#39574,#39575);
#32976=AXIS2_PLACEMENT_3D('',#70380,#39576,#39577);
#32977=AXIS2_PLACEMENT_3D('',#70382,#39579,#39580);
#32978=AXIS2_PLACEMENT_3D('',#70384,#39581,#39582);
#32979=AXIS2_PLACEMENT_3D('',#70385,#39583,#39584);
#32980=AXIS2_PLACEMENT_3D('',#70387,#39585,#39586);
#32981=AXIS2_PLACEMENT_3D('',#70389,#39588,#39589);
#39396=DIRECTION('axis',(0.,0.,1.));
#39397=DIRECTION('refdir',(1.,0.,0.));
#39398=DIRECTION('center_axis',(1.,0.,0.));
#39399=DIRECTION('ref_axis',(0.,1.,0.));
#39400=DIRECTION('',(-1.,0.,0.));
#39401=DIRECTION('center_axis',(1.,0.,0.));
#39402=DIRECTION('ref_axis',(0.,1.,0.));
#39403=DIRECTION('center_axis',(1.,0.,0.));
#39404=DIRECTION('ref_axis',(0.,1.,0.));
#39405=DIRECTION('',(-1.,0.,0.));
#39406=DIRECTION('center_axis',(1.,0.,0.));
#39407=DIRECTION('ref_axis',(0.,1.,0.));
#39408=DIRECTION('',(-1.,0.,0.));
#39409=DIRECTION('center_axis',(1.,0.,0.));
#39410=DIRECTION('ref_axis',(0.,1.,0.));
#39411=DIRECTION('',(-1.,0.,0.));
#39412=DIRECTION('center_axis',(1.,0.,0.));
#39413=DIRECTION('ref_axis',(0.,1.,0.));
#39414=DIRECTION('',(-1.,0.,0.));
#39415=DIRECTION('center_axis',(1.,0.,0.));
#39416=DIRECTION('ref_axis',(0.,1.,0.));
#39417=DIRECTION('',(-1.,0.,0.));
#39418=DIRECTION('center_axis',(1.,0.,0.));
#39419=DIRECTION('ref_axis',(0.,1.,0.));
#39420=DIRECTION('',(-1.,0.,0.));
#39421=DIRECTION('center_axis',(1.,0.,0.));
#39422=DIRECTION('ref_axis',(0.,1.,0.));
#39423=DIRECTION('',(-1.,0.,0.));
#39424=DIRECTION('center_axis',(1.,0.,0.));
#39425=DIRECTION('ref_axis',(0.,1.,0.));
#39426=DIRECTION('',(-1.,0.,0.));
#39427=DIRECTION('center_axis',(1.,0.,0.));
#39428=DIRECTION('ref_axis',(0.,1.,0.));
#39429=DIRECTION('',(-1.,0.,0.));
#39430=DIRECTION('center_axis',(1.,0.,0.));
#39431=DIRECTION('ref_axis',(0.,1.,0.));
#39432=DIRECTION('',(-1.,0.,0.));
#39433=DIRECTION('center_axis',(1.,0.,0.));
#39434=DIRECTION('ref_axis',(0.,1.,0.));
#39435=DIRECTION('',(-1.,0.,0.));
#39436=DIRECTION('center_axis',(1.,0.,0.));
#39437=DIRECTION('ref_axis',(0.,1.,0.));
#39438=DIRECTION('',(-1.,0.,0.));
#39439=DIRECTION('center_axis',(1.,0.,0.));
#39440=DIRECTION('ref_axis',(0.,1.,0.));
#39441=DIRECTION('',(-1.,0.,0.));
#39442=DIRECTION('center_axis',(1.,0.,0.));
#39443=DIRECTION('ref_axis',(0.,1.,0.));
#39444=DIRECTION('',(-1.,0.,0.));
#39445=DIRECTION('center_axis',(1.,0.,0.));
#39446=DIRECTION('ref_axis',(0.,1.,0.));
#39447=DIRECTION('',(-1.,0.,0.));
#39448=DIRECTION('center_axis',(1.,0.,0.));
#39449=DIRECTION('ref_axis',(0.,-0.991226743157339,-0.132172401240557));
#39450=DIRECTION('',(1.,0.,0.));
#39451=DIRECTION('center_axis',(1.,0.,0.));
#39452=DIRECTION('ref_axis',(0.,1.,8.34422700308396E-14));
#39453=DIRECTION('center_axis',(1.,0.,0.));
#39454=DIRECTION('ref_axis',(0.,1.,8.34422700308396E-14));
#39455=DIRECTION('',(1.,0.,0.));
#39456=DIRECTION('center_axis',(1.,0.,0.));
#39457=DIRECTION('ref_axis',(0.,1.,8.34422700308396E-14));
#39458=DIRECTION('center_axis',(1.,0.,0.));
#39459=DIRECTION('ref_axis',(0.,1.,8.34422700308396E-14));
#39460=DIRECTION('',(1.,0.,0.));
#39461=DIRECTION('center_axis',(1.,0.,0.));
#39462=DIRECTION('ref_axis',(0.,1.,8.34422700308396E-14));
#39463=DIRECTION('',(1.,0.,0.));
#39464=DIRECTION('center_axis',(1.,0.,0.));
#39465=DIRECTION('ref_axis',(0.,1.,8.34422700308396E-14));
#39466=DIRECTION('',(1.,0.,0.));
#39467=DIRECTION('center_axis',(1.,0.,0.));
#39468=DIRECTION('ref_axis',(0.,1.,8.34422700308396E-14));
#39469=DIRECTION('',(1.,0.,0.));
#39470=DIRECTION('center_axis',(1.,0.,0.));
#39471=DIRECTION('ref_axis',(0.,1.,8.34422700308396E-14));
#39472=DIRECTION('',(1.,0.,0.));
#39473=DIRECTION('center_axis',(1.,0.,0.));
#39474=DIRECTION('ref_axis',(0.,1.,8.34422700308396E-14));
#39475=DIRECTION('',(1.,0.,0.));
#39476=DIRECTION('center_axis',(1.,0.,0.));
#39477=DIRECTION('ref_axis',(0.,1.,8.34422700308396E-14));
#39478=DIRECTION('',(1.,0.,0.));
#39479=DIRECTION('center_axis',(1.,0.,0.));
#39480=DIRECTION('ref_axis',(0.,1.,8.34422700308396E-14));
#39481=DIRECTION('',(1.,0.,0.));
#39482=DIRECTION('center_axis',(1.,0.,0.));
#39483=DIRECTION('ref_axis',(0.,1.,8.34422700308396E-14));
#39484=DIRECTION('',(1.,0.,0.));
#39485=DIRECTION('center_axis',(1.,0.,0.));
#39486=DIRECTION('ref_axis',(0.,1.,8.34422700308396E-14));
#39487=DIRECTION('',(1.,0.,0.));
#39488=DIRECTION('center_axis',(1.,0.,0.));
#39489=DIRECTION('ref_axis',(0.,1.,8.34422700308396E-14));
#39490=DIRECTION('',(1.,0.,0.));
#39491=DIRECTION('center_axis',(1.,0.,0.));
#39492=DIRECTION('ref_axis',(0.,1.,8.34422700308396E-14));
#39493=DIRECTION('',(1.,0.,0.));
#39494=DIRECTION('center_axis',(1.,0.,0.));
#39495=DIRECTION('ref_axis',(0.,1.,8.34422700308396E-14));
#39496=DIRECTION('',(1.,0.,0.));
#39497=DIRECTION('center_axis',(1.,0.,0.));
#39498=DIRECTION('ref_axis',(0.,1.,8.34422700308396E-14));
#39499=DIRECTION('',(1.,0.,0.));
#39500=DIRECTION('center_axis',(-1.,0.,0.));
#39501=DIRECTION('ref_axis',(0.,-1.,0.));
#39502=DIRECTION('center_axis',(-1.,0.,0.));
#39503=DIRECTION('ref_axis',(0.,-1.,0.));
#39504=DIRECTION('',(0.707106781186547,-0.707106781186547,8.65956056235493E-17));
#39505=DIRECTION('center_axis',(1.,0.,0.));
#39506=DIRECTION('ref_axis',(0.,-1.,0.));
#39507=DIRECTION('center_axis',(1.,0.,0.));
#39508=DIRECTION('ref_axis',(0.,-1.,0.));
#39509=DIRECTION('center_axis',(1.,0.,0.));
#39510=DIRECTION('ref_axis',(0.,1.,0.));
#39511=DIRECTION('center_axis',(-1.,0.,0.));
#39512=DIRECTION('ref_axis',(0.,-1.,0.));
#39513=DIRECTION('center_axis',(-1.,0.,0.));
#39514=DIRECTION('ref_axis',(0.,-1.,0.));
#39515=DIRECTION('',(-1.,0.,0.));
#39516=DIRECTION('',(1.,0.,0.));
#39517=DIRECTION('',(-1.,0.,0.));
#39518=DIRECTION('center_axis',(-1.,0.,0.));
#39519=DIRECTION('ref_axis',(0.,0.,1.));
#39520=DIRECTION('center_axis',(1.,0.,0.));
#39521=DIRECTION('ref_axis',(0.,0.,-1.));
#39522=DIRECTION('center_axis',(1.,0.,0.));
#39523=DIRECTION('ref_axis',(0.,-1.,0.));
#39524=DIRECTION('',(0.707106781186547,0.707106781186547,-8.65956056235493E-17));
#39525=DIRECTION('center_axis',(1.,0.,0.));
#39526=DIRECTION('ref_axis',(0.,-1.,0.));
#39527=DIRECTION('center_axis',(1.,0.,0.));
#39528=DIRECTION('ref_axis',(0.,0.,-1.));
#39529=DIRECTION('center_axis',(1.,0.,0.));
#39530=DIRECTION('ref_axis',(0.,0.,-1.));
#39531=DIRECTION('',(0.,-0.651997912940355,0.758220760413101));
#39532=DIRECTION('center_axis',(0.,-1.,0.));
#39533=DIRECTION('ref_axis',(1.,0.,0.));
#39534=DIRECTION('',(0.,-1.,0.));
#39535=DIRECTION('center_axis',(0.,-1.,0.));
#39536=DIRECTION('ref_axis',(1.,0.,0.));
#39537=DIRECTION('center_axis',(0.,-1.,0.));
#39538=DIRECTION('ref_axis',(1.,0.,0.));
#39539=DIRECTION('center_axis',(1.,0.,0.));
#39540=DIRECTION('ref_axis',(0.,1.,0.));
#39541=DIRECTION('center_axis',(1.,0.,0.));
#39542=DIRECTION('ref_axis',(0.,0.,-1.));
#39543=DIRECTION('',(-1.,0.,0.));
#39544=DIRECTION('center_axis',(1.,0.,0.));
#39545=DIRECTION('ref_axis',(0.,0.,-1.));
#39546=DIRECTION('center_axis',(1.,0.,0.));
#39547=DIRECTION('ref_axis',(0.,0.,-1.));
#39548=DIRECTION('center_axis',(1.,0.,0.));
#39549=DIRECTION('ref_axis',(0.,1.,0.));
#39550=DIRECTION('center_axis',(1.,0.,0.));
#39551=DIRECTION('ref_axis',(0.,1.,0.));
#39552=DIRECTION('center_axis',(-1.,0.,0.));
#39553=DIRECTION('ref_axis',(0.,1.,8.34422700308396E-14));
#39554=DIRECTION('center_axis',(1.,0.,0.));
#39555=DIRECTION('ref_axis',(0.,0.888994820201767,0.457917251972918));
#39556=DIRECTION('center_axis',(0.,1.,0.));
#39557=DIRECTION('ref_axis',(1.,0.,0.));
#39558=DIRECTION('center_axis',(0.,1.,0.));
#39559=DIRECTION('ref_axis',(1.,0.,0.));
#39560=DIRECTION('center_axis',(1.,0.,0.));
#39561=DIRECTION('ref_axis',(0.,1.,0.));
#39562=DIRECTION('',(-0.707106781186548,0.707106781186547,8.65956056235493E-17));
#39563=DIRECTION('center_axis',(1.,0.,0.));
#39564=DIRECTION('ref_axis',(0.,0.0481637001355167,-0.998839455562933));
#39565=DIRECTION('center_axis',(1.,0.,0.));
#39566=DIRECTION('ref_axis',(0.,1.,0.));
#39567=DIRECTION('center_axis',(-1.,0.,0.));
#39568=DIRECTION('ref_axis',(0.,0.,1.));
#39569=DIRECTION('center_axis',(1.,0.,0.));
#39570=DIRECTION('ref_axis',(0.,0.,-1.));
#39571=DIRECTION('center_axis',(1.,0.,0.));
#39572=DIRECTION('ref_axis',(0.,1.,0.));
#39573=DIRECTION('',(-0.707106781186547,0.707106781186548,8.65956056235493E-17));
#39574=DIRECTION('center_axis',(-1.,0.,0.));
#39575=DIRECTION('ref_axis',(0.,1.,0.));
#39576=DIRECTION('center_axis',(1.,0.,0.));
#39577=DIRECTION('ref_axis',(0.,0.,-1.));
#39578=DIRECTION('',(-0.707106781186547,-0.707106781186548,-8.65956056235493E-17));
#39579=DIRECTION('center_axis',(1.,0.,0.));
#39580=DIRECTION('ref_axis',(0.,0.,-1.));
#39581=DIRECTION('center_axis',(1.,0.,0.));
#39582=DIRECTION('ref_axis',(0.,0.,-1.));
#39583=DIRECTION('center_axis',(1.,0.,0.));
#39584=DIRECTION('ref_axis',(0.,1.,0.));
#39585=DIRECTION('center_axis',(1.,0.,0.));
#39586=DIRECTION('ref_axis',(0.,0.,-1.));
#39587=DIRECTION('',(-1.,0.,0.));
#39588=DIRECTION('center_axis',(-1.,0.,0.));
#39589=DIRECTION('ref_axis',(0.,1.,0.));
#39590=DIRECTION('',(-0.707106781186546,-0.70710678118655,-8.65956056235496E-17));
#66051=CARTESIAN_POINT('',(0.,0.,0.));
#66052=CARTESIAN_POINT('Origin',(-3.775,0.,0.));
#66053=CARTESIAN_POINT('',(-13.2148283363937,-6.93306764378165,0.000177865042129965));
#66054=CARTESIAN_POINT('',(-13.3941716636063,-6.93294642624908,0.000111209669744707));
#66055=CARTESIAN_POINT('',(-3.775,-6.933,-8.4904762584886E-16));
#66056=CARTESIAN_POINT('',(-13.617,3.02035542106413,6.24066579987949));
#66057=CARTESIAN_POINT('Ctrl Pts',(-13.2148283363937,-6.93306764378165,
0.000177865042129965));
#66058=CARTESIAN_POINT('Ctrl Pts',(-13.2218364625447,-6.93331928540806,
0.244392711657743));
#66059=CARTESIAN_POINT('Ctrl Pts',(-13.2288445886957,-6.92066616143694,
0.488581520566852));
#66060=CARTESIAN_POINT('Ctrl Pts',(-13.2358527148466,-6.89491117443486,
0.731380409494485));
#66061=CARTESIAN_POINT('Ctrl Pts',(-13.2689040081711,-6.77344708950859,
1.87645358939269));
#66062=CARTESIAN_POINT('Ctrl Pts',(-13.3019553014956,-6.36057186435389,
2.99061222182));
#66063=CARTESIAN_POINT('Ctrl Pts',(-13.33500659482,-5.70651333434507,3.93832482936462));
#66064=CARTESIAN_POINT('Ctrl Pts',(-13.3680578881445,-5.05245480433625,
4.88603743690924));
#66065=CARTESIAN_POINT('Ctrl Pts',(-13.401109181469,-4.15721296947331,5.66730401957118));
#66066=CARTESIAN_POINT('Ctrl Pts',(-13.4341604747935,-3.12969490598308,
6.18706519987829));
#66067=CARTESIAN_POINT('Ctrl Pts',(-13.467211768118,-2.10217684249286,6.7068263801854));
#66068=CARTESIAN_POINT('Ctrl Pts',(-13.5002630614424,-0.942382550375355,
6.96508215813768));
#66069=CARTESIAN_POINT('Ctrl Pts',(-13.5333143547669,0.208594027287818,
6.93044705647606));
#66070=CARTESIAN_POINT('Ctrl Pts',(-13.5612095698446,1.18001559521549,6.90121511082712));
#66071=CARTESIAN_POINT('Ctrl Pts',(-13.5891047849223,2.14515602214522,6.66334759170891));
#66072=CARTESIAN_POINT('Ctrl Pts',(-13.617,3.02048254223755,6.24076191290031));
#66073=CARTESIAN_POINT('',(-13.617,-3.02022829989073,6.24056968685866));
#66074=CARTESIAN_POINT('Origin',(-13.617,0.,0.));
#66075=CARTESIAN_POINT('Ctrl Pts',(-13.617,-3.0202282998907,6.24056968685867));
#66076=CARTESIAN_POINT('Ctrl Pts',(-13.5839487066755,-4.0569986079954,5.73880731865404));
#66077=CARTESIAN_POINT('Ctrl Pts',(-13.550897413351,-4.96580358103262,4.97396809622495));
#66078=CARTESIAN_POINT('Ctrl Pts',(-13.5178461200266,-5.63641088424476,
4.03806620002614));
#66079=CARTESIAN_POINT('Ctrl Pts',(-13.4847948267021,-6.30701818745691,
3.10216430382733));
#66080=CARTESIAN_POINT('Ctrl Pts',(-13.4517435333776,-6.73942782084398,
1.9951997338588));
#66081=CARTESIAN_POINT('Ctrl Pts',(-13.4186922400531,-6.8809997664126,0.852378123583212));
#66082=CARTESIAN_POINT('Ctrl Pts',(-13.4105187145708,-6.91601025430248,
0.569760391756853));
#66083=CARTESIAN_POINT('Ctrl Pts',(-13.4023451890886,-6.93323415571197,
0.284949772367894));
#66084=CARTESIAN_POINT('Ctrl Pts',(-13.3941716636063,-6.93294642624908,
0.000111209669744707));
#66085=CARTESIAN_POINT('Origin',(-3.775,0.,0.));
#66086=CARTESIAN_POINT('',(-11.9648283363937,-6.93317898118896,-0.000167065473373196));
#66087=CARTESIAN_POINT('',(-12.1441716636063,-6.93330133372241,-0.00014816709062256));
#66088=CARTESIAN_POINT('',(-3.775,-6.933,-8.4904762584886E-16));
#66089=CARTESIAN_POINT('Ctrl Pts',(-11.9648283363937,-6.93317898118896,
-0.000167065473373196));
#66090=CARTESIAN_POINT('Ctrl Pts',(-11.9918876093176,-6.93222498183581,
0.942733971459933));
#66091=CARTESIAN_POINT('Ctrl Pts',(-12.0189468822415,-6.7384283406596,1.88601512439082));
#66092=CARTESIAN_POINT('Ctrl Pts',(-12.0460061551654,-6.36433591287228,
2.75135297573217));
#66093=CARTESIAN_POINT('Ctrl Pts',(-12.0790574484899,-5.90740425044193,
3.80831172070338));
#66094=CARTESIAN_POINT('Ctrl Pts',(-12.1121087418143,-5.18148623385836,
4.74898552680103));
#66095=CARTESIAN_POINT('Ctrl Pts',(-12.1451600351388,-4.27489147628079,
5.45893924348122));
#66096=CARTESIAN_POINT('Ctrl Pts',(-12.1782113284633,-3.36829671870322,
6.16889296016141));
#66097=CARTESIAN_POINT('Ctrl Pts',(-12.2112626217878,-2.28102522013168,
6.64812658742415));
#66098=CARTESIAN_POINT('Ctrl Pts',(-12.2443139151122,-1.14534608355589,
6.83834023540624));
#66099=CARTESIAN_POINT('Ctrl Pts',(-12.2773652084367,-0.00966694698010501,
7.02855388338833));
#66100=CARTESIAN_POINT('Ctrl Pts',(-12.3104165017612,1.17441982759993,6.92974755208976));
#66101=CARTESIAN_POINT('Ctrl Pts',(-12.3434677950857,2.26286733274423,6.55394127266096));
#66102=CARTESIAN_POINT('Ctrl Pts',(-12.3765190884102,3.35131483788853,6.17813499323216));
#66103=CARTESIAN_POINT('Ctrl Pts',(-12.4095703817346,4.34412307359712,5.52532876567314));
#66104=CARTESIAN_POINT('Ctrl Pts',(-12.4426216750591,5.12051461339035,4.67493796181516));
#66105=CARTESIAN_POINT('Ctrl Pts',(-12.4756729683836,5.89690615318357,3.82454715795718));
#66106=CARTESIAN_POINT('Ctrl Pts',(-12.5087242617081,6.45688099706144,2.77657177780023));
#66107=CARTESIAN_POINT('Ctrl Pts',(-12.5417755550326,6.73231690145685,1.65850050356931));
#66108=CARTESIAN_POINT('Ctrl Pts',(-12.574826848357,7.00775280585226,0.540429229338383));
#66109=CARTESIAN_POINT('Ctrl Pts',(-12.6078781416815,6.99864977076521,-0.647737938966518));
#66110=CARTESIAN_POINT('Ctrl Pts',(-12.640929435006,6.7061152074704,-1.7614577884509));
#66111=CARTESIAN_POINT('Ctrl Pts',(-12.6739807283305,6.41358064417558,-2.87517763793529));
#66112=CARTESIAN_POINT('Ctrl Pts',(-12.707032021655,5.83761455267299,-3.91445016859917));
#66113=CARTESIAN_POINT('Ctrl Pts',(-12.7400833149794,5.04828453444703,-4.75284530198096));
#66114=CARTESIAN_POINT('Ctrl Pts',(-12.7731346083039,4.25895451622106,-5.59124043536275));
#66115=CARTESIAN_POINT('Ctrl Pts',(-12.8061859016284,3.25626057127172,-6.22875817146247));
#66116=CARTESIAN_POINT('Ctrl Pts',(-12.8392371949529,2.16218276932853,-6.5878433086778));
#66117=CARTESIAN_POINT('Ctrl Pts',(-12.8722884882773,1.06810496738535,-6.94692844589313));
#66118=CARTESIAN_POINT('Ctrl Pts',(-12.9053397816018,-0.117356691551664,
-7.02758098422409));
#66119=CARTESIAN_POINT('Ctrl Pts',(-12.9383910749263,-1.24998808595104,
-6.81998875087525));
#66120=CARTESIAN_POINT('Ctrl Pts',(-12.9714423682508,-2.38261948035043,
-6.6123965175264));
#66121=CARTESIAN_POINT('Ctrl Pts',(-13.0044936615752,-3.46242061021218,
-6.11655951249774));
#66122=CARTESIAN_POINT('Ctrl Pts',(-13.0375449548997,-4.35803107659019,
-5.39279862959555));
#66123=CARTESIAN_POINT('Ctrl Pts',(-13.0705962482242,-5.25364154296821,
-4.66903774669337));
#66124=CARTESIAN_POINT('Ctrl Pts',(-13.1036475415487,-5.96506134586249,
-3.71735298591766));
#66125=CARTESIAN_POINT('Ctrl Pts',(-13.1366988348732,-6.40574477496072,
-2.65351674184525));
#66126=CARTESIAN_POINT('Ctrl Pts',(-13.1627420020467,-6.75298662422614,
-1.81525407909162));
#66127=CARTESIAN_POINT('Ctrl Pts',(-13.1887851692202,-6.93213250865378,
-0.907358320760865));
#66128=CARTESIAN_POINT('Ctrl Pts',(-13.2148283363937,-6.93306764378165,
0.000177865042129965));
#66129=CARTESIAN_POINT('Ctrl Pts',(-13.3941716636063,-6.93294642624908,
0.000111209669744707));
#66130=CARTESIAN_POINT('Ctrl Pts',(-13.3692938957641,-6.93207066378957,
-0.866852213967783));
#66131=CARTESIAN_POINT('Ctrl Pts',(-13.3444161279219,-6.76896512341342,
-1.73407450766015));
#66132=CARTESIAN_POINT('Ctrl Pts',(-13.3195383600797,-6.45138278311444,
-2.54051030748334));
#66133=CARTESIAN_POINT('Ctrl Pts',(-13.2864870667552,-6.02945959649748,
-3.61189847769166));
#66134=CARTESIAN_POINT('Ctrl Pts',(-13.2534357734307,-5.33487896551338,
-4.57599616752565));
#66135=CARTESIAN_POINT('Ctrl Pts',(-13.2203844801063,-4.45212669250648,
-5.31539786545727));
#66136=CARTESIAN_POINT('Ctrl Pts',(-13.1873331867818,-3.56937441949959,
-6.05479956338889));
#66137=CARTESIAN_POINT('Ctrl Pts',(-13.1542818934573,-2.49845050446989,
-6.56950526941814));
#66138=CARTESIAN_POINT('Ctrl Pts',(-13.1212306001328,-1.36964132464014,
-6.79696181781881));
#66139=CARTESIAN_POINT('Ctrl Pts',(-13.0881793068083,-0.240832144810394,
-7.02441836621948));
#66140=CARTESIAN_POINT('Ctrl Pts',(-13.0551280134839,0.945862299819417,
-6.96462575699158));
#66141=CARTESIAN_POINT('Ctrl Pts',(-13.0220767201594,2.04608097294984,-6.62482593361867));
#66142=CARTESIAN_POINT('Ctrl Pts',(-12.9890254268349,3.14629964608026,-6.28502611024576));
#66143=CARTESIAN_POINT('Ctrl Pts',(-12.9559741335104,4.1600425477113,-5.66521907272784));
#66144=CARTESIAN_POINT('Ctrl Pts',(-12.922922840186,4.96398389811699,-4.84082229058768));
#66145=CARTESIAN_POINT('Ctrl Pts',(-12.8898715468615,5.76792524852269,-4.01642550844751));
#66146=CARTESIAN_POINT('Ctrl Pts',(-12.856820253537,6.36206504770304,-2.9874389816851));
#66147=CARTESIAN_POINT('Ctrl Pts',(-12.8237689602125,6.67412563574283,-1.87903278923947));
#66148=CARTESIAN_POINT('Ctrl Pts',(-12.790717666888,6.98618622378262,-0.77062659679384));
#66149=CARTESIAN_POINT('Ctrl Pts',(-12.7576663735636,7.01616760068184,0.417199261334988));
#66150=CARTESIAN_POINT('Ctrl Pts',(-12.7246150802391,6.7604220353384,1.53993860937376));
#66151=CARTESIAN_POINT('Ctrl Pts',(-12.6915637869146,6.50467646999496,2.66267795741254));
#66152=CARTESIAN_POINT('Ctrl Pts',(-12.6585124935901,5.96320396240885,3.72033079536126));
#66153=CARTESIAN_POINT('Ctrl Pts',(-12.6254612002656,5.2018761213938,4.58423347136944));
#66154=CARTESIAN_POINT('Ctrl Pts',(-12.5924099069412,4.44054828037874,5.44813614737763));
#66155=CARTESIAN_POINT('Ctrl Pts',(-12.5593586136167,3.45936510593474,6.11828866144528));
#66156=CARTESIAN_POINT('Ctrl Pts',(-12.5263073202922,2.37768969654824,6.51316422990427));
#66157=CARTESIAN_POINT('Ctrl Pts',(-12.4932560269677,1.29601428716175,6.90803979836326));
#66158=CARTESIAN_POINT('Ctrl Pts',(-12.4602047336432,0.113846642832758,
7.02763842121359));
#66159=CARTESIAN_POINT('Ctrl Pts',(-12.4271534403188,-1.02499973766536,
6.85741125425395));
#66160=CARTESIAN_POINT('Ctrl Pts',(-12.3941021469943,-2.16384611816347,
6.68718408729431));
#66161=CARTESIAN_POINT('Ctrl Pts',(-12.3610508536698,-3.25937123483072,
6.2271311305247));
#66162=CARTESIAN_POINT('Ctrl Pts',(-12.3279995603453,-4.17830194280872,
5.53321858179927));
#66163=CARTESIAN_POINT('Ctrl Pts',(-12.2949482670209,-5.09723265078673,
4.83930603307384));
#66164=CARTESIAN_POINT('Ctrl Pts',(-12.2618969736964,-5.8395689500755,3.91153389239259));
#66165=CARTESIAN_POINT('Ctrl Pts',(-12.2288456803719,-6.31500388982293,
2.86276795740906));
#66166=CARTESIAN_POINT('Ctrl Pts',(-12.2006210081167,-6.72100904130986,
1.96715777669006));
#66167=CARTESIAN_POINT('Ctrl Pts',(-12.1723963358615,-6.93237437728127,
0.983311965242192));
#66168=CARTESIAN_POINT('Ctrl Pts',(-12.1441716636063,-6.93330133372241,
-0.00014816709062256));
#66169=CARTESIAN_POINT('Origin',(-3.775,0.,0.));
#66170=CARTESIAN_POINT('',(-10.7148283363937,-6.93246113187516,7.73909840809384E-5));
#66171=CARTESIAN_POINT('',(-10.8941716636063,-6.93242320179691,4.17880428927411E-5));
#66172=CARTESIAN_POINT('',(-3.775,-6.933,-8.4904762584886E-16));
#66173=CARTESIAN_POINT('Ctrl Pts',(-10.7148283363937,-6.93246113187516,
7.73909840809384E-5));
#66174=CARTESIAN_POINT('Ctrl Pts',(-10.7288874627661,-6.93265361386657,
0.490124109213171));
#66175=CARTESIAN_POINT('Ctrl Pts',(-10.7429465891384,-6.88142264742765,
0.980131164451067));
#66176=CARTESIAN_POINT('Ctrl Pts',(-10.7570057155107,-6.77835452257098,
1.45898073080005));
#66177=CARTESIAN_POINT('Ctrl Pts',(-10.7900570088352,-6.53605391748161,
2.58469772462808));
#66178=CARTESIAN_POINT('Ctrl Pts',(-10.8231083021597,-6.00726861161217,
3.64875142588059));
#66179=CARTESIAN_POINT('Ctrl Pts',(-10.8561595954841,-5.25632656572988,
4.52169723012369));
#66180=CARTESIAN_POINT('Ctrl Pts',(-10.8892108888086,-4.50538451984759,
5.3946430343668));
#66181=CARTESIAN_POINT('Ctrl Pts',(-10.9222621821331,-3.53228573395244,
6.07648094160049));
#66182=CARTESIAN_POINT('Ctrl Pts',(-10.9553134754576,-2.45540993574669,
6.48426378657882));
#66183=CARTESIAN_POINT('Ctrl Pts',(-10.9883647687821,-1.37853413754095,
6.89204663155715));
#66184=CARTESIAN_POINT('Ctrl Pts',(-11.0214160621065,-0.197881327024614,
7.02577441428012));
#66185=CARTESIAN_POINT('Ctrl Pts',(-11.054467355431,0.942919338880705,6.86917883934291));
#66186=CARTESIAN_POINT('Ctrl Pts',(-11.0875186487555,2.08372000478602,6.7125832644057));
#66187=CARTESIAN_POINT('Ctrl Pts',(-11.12056994208,3.18466852608032,6.2656643318083));
#66188=CARTESIAN_POINT('Ctrl Pts',(-11.1536212354045,4.1118319577694,5.58279076784725));
#66189=CARTESIAN_POINT('Ctrl Pts',(-11.1866725287289,5.03899538945848,4.89991720388618));
#66190=CARTESIAN_POINT('Ctrl Pts',(-11.2197238220534,5.79237373154235,3.98108900856145));
#66191=CARTESIAN_POINT('Ctrl Pts',(-11.2527751153779,6.28031675869468,2.93808376615998));
#66192=CARTESIAN_POINT('Ctrl Pts',(-11.2858264087024,6.76825978584702,1.89507852375851));
#66193=CARTESIAN_POINT('Ctrl Pts',(-11.3188777020268,6.99076749806784,0.727896234280309));
#66194=CARTESIAN_POINT('Ctrl Pts',(-11.3519289953513,6.9207713153042,-0.421472665512276));
#66195=CARTESIAN_POINT('Ctrl Pts',(-11.3849802886758,6.85077513254057,-1.57084156530486));
#66196=CARTESIAN_POINT('Ctrl Pts',(-11.4180315820003,6.48827505479248,-2.70239707541183));
#66197=CARTESIAN_POINT('Ctrl Pts',(-11.4510828753248,5.87737005856666,-3.67848283958341));
#66198=CARTESIAN_POINT('Ctrl Pts',(-11.4841341686492,5.26646506234084,-4.65456860375499));
#66199=CARTESIAN_POINT('Ctrl Pts',(-11.5171854619737,4.40715514763729,-5.47518462199118));
#66200=CARTESIAN_POINT('Ctrl Pts',(-11.5502367552982,3.40397736165498,-6.04050104941805));
#66201=CARTESIAN_POINT('Ctrl Pts',(-11.5832880486227,2.40079957567267,-6.60581747684491));
#66202=CARTESIAN_POINT('Ctrl Pts',(-11.6163393419471,1.25375391841161,-6.91583431346245));
#66203=CARTESIAN_POINT('Ctrl Pts',(-11.6493906352716,0.102381158542403,
-6.93283729107388));
#66204=CARTESIAN_POINT('Ctrl Pts',(-11.6824419285961,-1.0489916013268,-6.94984026868531));
#66205=CARTESIAN_POINT('Ctrl Pts',(-11.7154932219206,-2.20469146380415,
-6.67382938729065));
#66206=CARTESIAN_POINT('Ctrl Pts',(-11.7485445152451,-3.22412485607506,
-6.13838201153716));
#66207=CARTESIAN_POINT('Ctrl Pts',(-11.7815958085695,-4.24355824834597,
-5.60293463578368));
#66208=CARTESIAN_POINT('Ctrl Pts',(-11.814647101894,-5.12672517041044,-4.80805076567137));
#66209=CARTESIAN_POINT('Ctrl Pts',(-11.8476983952185,-5.76618631467301,
-3.85042987084347));
#66210=CARTESIAN_POINT('Ctrl Pts',(-11.880749688543,-6.40564745893558,-2.89280897601557));
#66211=CARTESIAN_POINT('Ctrl Pts',(-11.9138009818675,-6.80140282539625,
-1.77245105647208));
#66212=CARTESIAN_POINT('Ctrl Pts',(-11.9468522751919,-6.90530785448801,
-0.625650254777943));
#66213=CARTESIAN_POINT('Ctrl Pts',(-11.9528442955925,-6.9241452732822,-0.417741483048112));
#66214=CARTESIAN_POINT('Ctrl Pts',(-11.9588363159931,-6.93339023533471,
-0.20896359392941));
#66215=CARTESIAN_POINT('Ctrl Pts',(-11.9648283363937,-6.93317898118896,
-0.000167065473373196));
#66216=CARTESIAN_POINT('Ctrl Pts',(-12.1441716636063,-6.93330133372241,
-0.00014816709062256));
#66217=CARTESIAN_POINT('Ctrl Pts',(-12.139345042537,-6.93345984991167,-0.168326892164513));
#66218=CARTESIAN_POINT('Ctrl Pts',(-12.1345184214677,-6.92746442206593,
-0.336494338650843));
#66219=CARTESIAN_POINT('Ctrl Pts',(-12.1296918003985,-6.91523604410695,
-0.504207325629335));
#66220=CARTESIAN_POINT('Ctrl Pts',(-12.096640507074,-6.83149967843746,-1.6526569443984));
#66221=CARTESIAN_POINT('Ctrl Pts',(-12.0635892137495,-6.45549336689239,
-2.77979645265072));
#66222=CARTESIAN_POINT('Ctrl Pts',(-12.030537920425,-5.83295914650944,-3.74850666788663));
#66223=CARTESIAN_POINT('Ctrl Pts',(-11.9974866271005,-5.2104249261265,-4.71721688312255));
#66224=CARTESIAN_POINT('Ctrl Pts',(-11.9644353337761,-4.3413627969057,-5.52749780534206));
#66225=CARTESIAN_POINT('Ctrl Pts',(-11.9313840404516,-3.3314961877589,-6.08077690042575));
#66226=CARTESIAN_POINT('Ctrl Pts',(-11.8983327471271,-2.32162957861211,
-6.63405599550944));
#66227=CARTESIAN_POINT('Ctrl Pts',(-11.8652814538026,-1.17095848953932,
-6.9303332634573));
#66228=CARTESIAN_POINT('Ctrl Pts',(-11.8322301604781,-0.0194647302894101,
-6.93356587491011));
#66229=CARTESIAN_POINT('Ctrl Pts',(-11.7991788671537,1.13202902896051,-6.93679848636293));
#66230=CARTESIAN_POINT('Ctrl Pts',(-11.7661275738292,2.28434545838755,-6.6469864413207));
#66231=CARTESIAN_POINT('Ctrl Pts',(-11.7330762805047,3.29730258707578,-6.09938605419939));
#66232=CARTESIAN_POINT('Ctrl Pts',(-11.7000249871802,4.310259715764,-5.55178566707809));
#66233=CARTESIAN_POINT('Ctrl Pts',(-11.6669736938558,5.18385754371339,-4.7463969378777));
#66234=CARTESIAN_POINT('Ctrl Pts',(-11.6339224005313,5.81182086618272,-3.7811972732666));
#66235=CARTESIAN_POINT('Ctrl Pts',(-11.6008711072068,6.43978418865204,-2.81599760865551));
#66236=CARTESIAN_POINT('Ctrl Pts',(-11.5678198138823,6.82211300564129,-1.69098700863372));
#66237=CARTESIAN_POINT('Ctrl Pts',(-11.5347685205578,6.91229612830372,-0.543025627548823));
#66238=CARTESIAN_POINT('Ctrl Pts',(-11.5017172272334,7.00247925096614,0.604935753536091));
#66239=CARTESIAN_POINT('Ctrl Pts',(-11.4686659339089,6.80051667930173,1.77584791568409));
#66240=CARTESIAN_POINT('Ctrl Pts',(-11.4356146405844,6.3309776293689,2.82726667529135));
#66241=CARTESIAN_POINT('Ctrl Pts',(-11.4025633472599,5.86143857943607,3.8786854348986));
#66242=CARTESIAN_POINT('Ctrl Pts',(-11.3695120539354,5.12432305123482,4.8106107919651));
#66243=CARTESIAN_POINT('Ctrl Pts',(-11.336460760611,4.20930286096558,5.50967186162471));
#66244=CARTESIAN_POINT('Ctrl Pts',(-11.3034094672865,3.29428267069634,6.20873293128433));
#66245=CARTESIAN_POINT('Ctrl Pts',(-11.270358173962,2.2013578183591,6.67492971353706));
#66246=CARTESIAN_POINT('Ctrl Pts',(-11.2373068806375,1.06348515100223,6.85154828711766));
#66247=CARTESIAN_POINT('Ctrl Pts',(-11.2042555873131,-0.0743875163546409,
7.02816686069827));
#66248=CARTESIAN_POINT('Ctrl Pts',(-11.1712042939886,-1.25720799873115,
6.91520722560674));
#66249=CARTESIAN_POINT('Ctrl Pts',(-11.1381530006641,-2.3410834368994,6.5264111837318));
#66250=CARTESIAN_POINT('Ctrl Pts',(-11.1051017073396,-3.42495887506765,
6.13761514185686));
#66251=CARTESIAN_POINT('Ctrl Pts',(-11.0720504140151,-4.40988926902763,
5.47298269319852));
#66252=CARTESIAN_POINT('Ctrl Pts',(-11.0389991206907,-5.17605554846697,
4.61336791905991));
#66253=CARTESIAN_POINT('Ctrl Pts',(-11.0059478273662,-5.94222182790631,
3.75375314492132));
#66254=CARTESIAN_POINT('Ctrl Pts',(-10.9728965340417,-6.489623992825,2.69915604530247));
#66255=CARTESIAN_POINT('Ctrl Pts',(-10.9398452407172,-6.75166929831051,
1.57787080705134));
#66256=CARTESIAN_POINT('Ctrl Pts',(-10.9246207150136,-6.87237608729205,
1.061369508198));
#66257=CARTESIAN_POINT('Ctrl Pts',(-10.9093961893099,-6.93253499603995,
0.530718118686483));
#66258=CARTESIAN_POINT('Ctrl Pts',(-10.8941716636063,-6.93242320179691,
4.17880428927411E-5));
#66259=CARTESIAN_POINT('Origin',(-3.775,0.,0.));
#66260=CARTESIAN_POINT('',(-9.46482833639373,-6.9335752955847,3.8715574435539E-5));
#66261=CARTESIAN_POINT('',(-9.64417166360628,-6.93351961894304,7.87873629847102E-5));
#66262=CARTESIAN_POINT('',(-3.775,-6.933,-8.4904762584886E-16));
#66263=CARTESIAN_POINT('Ctrl Pts',(-9.46482833639373,-6.9335752955847,3.8715574435539E-5));
#66264=CARTESIAN_POINT('Ctrl Pts',(-9.46588731621449,-6.93358665184356,
0.0369335697061642));
#66265=CARTESIAN_POINT('Ctrl Pts',(-9.46694629603526,-6.93329830646238,
0.0738282457414585));
#66266=CARTESIAN_POINT('Ctrl Pts',(-9.46800527585603,-6.9327091605576,0.11071811787296));
#66267=CARTESIAN_POINT('Ctrl Pts',(-9.50105656918051,-6.91432162027785,
1.26206959843057));
#66268=CARTESIAN_POINT('Ctrl Pts',(-9.534107862505,-6.60292563630512,2.40874161780564));
#66269=CARTESIAN_POINT('Ctrl Pts',(-9.56715915582948,-6.03640325342724,
3.41123886125227));
#66270=CARTESIAN_POINT('Ctrl Pts',(-9.60021044915396,-5.46988087054935,
4.4137361046989));
#66271=CARTESIAN_POINT('Ctrl Pts',(-9.63326174247843,-4.6482320887663,5.27205857221708));
#66272=CARTESIAN_POINT('Ctrl Pts',(-9.66631303580291,-3.67141239097886,
5.88178934184756));
#66273=CARTESIAN_POINT('Ctrl Pts',(-9.69936432912738,-2.69459269319141,
6.49152011147804));
#66274=CARTESIAN_POINT('Ctrl Pts',(-9.73241562245186,-1.56260207939957,
6.85265918322081));
#66275=CARTESIAN_POINT('Ctrl Pts',(-9.76546691577634,-0.413149837256818,
6.9212731501133));
#66276=CARTESIAN_POINT('Ctrl Pts',(-9.79851820910082,0.736302404885922,
6.98988711700579));
#66277=CARTESIAN_POINT('Ctrl Pts',(-9.8315695024253,1.90321627537957,6.76597597904801));
#66278=CARTESIAN_POINT('Ctrl Pts',(-9.86462079574978,2.94563399127012,6.27677904629267));
#66279=CARTESIAN_POINT('Ctrl Pts',(-9.89767208907426,3.98805170716067,5.78758211353733));
#66280=CARTESIAN_POINT('Ctrl Pts',(-9.93072338239874,4.90597326844813,5.03309938598441));
#66281=CARTESIAN_POINT('Ctrl Pts',(-9.96377467572322,5.58773138497425,4.1051154400185));
#66282=CARTESIAN_POINT('Ctrl Pts',(-9.99682596904769,6.26948950150039,3.17713149405257));
#66283=CARTESIAN_POINT('Ctrl Pts',(-10.0298772623722,6.71508417326519,2.07564632967368));
#66284=CARTESIAN_POINT('Ctrl Pts',(-10.0629285556967,6.87030777338264,0.934658175753425));
#66285=CARTESIAN_POINT('Ctrl Pts',(-10.0959798490211,7.02553137350009,-0.206329978166798));
#66286=CARTESIAN_POINT('Ctrl Pts',(-10.1290311423456,6.89038390197017,-1.38682112162837));
#66287=CARTESIAN_POINT('Ctrl Pts',(-10.1620824356701,6.48130636263677,-2.46320576488217));
#66288=CARTESIAN_POINT('Ctrl Pts',(-10.1951337289946,6.07222882330335,-3.53959040813599));
#66289=CARTESIAN_POINT('Ctrl Pts',(-10.228185022319,5.38922121616644,-4.51186855118207));
#66290=CARTESIAN_POINT('Ctrl Pts',(-10.2612363156435,4.51537300318336,-5.26176029942713));
#66291=CARTESIAN_POINT('Ctrl Pts',(-10.294287608968,3.64152479020029,-6.01165204767217));
#66292=CARTESIAN_POINT('Ctrl Pts',(-10.3273389022925,2.57683597137107,-6.53915740111618));
#66293=CARTESIAN_POINT('Ctrl Pts',(-10.360390195617,1.45082841465755,-6.78010410817761));
#66294=CARTESIAN_POINT('Ctrl Pts',(-10.3934414889414,0.32482085794402,-7.02105081523904));
#66295=CARTESIAN_POINT('Ctrl Pts',(-10.4264927822659,-0.862505436653806,
-6.9754388759179));
#66296=CARTESIAN_POINT('Ctrl Pts',(-10.4595440755904,-1.9667094673739,-6.64881708858398));
#66297=CARTESIAN_POINT('Ctrl Pts',(-10.4925953689149,-3.070913498094,-6.32219530125007));
#66298=CARTESIAN_POINT('Ctrl Pts',(-10.5256466622394,-4.09199526493636,
-5.71456366590338));
#66299=CARTESIAN_POINT('Ctrl Pts',(-10.5586979555638,-4.90573779910758,
-4.89984198244309));
#66300=CARTESIAN_POINT('Ctrl Pts',(-10.5917492488883,-5.7194803332788,-4.0851202989828));
#66301=CARTESIAN_POINT('Ctrl Pts',(-10.6248005422128,-6.32588363477888,
-3.0633085674089));
#66302=CARTESIAN_POINT('Ctrl Pts',(-10.6578518355373,-6.65117733337426,
-1.95871255842018));
#66303=CARTESIAN_POINT('Ctrl Pts',(-10.6768440024894,-6.83809988952223,
-1.32398182000576));
#66304=CARTESIAN_POINT('Ctrl Pts',(-10.6958361694416,-6.9322011121542,-0.661916024572997));
#66305=CARTESIAN_POINT('Ctrl Pts',(-10.7148283363937,-6.93246113187516,
7.73909840809384E-5));
#66306=CARTESIAN_POINT('Ctrl Pts',(-10.8941716636063,-6.93242320179691,
4.17880428927411E-5));
#66307=CARTESIAN_POINT('Ctrl Pts',(-10.8763448959854,-6.93229229919733,
-0.621340041014074));
#66308=CARTESIAN_POINT('Ctrl Pts',(-10.8585181283646,-6.8495264177626,-1.24275606595426));
#66309=CARTESIAN_POINT('Ctrl Pts',(-10.8406913607438,-6.68457054115384,
-1.8415296027582));
#66310=CARTESIAN_POINT('Ctrl Pts',(-10.8076400674193,-6.37873803245931,
-2.95167139743321));
#66311=CARTESIAN_POINT('Ctrl Pts',(-10.7745887740948,-5.79038456901791,
-3.98398160989983));
#66312=CARTESIAN_POINT('Ctrl Pts',(-10.7415374807704,-4.99108471633639,
-4.81287730488004));
#66313=CARTESIAN_POINT('Ctrl Pts',(-10.7084861874459,-4.19178486365487,
-5.64177299986026));
#66314=CARTESIAN_POINT('Ctrl Pts',(-10.6754348941214,-3.18153862173323,
-6.26725417735407));
#66315=CARTESIAN_POINT('Ctrl Pts',(-10.6423836007969,-2.08324479258817,
-6.61322959919343));
#66316=CARTESIAN_POINT('Ctrl Pts',(-10.6093323074724,-0.984950963443121,
-6.9592050210328));
#66317=CARTESIAN_POINT('Ctrl Pts',(-10.576281014148,0.201390452925348,-7.02567468721771));
#66318=CARTESIAN_POINT('Ctrl Pts',(-10.5432297208235,1.33145826747934,-6.80455240845744));
#66319=CARTESIAN_POINT('Ctrl Pts',(-10.510178427499,2.46152608203333,-6.58343012969718));
#66320=CARTESIAN_POINT('Ctrl Pts',(-10.4771271341745,3.53532029477285,-6.07471590599172));
#66321=CARTESIAN_POINT('Ctrl Pts',(-10.44407584085,4.42221134541617,-5.34029600433914));
#66322=CARTESIAN_POINT('Ctrl Pts',(-10.4110245475256,5.30910239605948,-4.60587610268656));
#66323=CARTESIAN_POINT('Ctrl Pts',(-10.3779732542011,6.0090902846066,-3.64575052308685));
#66324=CARTESIAN_POINT('Ctrl Pts',(-10.3449219608766,6.4370198584233,-2.57672077256163));
#66325=CARTESIAN_POINT('Ctrl Pts',(-10.3118706675521,6.86494943223999,-1.50769102203641));
#66326=CARTESIAN_POINT('Ctrl Pts',(-10.2788193742277,7.02082069132626,-0.329757100585688));
#66327=CARTESIAN_POINT('Ctrl Pts',(-10.2457680809032,6.88567153494304,0.813782594039565));
#66328=CARTESIAN_POINT('Ctrl Pts',(-10.2127167875787,6.75052237855983,1.95732228866483));
#66329=CARTESIAN_POINT('Ctrl Pts',(-10.1796654942542,6.32435280670714,3.0664677564646));
#66330=CARTESIAN_POINT('Ctrl Pts',(-10.1466142009297,5.65900733774437,4.0062888748619));
#66331=CARTESIAN_POINT('Ctrl Pts',(-10.1135629076053,4.99366186878161,4.9461099932592));
#66332=CARTESIAN_POINT('Ctrl Pts',(-10.0805116142808,4.08914050270877,5.71660676225401));
#66333=CARTESIAN_POINT('Ctrl Pts',(-10.0474603209563,3.05548036480908,6.22404646012164));
#66334=CARTESIAN_POINT('Ctrl Pts',(-10.0144090276318,2.0218202269094,6.73148615798928));
#66335=CARTESIAN_POINT('Ctrl Pts',(-9.98135773430734,0.859021317182861,
6.97586878472975));
#66336=CARTESIAN_POINT('Ctrl Pts',(-9.94830644098286,-0.291459175952402,
6.92746462612693));
#66337=CARTESIAN_POINT('Ctrl Pts',(-9.91525514765838,-1.44193966908766,
6.87906046752411));
#66338=CARTESIAN_POINT('Ctrl Pts',(-9.8822038543339,-2.58010174563166,6.537869523578));
#66339=CARTESIAN_POINT('Ctrl Pts',(-9.84915256100942,-3.56748534515149,
5.94539846516749));
#66340=CARTESIAN_POINT('Ctrl Pts',(-9.81610126768494,-4.55486894467133,
5.35292740675699));
#66341=CARTESIAN_POINT('Ctrl Pts',(-9.78304997436047,-5.39147406716701,
4.5091762338821));
#66342=CARTESIAN_POINT('Ctrl Pts',(-9.74999868103599,-5.97552575614819,
3.51678923666124));
#66343=CARTESIAN_POINT('Ctrl Pts',(-9.71694738771152,-6.55957744512937,
2.52440223944039));
#66344=CARTESIAN_POINT('Ctrl Pts',(-9.68389609438704,-6.89107570059605,
1.38337941787357));
#66345=CARTESIAN_POINT('Ctrl Pts',(-9.65084480106256,-6.9296929897379,0.232528848670892));
#66346=CARTESIAN_POINT('Ctrl Pts',(-9.64862042191046,-6.93229196497418,
0.155075661342478));
#66347=CARTESIAN_POINT('Ctrl Pts',(-9.64639604275837,-6.93356436504135,
0.0775779602098864));
#66348=CARTESIAN_POINT('Ctrl Pts',(-9.64417166360628,-6.93351961894304,
7.87873629847102E-5));
#66349=CARTESIAN_POINT('Origin',(-3.775,0.,0.));
#66350=CARTESIAN_POINT('',(-8.21482833639373,-6.93258532737551,-0.000132552009395881));
#66351=CARTESIAN_POINT('',(-8.39417166360628,-6.93268012709199,-0.00015517830160834));
#66352=CARTESIAN_POINT('',(-3.775,-6.933,-8.4904762584886E-16));
#66353=CARTESIAN_POINT('Ctrl Pts',(-8.21482833639373,-6.93258532737551,
-0.000132552009395881));
#66354=CARTESIAN_POINT('Ctrl Pts',(-8.23593846298743,-6.93207868762057,
0.735646992959097));
#66355=CARTESIAN_POINT('Ctrl Pts',(-8.25704858958112,-6.81542918802548,
1.47158339831407));
#66356=CARTESIAN_POINT('Ctrl Pts',(-8.27815871617481,-6.58523850360685,
2.17010337475394));
#66357=CARTESIAN_POINT('Ctrl Pts',(-8.31121000949928,-6.22483802009874,
3.26374857540489));
#66358=CARTESIAN_POINT('Ctrl Pts',(-8.34426130282376,-5.58611481446254,
4.26567514229184));
#66359=CARTESIAN_POINT('Ctrl Pts',(-8.37731259614824,-4.74677104834537,
5.0539963811913));
#66360=CARTESIAN_POINT('Ctrl Pts',(-8.41036388947272,-3.90742728222822,
5.84231762009076));
#66361=CARTESIAN_POINT('Ctrl Pts',(-8.44341518279719,-2.86746295563012,
6.41703353100273));
#66362=CARTESIAN_POINT('Ctrl Pts',(-8.47646647612167,-1.75339214460081,
6.70822858836495));
#66363=CARTESIAN_POINT('Ctrl Pts',(-8.50951776944615,-0.639321333571469,
6.99942364572718));
#66364=CARTESIAN_POINT('Ctrl Pts',(-8.54256906277064,0.548855961889083,
7.00709784953965));
#66365=CARTESIAN_POINT('Ctrl Pts',(-8.57562035609511,1.66659521378707,6.73031761508226));
#66366=CARTESIAN_POINT('Ctrl Pts',(-8.60867164941959,2.78433446568503,6.45353738062489));
#66367=CARTESIAN_POINT('Ctrl Pts',(-8.64172294274407,3.83163567402044,5.89230270789768));
#66368=CARTESIAN_POINT('Ctrl Pts',(-8.67477423606855,4.68109221403745,5.11488909852233));
#66369=CARTESIAN_POINT('Ctrl Pts',(-8.70782552939302,5.53054875405448,4.33747548914697));
#66370=CARTESIAN_POINT('Ctrl Pts',(-8.7408768227175,6.18216062575312,3.34388294312347));
#66371=CARTESIAN_POINT('Ctrl Pts',(-8.77392811604198,6.55665773132082,2.25498430167829));
#66372=CARTESIAN_POINT('Ctrl Pts',(-8.80697940936646,6.93115483688851,1.16608566023314));
#66373=CARTESIAN_POINT('Ctrl Pts',(-8.84003070269094,7.02853717632526,-0.018119076633696));
#66374=CARTESIAN_POINT('Ctrl Pts',(-8.87308199601542,6.83695796183047,-1.15356865190917));
#66375=CARTESIAN_POINT('Ctrl Pts',(-8.9061332893399,6.64537874733568,-2.28901822718469));
#66376=CARTESIAN_POINT('Ctrl Pts',(-8.93918458266438,6.16483797890932,-3.37571264086885));
#66377=CARTESIAN_POINT('Ctrl Pts',(-8.97223587598886,5.45379455727212,-4.28145299326918));
#66378=CARTESIAN_POINT('Ctrl Pts',(-9.00528716931333,4.74275113563496,-5.18719334566947));
#66379=CARTESIAN_POINT('Ctrl Pts',(-9.03833846263781,3.80120506078698,-5.91197963678595));
#66380=CARTESIAN_POINT('Ctrl Pts',(-9.07138975596229,2.7436975998381,-6.36763993070802));
#66381=CARTESIAN_POINT('Ctrl Pts',(-9.10444104928677,1.68619013888922,-6.82330022463009));
#66382=CARTESIAN_POINT('Ctrl Pts',(-9.13749234261125,0.512721291839444,
-7.00983452135775));
#66383=CARTESIAN_POINT('Ctrl Pts',(-9.17054363593573,-0.6339537302327,-6.90455049039608));
#66384=CARTESIAN_POINT('Ctrl Pts',(-9.20359492926021,-1.78062875230486,
-6.79926645943441));
#66385=CARTESIAN_POINT('Ctrl Pts',(-9.23664622258468,-2.90050994939938,
-6.40216410078339));
#66386=CARTESIAN_POINT('Ctrl Pts',(-9.26969751590916,-3.85736117253282,
-5.76155183879664));
#66387=CARTESIAN_POINT('Ctrl Pts',(-9.30274880923364,-4.81421239566625,
-5.12093957680988));
#66388=CARTESIAN_POINT('Ctrl Pts',(-9.33580010255813,-5.60803364483859,
-4.23681741148739));
#66389=CARTESIAN_POINT('Ctrl Pts',(-9.3688513958826,-6.14225472113137,-3.21674085795608));
#66390=CARTESIAN_POINT('Ctrl Pts',(-9.40084370938631,-6.65935908934048,
-2.22934806282485));
#66391=CARTESIAN_POINT('Ctrl Pts',(-9.43283602289002,-6.93323221728751,
-1.11457340158659));
#66392=CARTESIAN_POINT('Ctrl Pts',(-9.46482833639373,-6.9335752955847,3.8715574435539E-5));
#66393=CARTESIAN_POINT('Ctrl Pts',(-9.64417166360628,-6.93351961894304,
7.87873629847102E-5));
#66394=CARTESIAN_POINT('Ctrl Pts',(-9.61334474943389,-6.93289949798433,
-1.07395589217263));
#66395=CARTESIAN_POINT('Ctrl Pts',(-9.5825178352615,-6.67930505166503,-2.14827323277089));
#66396=CARTESIAN_POINT('Ctrl Pts',(-9.55169092108911,-6.19783372514389,
-3.10830688847735));
#66397=CARTESIAN_POINT('Ctrl Pts',(-9.51863962776464,-5.68162084859103,
-4.13761373958437));
#66398=CARTESIAN_POINT('Ctrl Pts',(-9.48558833444016,-4.9034587726683,-5.03554912495985));
#66399=CARTESIAN_POINT('Ctrl Pts',(-9.45253704111568,-3.95801272149387,
-5.69287711917089));
#66400=CARTESIAN_POINT('Ctrl Pts',(-9.4194857477912,-3.01256667031946,-6.35020511338191));
#66401=CARTESIAN_POINT('Ctrl Pts',(-9.38643445446672,-1.89983664389337,
-6.76692571642851));
#66402=CARTESIAN_POINT('Ctrl Pts',(-9.35338316114224,-0.755188834675868,
-6.8923438989554));
#66403=CARTESIAN_POINT('Ctrl Pts',(-9.32033186781776,0.389458974541642,
-7.01776208148228));
#66404=CARTESIAN_POINT('Ctrl Pts',(-9.28728057449329,1.56602456655058,-6.85187784348945));
#66405=CARTESIAN_POINT('Ctrl Pts',(-9.25422928116881,2.6313760040547,-6.41487138785898));
#66406=CARTESIAN_POINT('Ctrl Pts',(-9.22117798784433,3.69672744155883,-5.97786493222852));
#66407=CARTESIAN_POINT('Ctrl Pts',(-9.18812669451985,4.65086472455815,-5.26973625896042));
#66408=CARTESIAN_POINT('Ctrl Pts',(-9.15507540119538,5.3777148362232,-4.37663086606029));
#66409=CARTESIAN_POINT('Ctrl Pts',(-9.1220241078709,6.10456494788824,-3.48352547316016));
#66410=CARTESIAN_POINT('Ctrl Pts',(-9.08897281454642,6.60412788821901,-2.405443360628));
#66411=CARTESIAN_POINT('Ctrl Pts',(-9.05592152122194,6.81563066509628,-1.27353572171572));
#66412=CARTESIAN_POINT('Ctrl Pts',(-9.02287022789746,7.02713344197355,-0.141628082803403));
#66413=CARTESIAN_POINT('Ctrl Pts',(-8.98981893457298,6.95057605539729,1.04410508248903));
#66414=CARTESIAN_POINT('Ctrl Pts',(-8.9567676412485,6.59527188927863,2.13941658028022));
#66415=CARTESIAN_POINT('Ctrl Pts',(-8.92371634792402,6.23996772315997,3.23472807807139));
#66416=CARTESIAN_POINT('Ctrl Pts',(-8.89066505459954,5.60591677749891,4.2396179083613));
#66417=CARTESIAN_POINT('Ctrl Pts',(-8.85761376127506,4.77025282266349,5.03183888905018));
#66418=CARTESIAN_POINT('Ctrl Pts',(-8.82456246795059,3.93458886782808,5.82405986973906));
#66419=CARTESIAN_POINT('Ctrl Pts',(-8.79151117462611,2.89731190381832,6.4036120008269));
#66420=CARTESIAN_POINT('Ctrl Pts',(-8.75845988130163,1.78460908278264,6.69999141933305));
#66421=CARTESIAN_POINT('Ctrl Pts',(-8.72540858797715,0.671906261746978,
6.99637083783919));
#66422=CARTESIAN_POINT('Ctrl Pts',(-8.69235729465267,-0.516222416314614,
7.00957754376366));
#66423=CARTESIAN_POINT('Ctrl Pts',(-8.65930600132819,-1.63523833782786,
6.73800491065306));
#66424=CARTESIAN_POINT('Ctrl Pts',(-8.62625470800371,-2.75425425934114,
6.46643227754245));
#66425=CARTESIAN_POINT('Ctrl Pts',(-8.59320341467923,-3.80415742430608,
5.91008030539675));
#66426=CARTESIAN_POINT('Ctrl Pts',(-8.56015212135476,-4.65722467389882,
5.13663050396997));
#66427=CARTESIAN_POINT('Ctrl Pts',(-8.52710082803028,-5.51029192349154,
4.36318070254321));
#66428=CARTESIAN_POINT('Ctrl Pts',(-8.4940495347058,-6.16652325771206,3.37263307183539));
#66429=CARTESIAN_POINT('Ctrl Pts',(-8.46099824138132,-6.54608661040156,
2.28549003205181));
#66430=CARTESIAN_POINT('Ctrl Pts',(-8.43872271545631,-6.80190030035354,
1.55279002152113));
#66431=CARTESIAN_POINT('Ctrl Pts',(-8.41644718953129,-6.93204216650887,
0.776213154833276));
#66432=CARTESIAN_POINT('Ctrl Pts',(-8.39417166360628,-6.93268012709199,
-0.00015517830160834));
#66433=CARTESIAN_POINT('Origin',(-3.775,0.,0.));
#66434=CARTESIAN_POINT('',(-6.96482833639374,-6.93294662844253,0.000179318065722245));
#66435=CARTESIAN_POINT('',(-7.14417166360628,-6.93282359318651,0.000173910073648998));
#66436=CARTESIAN_POINT('',(-3.775,-6.933,-8.4904762584886E-16));
#66437=CARTESIAN_POINT('Ctrl Pts',(-6.96482833639374,-6.93294662844253,
0.000179318065722245));
#66438=CARTESIAN_POINT('Ctrl Pts',(-6.97293831643587,-6.93323237473856,
0.282805046459917));
#66439=CARTESIAN_POINT('Ctrl Pts',(-6.981048296478,-6.91627613789149,0.565396712104997));
#66440=CARTESIAN_POINT('Ctrl Pts',(-6.98915827652014,-6.88180763536459,
0.845835963022602));
#66441=CARTESIAN_POINT('Ctrl Pts',(-7.02220956984461,-6.74133520737417,
1.98873395951844));
#66442=CARTESIAN_POINT('Ctrl Pts',(-7.05526086316909,-6.31000567023157,
3.09588300514889));
#66443=CARTESIAN_POINT('Ctrl Pts',(-7.08831215649357,-5.64029126405976,
4.03259584673145));
#66444=CARTESIAN_POINT('Ctrl Pts',(-7.12136344981805,-4.97057685788794,
4.96930868831402));
#66445=CARTESIAN_POINT('Ctrl Pts',(-7.15441474314253,-4.06247758268689,
5.73558532584869));
#66446=CARTESIAN_POINT('Ctrl Pts',(-7.18746603646701,-3.02646582469637,
6.23820642640571));
#66447=CARTESIAN_POINT('Ctrl Pts',(-7.22051732979149,-1.99045406670588,
6.74082752696272));
#66448=CARTESIAN_POINT('Ctrl Pts',(-7.25356862311596,-0.826529825925916,
6.97979309054209));
#66449=CARTESIAN_POINT('Ctrl Pts',(-7.28661991644044,0.323712810088738,
6.92603240124453));
#66450=CARTESIAN_POINT('Ctrl Pts',(-7.31967120976492,1.47395544610341,6.87227171194696));
#66451=CARTESIAN_POINT('Ctrl Pts',(-7.3527225030894,2.61051647735277,6.52578476977245));
#66452=CARTESIAN_POINT('Ctrl Pts',(-7.38577379641388,3.59513061428307,5.92872251608635));
#66453=CARTESIAN_POINT('Ctrl Pts',(-7.41882508973836,4.57974475121336,5.33166026240026));
#66454=CARTESIAN_POINT('Ctrl Pts',(-7.45187638306283,5.4124119938246,4.48402269720259));
#66455=CARTESIAN_POINT('Ctrl Pts',(-7.48492767638731,5.99183643786163,3.48892689926549));
#66456=CARTESIAN_POINT('Ctrl Pts',(-7.51797896971179,6.57126088189867,2.49383110132837));
#66457=CARTESIAN_POINT('Ctrl Pts',(-7.55103026303627,6.89744252736151,1.3512770706518));
#66458=CARTESIAN_POINT('Ctrl Pts',(-7.58408155636075,6.93070061939663,0.200259159090933));
#66459=CARTESIAN_POINT('Ctrl Pts',(-7.61713284968523,6.96395871143175,-0.950758752469911));
#66460=CARTESIAN_POINT('Ctrl Pts',(-7.6501841430097,6.70429325003918,-2.11024054491504));
#66461=CARTESIAN_POINT('Ctrl Pts',(-7.68323543633418,6.18329314177072,-3.13713256484896));
#66462=CARTESIAN_POINT('Ctrl Pts',(-7.71628672965866,5.66229303350226,-4.16402458478286));
#66463=CARTESIAN_POINT('Ctrl Pts',(-7.74933802298314,4.8799582783579,-5.05832683220554));
#66464=CARTESIAN_POINT('Ctrl Pts',(-7.78238931630762,3.9314617165758,-5.7112453613554));
#66465=CARTESIAN_POINT('Ctrl Pts',(-7.81544060963211,2.98296515479368,-6.36416389050527));
#66466=CARTESIAN_POINT('Ctrl Pts',(-7.84849190295658,1.8683067863738,-6.77569870138231));
#66467=CARTESIAN_POINT('Ctrl Pts',(-7.88154319628106,0.723087391059321,
-6.89578562829469));
#66468=CARTESIAN_POINT('Ctrl Pts',(-7.91459448960554,-0.422132004255161,
-7.01587255520707));
#66469=CARTESIAN_POINT('Ctrl Pts',(-7.94764578293001,-1.59791242646425,
-6.84451159815479));
#66470=CARTESIAN_POINT('Ctrl Pts',(-7.98069707625449,-2.66121745600175,
-6.40254921561531));
#66471=CARTESIAN_POINT('Ctrl Pts',(-8.01374836957897,-3.72452248553925,
-5.96058683307582));
#66472=CARTESIAN_POINT('Ctrl Pts',(-8.04679966290345,-4.67535212240517,
-5.24802302504913));
#66473=CARTESIAN_POINT('Ctrl Pts',(-8.07985095622793,-5.39803573260544,
-4.35154283398653));
#66474=CARTESIAN_POINT('Ctrl Pts',(-8.11290224955241,-6.1207193428057,-3.45506264292393));
#66475=CARTESIAN_POINT('Ctrl Pts',(-8.14595354287689,-6.61525692634032,
-2.37466606882542));
#66476=CARTESIAN_POINT('Ctrl Pts',(-8.17900483620136,-6.82148683741763,
-1.24178586456869));
#66477=CARTESIAN_POINT('Ctrl Pts',(-8.19094600293215,-6.89599604735606,
-0.832485348784596));
#66478=CARTESIAN_POINT('Ctrl Pts',(-8.20288716966294,-6.93287191351981,
-0.416334045855466));
#66479=CARTESIAN_POINT('Ctrl Pts',(-8.21482833639373,-6.93258532737551,
-0.000132552009395881));
#66480=CARTESIAN_POINT('Ctrl Pts',(-8.39417166360628,-6.93268012709199,
-0.00015517830160834));
#66481=CARTESIAN_POINT('Ctrl Pts',(-8.38339589620681,-6.93298874000092,
-0.37572272280464));
#66482=CARTESIAN_POINT('Ctrl Pts',(-8.37262012880735,-6.90299172060379,
-0.751241467689222));
#66483=CARTESIAN_POINT('Ctrl Pts',(-8.36184436140789,-6.8422552629613,-1.12172078253239));
#66484=CARTESIAN_POINT('Ctrl Pts',(-8.32879306808341,-6.65596519167306,
-2.25805010847369));
#66485=CARTESIAN_POINT('Ctrl Pts',(-8.29574177475893,-6.1804896779381,-3.34697031149697));
#66486=CARTESIAN_POINT('Ctrl Pts',(-8.26269048143445,-5.47367142247792,
-4.25601171946639));
#66487=CARTESIAN_POINT('Ctrl Pts',(-8.22963918810997,-4.76685316701774,
-5.16505312743582));
#66488=CARTESIAN_POINT('Ctrl Pts',(-8.19658789478549,-3.82869216983234,
-5.89421574035139));
#66489=CARTESIAN_POINT('Ctrl Pts',(-8.16353660146101,-2.77331789547083,
-6.35479523258995));
#66490=CARTESIAN_POINT('Ctrl Pts',(-8.13048530813654,-1.71794362110932,
-6.81537472482851));
#66491=CARTESIAN_POINT('Ctrl Pts',(-8.09743401481205,-0.545356069571706,
-7.00737109639006));
#66492=CARTESIAN_POINT('Ctrl Pts',(-8.06438272148757,0.601796759709674,
-6.90742754268835));
#66493=CARTESIAN_POINT('Ctrl Pts',(-8.03133142816309,1.74894958899105,-6.80748398898665));
#66494=CARTESIAN_POINT('Ctrl Pts',(-7.99828013483862,2.87066769601621,-6.41560051002169));
#66495=CARTESIAN_POINT('Ctrl Pts',(-7.96522884151414,3.83049146744168,-5.7794506413104));
#66496=CARTESIAN_POINT('Ctrl Pts',(-7.93217754818967,4.79031523886716,-5.14330077259911));
#66497=CARTESIAN_POINT('Ctrl Pts',(-7.89912625486518,5.58824467469295,-4.26288451414151));
#66498=CARTESIAN_POINT('Ctrl Pts',(-7.8660749615407,6.12720980555135,-3.24530654888596));
#66499=CARTESIAN_POINT('Ctrl Pts',(-7.83302366821622,6.66617493640975,-2.22772858363043));
#66500=CARTESIAN_POINT('Ctrl Pts',(-7.79997237489175,6.94617576230075,-1.07298891157697));
#66501=CARTESIAN_POINT('Ctrl Pts',(-7.76692108156727,6.93314953234458,0.0784357038399208));
#66502=CARTESIAN_POINT('Ctrl Pts',(-7.73386978824279,6.92012330238841,1.22986031925681));
#66503=CARTESIAN_POINT('Ctrl Pts',(-7.7008184949183,6.61407001658507,2.37796987803714));
#66504=CARTESIAN_POINT('Ctrl Pts',(-7.66776720159383,6.05222176807958,3.38309418542708));
#66505=CARTESIAN_POINT('Ctrl Pts',(-7.63471590826935,5.49037351957408,4.38821849281703));
#66506=CARTESIAN_POINT('Ctrl Pts',(-7.60166461494488,4.67273030836643,5.25035754881659));
#66507=CARTESIAN_POINT('Ctrl Pts',(-7.5686133216204,3.69876033039241,5.86463013461226));
#66508=CARTESIAN_POINT('Ctrl Pts',(-7.53556202829592,2.72479035241839,6.47890272040792));
#66509=CARTESIAN_POINT('Ctrl Pts',(-7.50251073497143,1.594493607678,6.8453088359997));
#66510=CARTESIAN_POINT('Ctrl Pts',(-7.46945944164695,0.445373320719949,
6.91927432630602));
#66511=CARTESIAN_POINT('Ctrl Pts',(-7.43640814832247,-0.703746966238116,
6.99323981661234));
#66512=CARTESIAN_POINT('Ctrl Pts',(-7.403356854998,-1.87169079541385,6.77476468163321));
#66513=CARTESIAN_POINT('Ctrl Pts',(-7.37030556167353,-2.91637508698706,
6.29042692903177));
#66514=CARTESIAN_POINT('Ctrl Pts',(-7.33725426834905,-3.96105937856024,
5.80608917643034));
#66515=CARTESIAN_POINT('Ctrl Pts',(-7.30420297502456,-4.8824841325309,5.05588880620663));
#66516=CARTESIAN_POINT('Ctrl Pts',(-7.27115168170009,-5.56855588721342,
4.13108943602865));
#66517=CARTESIAN_POINT('Ctrl Pts',(-7.23810038837561,-6.25462764189595,
3.20629006585067));
#66518=CARTESIAN_POINT('Ctrl Pts',(-7.20504909505113,-6.70534639729033,
2.1068916957184));
#66519=CARTESIAN_POINT('Ctrl Pts',(-7.17199780172665,-6.86588116983432,
0.966638691136082));
#66520=CARTESIAN_POINT('Ctrl Pts',(-7.1627224223532,-6.91093298984508,0.646642765548731));
#66521=CARTESIAN_POINT('Ctrl Pts',(-7.15344704297974,-6.9331309329507,0.323429271653318));
#66522=CARTESIAN_POINT('Ctrl Pts',(-7.14417166360628,-6.93282359318651,
0.000173910073648998));
#66523=CARTESIAN_POINT('Origin',(-3.775,0.,0.));
#66524=CARTESIAN_POINT('',(-5.71482833639373,-6.9332949284688,-0.000149415166278977));
#66525=CARTESIAN_POINT('',(-5.89417166360628,-6.93340591766582,-0.000122946964495745));
#66526=CARTESIAN_POINT('',(-3.775,-6.933,-8.4904762584886E-16));
#66527=CARTESIAN_POINT('Ctrl Pts',(-5.71482833639373,-6.9332949284688,-0.000149415166278977));
#66528=CARTESIAN_POINT('Ctrl Pts',(-5.74298946320879,-6.9323649764916,0.981099183034019));
#66529=CARTESIAN_POINT('Ctrl Pts',(-5.77115059002384,-6.72197882763447,
1.96273382210663));
#66530=CARTESIAN_POINT('Ctrl Pts',(-5.7993117168389,-6.31774422827313,2.85671536429974));
#66531=CARTESIAN_POINT('Ctrl Pts',(-5.83236301016338,-5.84331447966477,
3.90593638346357));
#66532=CARTESIAN_POINT('Ctrl Pts',(-5.86541430348786,-5.10186755766788,
4.83441936161318));
#66533=CARTESIAN_POINT('Ctrl Pts',(-5.89846559681234,-4.18360220264049,
5.52921218769603));
#66534=CARTESIAN_POINT('Ctrl Pts',(-5.93151689013682,-3.26533684761313,
6.22400501377885));
#66535=CARTESIAN_POINT('Ctrl Pts',(-5.96456818346129,-2.17025305955524,
6.68510768779497));
#66536=CARTESIAN_POINT('Ctrl Pts',(-5.99761947678577,-1.03157032503942,
6.85642599836115));
#66537=CARTESIAN_POINT('Ctrl Pts',(-6.03067077011025,0.10711240947641,7.02774430892733));
#66538=CARTESIAN_POINT('Ctrl Pts',(-6.06372206343474,1.28939409045018,6.90927825604357));
#66539=CARTESIAN_POINT('Ctrl Pts',(-6.09677335675921,2.37144740508529,6.51543951022638));
#66540=CARTESIAN_POINT('Ctrl Pts',(-6.12982465008369,3.45350071972041,6.12160076440917));
#66541=CARTESIAN_POINT('Ctrl Pts',(-6.16287594340816,4.43532566801688,5.45238932565852));
#66542=CARTESIAN_POINT('Ctrl Pts',(-6.19592723673264,5.1974809643465,4.58921632000066));
#66543=CARTESIAN_POINT('Ctrl Pts',(-6.22897853005712,5.95963626067613,3.7260433143428));
#66544=CARTESIAN_POINT('Ctrl Pts',(-6.2620298233816,6.50212190503891,2.66890874177771));
#66545=CARTESIAN_POINT('Ctrl Pts',(-6.29508111670608,6.75894325866555,1.54641547866158));
#66546=CARTESIAN_POINT('Ctrl Pts',(-6.32813241003056,7.01576461229219,0.423922215545444));
#66547=CARTESIAN_POINT('Ctrl Pts',(-6.36118370335504,6.98692167518268,-0.763929738121745));
#66548=CARTESIAN_POINT('Ctrl Pts',(-6.39423499667951,6.67592325763527,-1.87263543293112));
#66549=CARTESIAN_POINT('Ctrl Pts',(-6.42728629000399,6.36492484008786,-2.9813411277405));
#66550=CARTESIAN_POINT('Ctrl Pts',(-6.46033758332848,5.77177094210252,-4.01090056369207));
#66551=CARTESIAN_POINT('Ctrl Pts',(-6.49338887665296,4.96862011319837,-4.8360654438526));
#66552=CARTESIAN_POINT('Ctrl Pts',(-6.52644016997744,4.16546928429424,-5.66123032401311));
#66553=CARTESIAN_POINT('Ctrl Pts',(-6.55949146330191,3.1523215244713,-6.28200064838259));
#66554=CARTESIAN_POINT('Ctrl Pts',(-6.59254275662639,2.05242861213926,-6.62285826502249));
#66555=CARTESIAN_POINT('Ctrl Pts',(-6.62559404995086,0.95253569980721,-6.9637158816624));
#66556=CARTESIAN_POINT('Ctrl Pts',(-6.65864534327534,-0.234102365033948,
-7.02466079057273));
#66557=CARTESIAN_POINT('Ctrl Pts',(-6.69169663659982,-1.36312830537076,
-6.79827890201643));
#66558=CARTESIAN_POINT('Ctrl Pts',(-6.7247479299243,-2.49215424570755,-6.57189701346013));
#66559=CARTESIAN_POINT('Ctrl Pts',(-6.75779922324879,-3.56356806153999,
-6.05818832743721));
#66560=CARTESIAN_POINT('Ctrl Pts',(-6.79085051657326,-4.44702977339938,
-5.31964669888933));
#66561=CARTESIAN_POINT('Ctrl Pts',(-6.82390180989774,-5.33049148525877,
-4.58110507034144));
#66562=CARTESIAN_POINT('Ctrl Pts',(-6.85695310322222,-6.02600109314511,
-3.61773049926859));
#66563=CARTESIAN_POINT('Ctrl Pts',(-6.89000439654669,-6.44894823766917,
-2.54671974005156));
#66564=CARTESIAN_POINT('Ctrl Pts',(-6.91494570982904,-6.76811448420257,
-1.73850885970419));
#66565=CARTESIAN_POINT('Ctrl Pts',(-6.93988702311139,-6.93206784848853,
-0.869003688169781));
#66566=CARTESIAN_POINT('Ctrl Pts',(-6.96482833639374,-6.93294662844253,
0.000179318065722245));
#66567=CARTESIAN_POINT('Ctrl Pts',(-7.14417166360628,-6.93282359318651,
0.000173910073648998));
#66568=CARTESIAN_POINT('Ctrl Pts',(-7.12039574965526,-6.93203577810175,
-0.828438198571558));
#66569=CARTESIAN_POINT('Ctrl Pts',(-7.09661983570424,-6.78337269219751,
-1.65732540685377));
#66570=CARTESIAN_POINT('Ctrl Pts',(-7.07284392175322,-6.4927056665093,-2.43299973809386));
#66571=CARTESIAN_POINT('Ctrl Pts',(-7.03979262842874,-6.08864460094668,
-3.51127752370906));
#66572=CARTESIAN_POINT('Ctrl Pts',(-7.00674133510426,-5.41017168012784,
-4.48672545590704));
#66573=CARTESIAN_POINT('Ctrl Pts',(-6.97369004177978,-4.53982471088598,
-5.24067802788111));
#66574=CARTESIAN_POINT('Ctrl Pts',(-6.9406387484553,-3.66947774164411,-5.99463059985517));
#66575=CARTESIAN_POINT('Ctrl Pts',(-6.90758745513082,-2.60725672397922,
-6.52708781160532));
#66576=CARTESIAN_POINT('Ctrl Pts',(-6.87453616180634,-1.48238331210909,
-6.77327500648447));
#66577=CARTESIAN_POINT('Ctrl Pts',(-6.84148486848186,-0.357509900238965,
-7.01946220136363));
#66578=CARTESIAN_POINT('Ctrl Pts',(-6.80843357515739,0.830015905836396,
-6.97937937937179));
#66579=CARTESIAN_POINT('Ctrl Pts',(-6.77538228183291,1.93572883332028,-6.65790270891211));
#66580=CARTESIAN_POINT('Ctrl Pts',(-6.74233098850843,3.04144176080416,-6.33642603845244));
#66581=CARTESIAN_POINT('Ctrl Pts',(-6.70927969518395,4.06534180969655,-5.73355551952493));
#66582=CARTESIAN_POINT('Ctrl Pts',(-6.67622840185947,4.8828691606461,-4.92263175115689));
#66583=CARTESIAN_POINT('Ctrl Pts',(-6.64317710853499,5.70039651159566,-4.11170798278886));
#66584=CARTESIAN_POINT('Ctrl Pts',(-6.61012581521051,6.31155116460237,-3.09273096498031));
#66585=CARTESIAN_POINT('Ctrl Pts',(-6.57707452188604,6.64198473648509,-1.98966161891559));
#66586=CARTESIAN_POINT('Ctrl Pts',(-6.54402322856156,6.97241830836781,-0.886592272850891));
#66587=CARTESIAN_POINT('Ctrl Pts',(-6.51097193523707,7.02213079912654,0.300569401470009));
#66588=CARTESIAN_POINT('Ctrl Pts',(-6.4779206419126,6.785074568784,1.42740242872407));
#66589=CARTESIAN_POINT('Ctrl Pts',(-6.44486934858812,6.54801833844146,2.55423545597816));
#66590=CARTESIAN_POINT('Ctrl Pts',(-6.41181805526364,6.02419338699765,3.62073983616544));
#66591=CARTESIAN_POINT('Ctrl Pts',(-6.37876676193916,5.27732423658162,4.49717283406753));
#66592=CARTESIAN_POINT('Ctrl Pts',(-6.34571546861469,4.53045508616559,5.37360583196962));
#66593=CARTESIAN_POINT('Ctrl Pts',(-6.31266417529021,3.56054173677734,6.05996744758651));
#66594=CARTESIAN_POINT('Ctrl Pts',(-6.27961288196573,2.48557640036856,6.47276019603829));
#66595=CARTESIAN_POINT('Ctrl Pts',(-6.24656158864125,1.41061106395978,6.88555294449007));
#66596=CARTESIAN_POINT('Ctrl Pts',(-6.21351029531677,0.230593740530481,
7.02477682577673));
#66597=CARTESIAN_POINT('Ctrl Pts',(-6.18045900199229,-0.91092372147787,
6.87349493133847));
#66598=CARTESIAN_POINT('Ctrl Pts',(-6.14740770866781,-2.05244118348622,
6.72221303690022));
#66599=CARTESIAN_POINT('Ctrl Pts',(-6.11435641534333,-3.15545878407361,
6.28042536673705));
#66600=CARTESIAN_POINT('Ctrl Pts',(-6.08130512201885,-4.08579186994391,
5.60187641714693));
#66601=CARTESIAN_POINT('Ctrl Pts',(-6.04825382869438,-5.0161249558142,4.92332746755682));
#66602=CARTESIAN_POINT('Ctrl Pts',(-6.0152025353699,-5.7737735269674,4.00801723853978));
#66603=CARTESIAN_POINT('Ctrl Pts',(-5.98215124204542,-6.26656787479109,
2.96729534561747));
#66604=CARTESIAN_POINT('Ctrl Pts',(-5.95282471589904,-6.70382599308494,
2.04385923362447));
#66605=CARTESIAN_POINT('Ctrl Pts',(-5.92349818975266,-6.93256242451305,
1.02168559205232));
#66606=CARTESIAN_POINT('Ctrl Pts',(-5.89417166360628,-6.93340591766582,
-0.000122946964495745));
#66607=CARTESIAN_POINT('Origin',(-3.775,0.,0.));
#66608=CARTESIAN_POINT('',(-4.46482833639373,-6.93242469144749,4.3789760074131E-5));
#66609=CARTESIAN_POINT('',(-4.64417166360628,-6.93240876118694,6.45577665183761E-6));
#66610=CARTESIAN_POINT('',(-3.775,-6.933,-8.4904762584886E-16));
#66611=CARTESIAN_POINT('Ctrl Pts',(-4.46482833639373,-6.93242469144749,
4.3789760074131E-5));
#66612=CARTESIAN_POINT('Ctrl Pts',(-4.47998931665723,-6.9325413820039,0.528504817274455));
#66613=CARTESIAN_POINT('Ctrl Pts',(-4.49515029692073,-6.87288824602125,
1.05693991976439));
#66614=CARTESIAN_POINT('Ctrl Pts',(-4.51031127718423,-6.75317819609387,
1.57140034946762));
#66615=CARTESIAN_POINT('Ctrl Pts',(-4.54336257050871,-6.49220747353687,
2.69293617831474));
#66616=CARTESIAN_POINT('Ctrl Pts',(-4.57641386383319,-5.94581611852691,
3.74805734008833));
#66617=CARTESIAN_POINT('Ctrl Pts',(-4.60946515715767,-5.18047390860605,
4.60840589453192));
#66618=CARTESIAN_POINT('Ctrl Pts',(-4.64251645048215,-4.41513169868519,
5.46875444897552));
#66619=CARTESIAN_POINT('Ctrl Pts',(-4.67556774380662,-3.43083863385344,
6.13433039608913));
#66620=CARTESIAN_POINT('Ctrl Pts',(-4.7086190371311,-2.34733625184864,6.524164875849));
#66621=CARTESIAN_POINT('Ctrl Pts',(-4.74167033045558,-1.26383386984384,
6.91399935560887));
#66622=CARTESIAN_POINT('Ctrl Pts',(-4.77472162378006,-0.0811221706659873,
7.028092368015));
#66623=CARTESIAN_POINT('Ctrl Pts',(-4.80777291710454,1.05691922017489,6.85256423308308));
#66624=CARTESIAN_POINT('Ctrl Pts',(-4.84082421042902,2.19496061101574,6.67703609815116));
#66625=CARTESIAN_POINT('Ctrl Pts',(-4.87387550375349,3.28833169351963,6.2118868158812));
#66626=CARTESIAN_POINT('Ctrl Pts',(-4.90692679707797,4.20402133572304,5.51370287695031));
#66627=CARTESIAN_POINT('Ctrl Pts',(-4.93997809040245,5.11971097792649,4.81551893801939));
#66628=CARTESIAN_POINT('Ctrl Pts',(-4.97302938372693,5.85771917982946,3.88430034242751));
#66629=CARTESIAN_POINT('Ctrl Pts',(-5.00608067705141,6.32826552936115,2.83333199544354));
#66630=CARTESIAN_POINT('Ctrl Pts',(-5.03913197037589,6.79881187889281,1.78236364845962));
#66631=CARTESIAN_POINT('Ctrl Pts',(-5.07218326370037,7.00189637605322,0.611645550083625));
#66632=CARTESIAN_POINT('Ctrl Pts',(-5.10523455702485,6.91281332002058,-0.536401723571765));
#66633=CARTESIAN_POINT('Ctrl Pts',(-5.13828585034933,6.82373026398793,-1.68444899722717));
#66634=CARTESIAN_POINT('Ctrl Pts',(-5.17133714367381,6.44247965476221,-2.80982544616197));
#66635=CARTESIAN_POINT('Ctrl Pts',(-5.20438843699828,5.81544151455764,-3.77562641124148));
#66636=CARTESIAN_POINT('Ctrl Pts',(-5.23743973032276,5.18840337435306,-4.74142737632099));
#66637=CARTESIAN_POINT('Ctrl Pts',(-5.27049102364724,4.31557770316962,-5.54765285754521));
#66638=CARTESIAN_POINT('Ctrl Pts',(-5.30354231697172,3.30314577138174,-6.09622365235295));
#66639=CARTESIAN_POINT('Ctrl Pts',(-5.3365936102962,2.29071383959387,-6.64479444716068));
#66640=CARTESIAN_POINT('Ctrl Pts',(-5.36964490362068,1.13867564720158,-6.93571055555193));
#66641=CARTESIAN_POINT('Ctrl Pts',(-5.40269619694516,-0.0128206836366791,
-6.9335813571758));
#66642=CARTESIAN_POINT('Ctrl Pts',(-5.43574749026964,-1.16431701447495,
-6.93145215879967));
#66643=CARTESIAN_POINT('Ctrl Pts',(-5.46879878359411,-2.31527148375918,
-6.63627765365614));
#66644=CARTESIAN_POINT('Ctrl Pts',(-5.50185007691859,-3.32566780676435,
-6.08396650595282));
#66645=CARTESIAN_POINT('Ctrl Pts',(-5.53490137024307,-4.33606412976952,
-5.5316553582495));
#66646=CARTESIAN_POINT('Ctrl Pts',(-5.56795266356755,-5.20590230649563,
-4.72220756798638));
#66647=CARTESIAN_POINT('Ctrl Pts',(-5.60100395689203,-5.8293645022086,-3.75409433910429));
#66648=CARTESIAN_POINT('Ctrl Pts',(-5.63405525021651,-6.45282669792157,
-2.78598111022221));
#66649=CARTESIAN_POINT('Ctrl Pts',(-5.66710654354098,-6.8299129126214,-1.65920244272117));
#66650=CARTESIAN_POINT('Ctrl Pts',(-5.70015783686546,-6.91474973236137,
-0.510833578881621));
#66651=CARTESIAN_POINT('Ctrl Pts',(-5.70504800337488,-6.92730192421013,
-0.34092449534652));
#66652=CARTESIAN_POINT('Ctrl Pts',(-5.70993816988431,-6.933456414195,-0.17054277562555));
#66653=CARTESIAN_POINT('Ctrl Pts',(-5.71482833639373,-6.9332949284688,-0.000149415166278977));
#66654=CARTESIAN_POINT('Ctrl Pts',(-5.89417166360628,-6.93340591766582,
-0.000122946964495745));
#66655=CARTESIAN_POINT('Ctrl Pts',(-5.89044689642818,-6.93351304987762,
-0.129903026931444));
#66656=CARTESIAN_POINT('Ctrl Pts',(-5.88672212925008,-6.92994390796523,
-0.259677217215776));
#66657=CARTESIAN_POINT('Ctrl Pts',(-5.88299736207198,-6.92265880264989,
-0.389242468881223));
#66658=CARTESIAN_POINT('Ctrl Pts',(-5.8499460687475,-6.85801525819082,-1.53892483363012));
#66659=CARTESIAN_POINT('Ctrl Pts',(-5.81689477542302,-6.50078804477848,
-2.67215600630032));
#66660=CARTESIAN_POINT('Ctrl Pts',(-5.78384348209855,-5.89443468272273,
-3.65107578236909));
#66661=CARTESIAN_POINT('Ctrl Pts',(-5.75079218877407,-5.288081320667,-4.62999555843786));
#66662=CARTESIAN_POINT('Ctrl Pts',(-5.71774089544959,-4.43260180996788,
-5.45460393790521));
#66663=CARTESIAN_POINT('Ctrl Pts',(-5.68468960212511,-3.43206722028373,
-6.02458539593727));
#66664=CARTESIAN_POINT('Ctrl Pts',(-5.65163830880063,-2.43153263059957,
-6.59456685396934));
#66665=CARTESIAN_POINT('Ctrl Pts',(-5.61858701547615,-1.28594296193037,
-6.90992139056613));
#66666=CARTESIAN_POINT('Ctrl Pts',(-5.58553572215167,-0.134661858544509,
-6.93228539381783));
#66667=CARTESIAN_POINT('Ctrl Pts',(-5.55248442882719,1.01661924484135,-6.95464939706954));
#66668=CARTESIAN_POINT('Ctrl Pts',(-5.51943313550271,2.17359178294388,-6.68402286697617));
#66669=CARTESIAN_POINT('Ctrl Pts',(-5.48638184217824,3.19550735898701,-6.1533281495583));
#66670=CARTESIAN_POINT('Ctrl Pts',(-5.45333054885376,4.21742293503015,-5.62263343214043));
#66671=CARTESIAN_POINT('Ctrl Pts',(-5.42027925552928,5.10428154901389,-4.83187052739805));
#66672=CARTESIAN_POINT('Ctrl Pts',(-5.3872279622048,5.74819479047523,-3.87723757954555));
#66673=CARTESIAN_POINT('Ctrl Pts',(-5.35417666888032,6.39210803193656,-2.92260463169304));
#66674=CARTESIAN_POINT('Ctrl Pts',(-5.32112537555584,6.79307590087549,-1.80410164073041));
#66675=CARTESIAN_POINT('Ctrl Pts',(-5.28807408223136,6.90231972463275,-0.657797093663752));
#66676=CARTESIAN_POINT('Ctrl Pts',(-5.25502278890689,7.01156354839,0.488507453402909));
#66677=CARTESIAN_POINT('Ctrl Pts',(-5.22197149558241,6.82908332696558,1.6626135565736));
#66678=CARTESIAN_POINT('Ctrl Pts',(-5.18892020225793,6.3770782031766,2.7216884810824));
#66679=CARTESIAN_POINT('Ctrl Pts',(-5.15586890893345,5.92507307938763,3.7807634055912));
#66680=CARTESIAN_POINT('Ctrl Pts',(-5.12281761560897,5.2035430532341,4.72480715143811));
#66681=CARTESIAN_POINT('Ctrl Pts',(-5.08976632228449,4.30026392842995,5.43897460403438));
#66682=CARTESIAN_POINT('Ctrl Pts',(-5.05671502896001,3.3969848036258,6.15314205663066));
#66683=CARTESIAN_POINT('Ctrl Pts',(-5.02366373563553,2.31195658017102,6.6374332159763));
#66684=CARTESIAN_POINT('Ctrl Pts',(-4.99061244231105,1.1771754618463,6.83293293758352));
#66685=CARTESIAN_POINT('Ctrl Pts',(-4.95756114898658,0.0423943435215721,
7.02843265919073));
#66686=CARTESIAN_POINT('Ctrl Pts',(-4.9245098556621,-1.1421396696731,6.93514094305953));
#66687=CARTESIAN_POINT('Ctrl Pts',(-4.89145856233762,-2.23232526349452,
6.56440694316333));
#66688=CARTESIAN_POINT('Ctrl Pts',(-4.85840726901314,-3.32251085731596,
6.19367294326712));
#66689=CARTESIAN_POINT('Ctrl Pts',(-4.82535597568866,-4.31834803176415,
5.54549665960591));
#66690=CARTESIAN_POINT('Ctrl Pts',(-4.79230468236418,-5.09869088135075,
4.69873024272701));
#66691=CARTESIAN_POINT('Ctrl Pts',(-4.7592533890397,-5.87903373093732,3.85196382584815));
#66692=CARTESIAN_POINT('Ctrl Pts',(-4.72620209571523,-6.44388225566231,
2.80660727575161));
#66693=CARTESIAN_POINT('Ctrl Pts',(-4.69315080239075,-6.72452132041392,
1.68983064500126));
#66694=CARTESIAN_POINT('Ctrl Pts',(-4.67682442279593,-6.86314887290602,
1.13817540363875));
#66695=CARTESIAN_POINT('Ctrl Pts',(-4.6604980432011,-6.93242723552036,0.569093139492368));
#66696=CARTESIAN_POINT('Ctrl Pts',(-4.64417166360628,-6.93240876118694,
6.45577665183761E-6));
#66697=CARTESIAN_POINT('Origin',(-3.775,0.,0.));
#66698=CARTESIAN_POINT('',(-3.21482833639373,-6.93352350063866,7.67097482256771E-5));
#66699=CARTESIAN_POINT('',(-3.39417166360628,-6.93343988028234,0.000112224652378165));
#66700=CARTESIAN_POINT('',(-3.775,-6.933,-8.4904762584886E-16));
#66701=CARTESIAN_POINT('Ctrl Pts',(-3.21482833639373,-6.93352350063866,
7.67097482256771E-5));
#66702=CARTESIAN_POINT('Ctrl Pts',(-3.21698917010567,-6.93356599650761,
0.0753617861455037));
#66703=CARTESIAN_POINT('Ctrl Pts',(-3.21915000381762,-6.93236527092446,
0.150645504658142));
#66704=CARTESIAN_POINT('Ctrl Pts',(-3.22131083752956,-6.92991264230934,
0.225888415961884));
#66705=CARTESIAN_POINT('Ctrl Pts',(-3.25436213085404,-6.89239816476019,
1.37677546402265));
#66706=CARTESIAN_POINT('Ctrl Pts',(-3.28741342417851,-6.56199343734975,
2.51811541993279));
#66707=CARTESIAN_POINT('Ctrl Pts',(-3.320464717503,-5.97889296266017,3.51106162685268));
#66708=CARTESIAN_POINT('Ctrl Pts',(-3.35351601082748,-5.3957924879706,4.50400783377254));
#66709=CARTESIAN_POINT('Ctrl Pts',(-3.38656730415196,-4.55999626600192,
5.34856029170215));
#66710=CARTESIAN_POINT('Ctrl Pts',(-3.41961859747644,-3.57318084861636,
5.94197723233487));
#66711=CARTESIAN_POINT('Ctrl Pts',(-3.45266989080091,-2.5863654312308,6.53539417296759));
#66712=CARTESIAN_POINT('Ctrl Pts',(-3.48572118412539,-1.44853081842837,
6.87767559630342));
#66713=CARTESIAN_POINT('Ctrl Pts',(-3.51877247744987,-0.298097233917136,
6.92718217211267));
#66714=CARTESIAN_POINT('Ctrl Pts',(-3.55182377077435,0.852336350594116,
6.97668874792192));
#66715=CARTESIAN_POINT('Ctrl Pts',(-3.58487506409883,2.01536890681417,6.73342047620457));
#66716=CARTESIAN_POINT('Ctrl Pts',(-3.61792635742331,3.04951482268625,6.22697150729964));
#66717=CARTESIAN_POINT('Ctrl Pts',(-3.65097765074779,4.08366073855829,5.72052253839471));
#66718=CARTESIAN_POINT('Ctrl Pts',(-3.68402894407227,4.98892001408236,4.95089287230221));
#66719=CARTESIAN_POINT('Ctrl Pts',(-3.71708023739674,5.65516575557641,4.01170974566463));
#66720=CARTESIAN_POINT('Ctrl Pts',(-3.75013153072122,6.32141149707046,3.07252661902703));
#66721=CARTESIAN_POINT('Ctrl Pts',(-3.7831828240457,6.74864370453449,1.96379003184436));
#66722=CARTESIAN_POINT('Ctrl Pts',(-3.81623411737018,6.88488858751857,0.820380365416631));
#66723=CARTESIAN_POINT('Ctrl Pts',(-3.84928541069466,7.02113347050265,-0.32302930101107));
#66724=CARTESIAN_POINT('Ctrl Pts',(-3.88233670401913,6.86639102900679,-1.50111204668383));
#66725=CARTESIAN_POINT('Ctrl Pts',(-3.91538799734361,6.4394860404881,-2.57055136903808));
#66726=CARTESIAN_POINT('Ctrl Pts',(-3.94843929066809,6.01258105196939,-3.63999069139237));
#66727=CARTESIAN_POINT('Ctrl Pts',(-3.98149058399257,5.31351351642781,-4.60078659042814));
#66728=CARTESIAN_POINT('Ctrl Pts',(-4.01454187731705,4.42732662341655,-5.33605601320785));
#66729=CARTESIAN_POINT('Ctrl Pts',(-4.04759317064153,3.54113973040531,-6.07132543598754));
#66730=CARTESIAN_POINT('Ctrl Pts',(-4.080644463966,2.4678334799244,-6.58106838251119));
#66731=CARTESIAN_POINT('Ctrl Pts',(-4.11369575729048,1.3379780705134,-6.80327343925921));
#66732=CARTESIAN_POINT('Ctrl Pts',(-4.14674705061496,0.208122661102384,
-7.02547849600723));
#66733=CARTESIAN_POINT('Ctrl Pts',(-4.17979834393945,-0.978281907238725,
-6.9601456629796));
#66734=CARTESIAN_POINT('Ctrl Pts',(-4.21284963726393,-2.07690676288808,
-6.61522283107489));
#66735=CARTESIAN_POINT('Ctrl Pts',(-4.2459009305884,-3.17553161853743,-6.27029999917018));
#66736=CARTESIAN_POINT('Ctrl Pts',(-4.27895222391288,-4.18637676149503,
-5.64578716838837));
#66737=CARTESIAN_POINT('Ctrl Pts',(-4.31200351723736,-4.98647053204155,
-4.81765777526651));
#66738=CARTESIAN_POINT('Ctrl Pts',(-4.34505481056184,-5.78656430258806,
-3.98952838214466));
#66739=CARTESIAN_POINT('Ctrl Pts',(-4.37810610388631,-6.37590670072351,
-2.95778242668277));
#66740=CARTESIAN_POINT('Ctrl Pts',(-4.41115739721079,-6.68280285473921,
-1.8479342009915));
#66741=CARTESIAN_POINT('Ctrl Pts',(-4.42904771027177,-6.84892247428479,
-1.24718517695605));
#66742=CARTESIAN_POINT('Ctrl Pts',(-4.44693802333275,-6.93228699384818,
-0.623552643876927));
#66743=CARTESIAN_POINT('Ctrl Pts',(-4.46482833639373,-6.93242469144749,
4.3789760074131E-5));
#66744=CARTESIAN_POINT('Ctrl Pts',(-4.64417166360628,-6.93240876118694,
6.45577665183761E-6));
#66745=CARTESIAN_POINT('Ctrl Pts',(-4.62744674987662,-6.93238983588688,
-0.5829718851691));
#66746=CARTESIAN_POINT('Ctrl Pts',(-4.61072183614696,-6.85964964898072,
-1.16595486408495));
#66747=CARTESIAN_POINT('Ctrl Pts',(-4.59399692241731,-6.71424448162094,
-1.73021259922285));
#66748=CARTESIAN_POINT('Ctrl Pts',(-4.56094562909283,-6.42689897329813,
-2.84528250129246));
#66749=CARTESIAN_POINT('Ctrl Pts',(-4.52789433576836,-5.85577835187427,
-3.88722559402747));
#66750=CARTESIAN_POINT('Ctrl Pts',(-4.49484304244388,-5.07036076759396,
-4.72928707988114));
#66751=CARTESIAN_POINT('Ctrl Pts',(-4.4617917491194,-4.28494318331366,-5.5713485657348));
#66752=CARTESIAN_POINT('Ctrl Pts',(-4.42874045579492,-3.28522863617693,
-6.21352844470713));
#66753=CARTESIAN_POINT('Ctrl Pts',(-4.39568916247044,-2.19283472306634,
-6.57770404281017));
#66754=CARTESIAN_POINT('Ctrl Pts',(-4.36263786914596,-1.10044080995574,
-6.94187964091322));
#66755=CARTESIAN_POINT('Ctrl Pts',(-4.32958657582149,0.0846324691287112,
-7.02805095814698));
#66756=CARTESIAN_POINT('Ctrl Pts',(-4.29653528249701,1.21821819699567,-6.82573505360377));
#66757=CARTESIAN_POINT('Ctrl Pts',(-4.26348398917253,2.35180392486264,-6.62341914906057));
#66758=CARTESIAN_POINT('Ctrl Pts',(-4.23043269584805,3.43390210151211,-6.1326160227404));
#66759=CARTESIAN_POINT('Ctrl Pts',(-4.19738140252357,4.33287297016345,-5.41303301504006));
#66760=CARTESIAN_POINT('Ctrl Pts',(-4.16433010919909,5.23184383881479,-4.69345000733972));
#66761=CARTESIAN_POINT('Ctrl Pts',(-4.13127881587461,5.947687399468,-3.74508711825922));
#66762=CARTESIAN_POINT('Ctrl Pts',(-4.09822752255013,6.39331962014627,-2.68331489619455));
#66763=CARTESIAN_POINT('Ctrl Pts',(-4.06517622922565,6.83895184082454,-1.62154267412987));
#66764=CARTESIAN_POINT('Ctrl Pts',(-4.03212493590118,7.01437272152787,-0.446361119081015));
#66765=CARTESIAN_POINT('Ctrl Pts',(-3.9990736425767,6.89824190463591,0.69926620296696));
#66766=CARTESIAN_POINT('Ctrl Pts',(-3.96602234925222,6.78211108774396,1.84489352501493));
#66767=CARTESIAN_POINT('Ctrl Pts',(-3.93297105592774,6.37442857325671,2.96096661406203));
#66768=CARTESIAN_POINT('Ctrl Pts',(-3.89991976260326,5.72478988606175,3.91171258631457));
#66769=CARTESIAN_POINT('Ctrl Pts',(-3.86686846927878,5.0751511988668,4.8624585585671));
#66770=CARTESIAN_POINT('Ctrl Pts',(-3.8338171759543,4.18355633896413,5.64787741402508));
#66771=CARTESIAN_POINT('Ctrl Pts',(-3.80076588262982,3.15846989213457,6.17242112448318));
#66772=CARTESIAN_POINT('Ctrl Pts',(-3.76771458930535,2.133383445305,6.69696483494128));
#66773=CARTESIAN_POINT('Ctrl Pts',(-3.73466329598087,0.974805411548551,
6.96063340039951));
#66774=CARTESIAN_POINT('Ctrl Pts',(-3.70161200265639,-0.17632050008306,
6.93135092739772));
#66775=CARTESIAN_POINT('Ctrl Pts',(-3.66856070933191,-1.32744641171467,
6.90206845439593));
#66776=CARTESIAN_POINT('Ctrl Pts',(-3.63550941600743,-2.4711202012214,6.57983494293414));
#66777=CARTESIAN_POINT('Ctrl Pts',(-3.60245812268295,-3.46821129548542,
6.00385084819352));
#66778=CARTESIAN_POINT('Ctrl Pts',(-3.56940682935847,-4.46530238974945,
5.42786675345291));
#66779=CARTESIAN_POINT('Ctrl Pts',(-3.53635553603399,-5.31581078877077,
4.59813207543344));
#66780=CARTESIAN_POINT('Ctrl Pts',(-3.50330424270951,-5.91627017017391,
3.61558596509572));
#66781=CARTESIAN_POINT('Ctrl Pts',(-3.47025294938503,-6.51672955157704,
2.633039854758));
#66782=CARTESIAN_POINT('Ctrl Pts',(-3.43720165606056,-6.86713991536202,
1.49768231210201));
#66783=CARTESIAN_POINT('Ctrl Pts',(-3.40415036273608,-6.92487302681091,
0.347632219498546));
#66784=CARTESIAN_POINT('Ctrl Pts',(-3.40082412969281,-6.93068320135103,
0.231892887246826));
#66785=CARTESIAN_POINT('Ctrl Pts',(-3.39749789664954,-6.9335291083434,0.116004747225949));
#66786=CARTESIAN_POINT('Ctrl Pts',(-3.39417166360628,-6.93343988028234,
0.000112224652378165));
#66787=CARTESIAN_POINT('Origin',(-3.775,0.,0.));
#66788=CARTESIAN_POINT('',(-1.96482833639373,-6.93267455605571,-0.000154115015024714));
#66789=CARTESIAN_POINT('',(-2.14417166360627,-6.93278353301175,-0.000170174852231984));
#66790=CARTESIAN_POINT('',(-3.775,-6.933,-8.4904762584886E-16));
#66791=CARTESIAN_POINT('Ctrl Pts',(-1.96482833639373,-6.93267455605571,
-0.000154115015024714));
#66792=CARTESIAN_POINT('Ctrl Pts',(-1.9870403168786,-6.93204351043128,0.774001260964231));
#66793=CARTESIAN_POINT('Ctrl Pts',(-2.00925229736346,-6.80265738467977,
1.5483623151292));
#66794=CARTESIAN_POINT('Ctrl Pts',(-2.03146427784833,-6.54827367295132,
2.27921624920437));
#66795=CARTESIAN_POINT('Ctrl Pts',(-2.06451557117281,-6.1697522403832,3.36672250597088));
#66796=CARTESIAN_POINT('Ctrl Pts',(-2.09756686449728,-5.51447039087689,
4.35789851282317));
#66797=CARTESIAN_POINT('Ctrl Pts',(-2.13061815782176,-4.66214468357019,
5.13216540613831));
#66798=CARTESIAN_POINT('Ctrl Pts',(-2.16366945114624,-3.8098189762635,5.90643229945344));
#66799=CARTESIAN_POINT('Ctrl Pts',(-2.19672074447072,-2.76044941115642,
6.46379007923142));
#66800=CARTESIAN_POINT('Ctrl Pts',(-2.2297720377952,-1.64169423341061,6.73643487688339));
#66801=CARTESIAN_POINT('Ctrl Pts',(-2.26282333111968,-0.522939055664844,
7.00907967453536));
#66802=CARTESIAN_POINT('Ctrl Pts',(-2.29587462444416,0.665201734719648,
6.99701149006133));
#66803=CARTESIAN_POINT('Ctrl Pts',(-2.32892591776863,1.77818805067639,6.7016984461356));
#66804=CARTESIAN_POINT('Ctrl Pts',(-2.36197721109311,2.89117436663317,6.40638540220986));
#66805=CARTESIAN_POINT('Ctrl Pts',(-2.39502850441759,3.92900620816221,5.8278274988324));
#66806=CARTESIAN_POINT('Ctrl Pts',(-2.42807979774207,4.76542892097592,5.03640764887344));
#66807=CARTESIAN_POINT('Ctrl Pts',(-2.46113109106655,5.60185163378963,4.24498779891447));
#66808=CARTESIAN_POINT('Ctrl Pts',(-2.49418238439103,6.23686521788803,3.24070600237399));
#66809=CARTESIAN_POINT('Ctrl Pts',(-2.52723367771551,6.59321879570106,2.14573547263377));
#66810=CARTESIAN_POINT('Ctrl Pts',(-2.56028497103999,6.9495723735141,1.05076494289354));
#66811=CARTESIAN_POINT('Ctrl Pts',(-2.59333626436446,7.02726594504176,-0.134894320046401));
#66812=CARTESIAN_POINT('Ctrl Pts',(-2.62638755768894,6.81684790683436,-1.26700411269759));
#66813=CARTESIAN_POINT('Ctrl Pts',(-2.65943885101342,6.60642986862698,-2.39911390534872));
#66814=CARTESIAN_POINT('Ctrl Pts',(-2.6924901443379,6.1079002206845,-3.47767422771116));
#66815=CARTESIAN_POINT('Ctrl Pts',(-2.72554143766238,5.38190625270701,-4.37147571119614));
#66816=CARTESIAN_POINT('Ctrl Pts',(-2.75859273098686,4.65591228472947,-5.26527719468117));
#66817=CARTESIAN_POINT('Ctrl Pts',(-2.79164402431133,3.70245399671694,-5.97431983928876));
#66818=CARTESIAN_POINT('Ctrl Pts',(-2.82469531763581,2.63752180418136,-6.41234696027691));
#66819=CARTESIAN_POINT('Ctrl Pts',(-2.85774661096029,1.57258961164582,-6.85037408126505));
#66820=CARTESIAN_POINT('Ctrl Pts',(-2.89079790428477,0.396183514587305,
-7.01738567863371));
#66821=CARTESIAN_POINT('Ctrl Pts',(-2.92384919760925,-0.74858395262916,
-6.89306440361402));
#66822=CARTESIAN_POINT('Ctrl Pts',(-2.95690049093373,-1.89335141984563,
-6.76874312859432));
#66823=CARTESIAN_POINT('Ctrl Pts',(-2.98995178425821,-3.00648025722006,
-6.35308898118627));
#66824=CARTESIAN_POINT('Ctrl Pts',(-3.02300307758269,-3.9525557560139,-5.69666725393945));
#66825=CARTESIAN_POINT('Ctrl Pts',(-3.05605437090717,-4.89863125480775,
-5.04024552669263));
#66826=CARTESIAN_POINT('Ctrl Pts',(-3.08910566423165,-5.67765341502102,
-4.14305621960703));
#66827=CARTESIAN_POINT('Ctrl Pts',(-3.12215695755613,-6.1948523812837,-3.11424449595857));
#66828=CARTESIAN_POINT('Ctrl Pts',(-3.15304741716866,-6.67823781561858,
-2.15269461994424));
#66829=CARTESIAN_POINT('Ctrl Pts',(-3.1839378767812,-6.93291599580554,-1.07617020320189));
#66830=CARTESIAN_POINT('Ctrl Pts',(-3.21482833639373,-6.93352350063866,
7.67097482256771E-5));
#66831=CARTESIAN_POINT('Ctrl Pts',(-3.39417166360628,-6.93343988028234,
0.000112224652378165));
#66832=CARTESIAN_POINT('Ctrl Pts',(-3.36444660332506,-6.93264248892117,
-1.03556752924019));
#66833=CARTESIAN_POINT('Ctrl Pts',(-3.33472154304385,-6.69743936418148,
-2.07159728252277));
#66834=CARTESIAN_POINT('Ctrl Pts',(-3.30499648276264,-6.24862210463677,
-3.004902060123));
#66835=CARTESIAN_POINT('Ctrl Pts',(-3.27194518943816,-5.74958221190098,
-4.04264360459012));
#66836=CARTESIAN_POINT('Ctrl Pts',(-3.23889389611369,-4.98644656731659,
-4.95338405097345));
#66837=CARTESIAN_POINT('Ctrl Pts',(-3.20584260278921,-4.05205239472479,
-5.62632970842377));
#66838=CARTESIAN_POINT('Ctrl Pts',(-3.17279130946473,-3.11765822213298,
-6.29927536587409));
#66839=CARTESIAN_POINT('Ctrl Pts',(-3.13974001614025,-2.01200552153376,
-6.7344262343914));
#66840=CARTESIAN_POINT('Ctrl Pts',(-3.10668872281577,-0.869599512260727,
-6.87884520001451));
#66841=CARTESIAN_POINT('Ctrl Pts',(-3.07363742949129,0.272806497012319,
-7.02326416563761));
#66842=CARTESIAN_POINT('Ctrl Pts',(-3.04058613616681,1.45196581495916,-6.8769512283665));
#66843=CARTESIAN_POINT('Ctrl Pts',(-3.00753484284234,2.52443097149833,-6.45770569688855));
#66844=CARTESIAN_POINT('Ctrl Pts',(-2.97448354951786,3.59689612803748,-6.03846016541059));
#66845=CARTESIAN_POINT('Ctrl Pts',(-2.94143225619338,4.56266712316898,-5.34628203972578));
#66846=CARTESIAN_POINT('Ctrl Pts',(-2.9083809628689,5.30425567195863,-4.46537639667492));
#66847=CARTESIAN_POINT('Ctrl Pts',(-2.87532966954442,6.04584422074829,-3.58447075362404));
#66848=CARTESIAN_POINT('Ctrl Pts',(-2.84227837621994,6.56325032319611,-2.51483759320713));
#66849=CARTESIAN_POINT('Ctrl Pts',(-2.80922708289546,6.79353032506368,-1.38660027402525));
#66850=CARTESIAN_POINT('Ctrl Pts',(-2.77617578957098,7.02381032693125,-0.258362954843403));
#66851=CARTESIAN_POINT('Ctrl Pts',(-2.7431244962465,6.96696422821857,0.928478523103413));
#66852=CARTESIAN_POINT('Ctrl Pts',(-2.71007320292203,6.62990748888108,2.02954213712485));
#66853=CARTESIAN_POINT('Ctrl Pts',(-2.67702190959755,6.29285074954358,3.13060575114631));
#66854=CARTESIAN_POINT('Ctrl Pts',(-2.64397061627307,5.67558336958127,4.14589150124242));
#66855=CARTESIAN_POINT('Ctrl Pts',(-2.61091932294859,4.8531973596086,4.95188751752045));
#66856=CARTESIAN_POINT('Ctrl Pts',(-2.57786802962411,4.03081134963592,5.7578835337985));
#66857=CARTESIAN_POINT('Ctrl Pts',(-2.54481673629963,3.00330670965288,6.35458981625845));
#66858=CARTESIAN_POINT('Ctrl Pts',(-2.51176544297515,1.89568176589007,6.66941565955809));
#66859=CARTESIAN_POINT('Ctrl Pts',(-2.47871414965067,0.788056822127327,
6.9842415028577));
#66860=CARTESIAN_POINT('Ctrl Pts',(-2.4456628563262,-0.399688425415167,
7.01718690699704));
#66861=CARTESIAN_POINT('Ctrl Pts',(-2.41261156300172,-1.52306200837649,
6.7642439870341));
#66862=CARTESIAN_POINT('Ctrl Pts',(-2.37956026967724,-2.64643559133784,
6.51130106707115));
#66863=CARTESIAN_POINT('Ctrl Pts',(-2.34650897635276,-3.70543750971801,
5.97246982300591));
#66864=CARTESIAN_POINT('Ctrl Pts',(-2.31345768302828,-4.57123772020481,
5.21330032732275));
#66865=CARTESIAN_POINT('Ctrl Pts',(-2.2804063897038,-5.4370379306916,4.45413083163958));
#66866=CARTESIAN_POINT('Ctrl Pts',(-2.24735509637932,-6.10963643328502,
3.47462308433849));
#66867=CARTESIAN_POINT('Ctrl Pts',(-2.21430380305484,-6.50721005777458,
2.39393647816395));
#66868=CARTESIAN_POINT('Ctrl Pts',(-2.19092642323865,-6.78841628874856,
1.62956030060298));
#66869=CARTESIAN_POINT('Ctrl Pts',(-2.16754904342246,-6.93203256432842,
0.814566176130428));
#66870=CARTESIAN_POINT('Ctrl Pts',(-2.14417166360627,-6.93278353301175,
-0.000170174852231984));
#66871=CARTESIAN_POINT('Origin',(-3.775,0.,0.));
#66872=CARTESIAN_POINT('',(-0.714828336393731,-6.93283010606057,0.00017441890636849));
#66873=CARTESIAN_POINT('',(-0.894171663606273,-6.9327161513647,0.000161366341133071));
#66874=CARTESIAN_POINT('',(-3.775,-6.933,-8.4904762584886E-16));
#66875=CARTESIAN_POINT('Ctrl Pts',(-0.714828336393731,-6.93283010606057,
0.00017441890636849));
#66876=CARTESIAN_POINT('Ctrl Pts',(-0.72404017032704,-6.93313670432102,
0.321214300938314));
#66877=CARTESIAN_POINT('Ctrl Pts',(-0.733252004260348,-6.91124292430801,
0.642212700743149));
#66878=CARTESIAN_POINT('Ctrl Pts',(-0.742463838193657,-6.86680430682767,
0.960059070181433));
#66879=CARTESIAN_POINT('Ctrl Pts',(-0.775515131518135,-6.70736224654842,
2.10046538498052));
#66880=CARTESIAN_POINT('Ctrl Pts',(-0.808566424842613,-6.25769718736783,
3.200295150628));
#66881=CARTESIAN_POINT('Ctrl Pts',(-0.841617718167092,-5.57251192825613,
4.12575152135315));
#66882=CARTESIAN_POINT('Ctrl Pts',(-0.874669011491571,-4.88732666914443,
5.05120789207829));
#66883=CARTESIAN_POINT('Ctrl Pts',(-0.90772030481605,-3.96662121010161,
5.8022908678811));
#66884=CARTESIAN_POINT('Ctrl Pts',(-0.940771598140529,-2.9224015089145,
6.28762946007467));
#66885=CARTESIAN_POINT('Ctrl Pts',(-0.973822891465008,-1.87818180772739,
6.77296805226824));
#66886=CARTESIAN_POINT('Ctrl Pts',(-1.00687418478949,-0.710447864395994,
6.99256226085256));
#66887=CARTESIAN_POINT('Ctrl Pts',(-1.03992547811396,0.438742774360017,
6.91969794026094));
#66888=CARTESIAN_POINT('Ctrl Pts',(-1.07297677143844,1.58793341311603,6.84683361966932));
#66889=CARTESIAN_POINT('Ctrl Pts',(-1.10602806476292,2.71858074729665,6.48151076990174));
#66890=CARTESIAN_POINT('Ctrl Pts',(-1.1390793580874,3.69313890233341,5.86817176423596));
#66891=CARTESIAN_POINT('Ctrl Pts',(-1.17213065141188,4.66769705737016,5.25483275857018));
#66892=CARTESIAN_POINT('Ctrl Pts',(-1.20518194473636,5.48616603326304,4.39347759700619));
#66893=CARTESIAN_POINT('Ctrl Pts',(-1.23823323806084,6.04897717788414,3.38889213577852));
#66894=CARTESIAN_POINT('Ctrl Pts',(-1.27128453138532,6.61178832250524,2.38430667455085));
#66895=CARTESIAN_POINT('Ctrl Pts',(-1.3043358247098,6.91894163585457,1.23649091365949));
#66896=CARTESIAN_POINT('Ctrl Pts',(-1.33738711803427,6.93307120388089,0.0850793066626232));
#66897=CARTESIAN_POINT('Ctrl Pts',(-1.37043841135875,6.94720077190721,-1.06633230033425));
#66898=CARTESIAN_POINT('Ctrl Pts',(-1.40348970468323,6.66830659461054,-2.22133975343664));
#66899=CARTESIAN_POINT('Ctrl Pts',(-1.43654099800771,6.13031679649852,-3.23943371302343));
#66900=CARTESIAN_POINT('Ctrl Pts',(-1.46959229133219,5.5923269983865,-4.25752767261022));
#66901=CARTESIAN_POINT('Ctrl Pts',(-1.50264358465667,4.79524157945913,-5.13870813868142));
#66902=CARTESIAN_POINT('Ctrl Pts',(-1.53569487798115,3.83602783246789,-5.77577746065725));
#66903=CARTESIAN_POINT('Ctrl Pts',(-1.56874617130562,2.87681408547664,-6.41284678263308));
#66904=CARTESIAN_POINT('Ctrl Pts',(-1.6017974646301,1.75547201042152,-6.80580496051356));
#66905=CARTESIAN_POINT('Ctrl Pts',(-1.63484875795458,0.608415475483342,
-6.90684771916227));
#66906=CARTESIAN_POINT('Ctrl Pts',(-1.66790005127906,-0.53864105945484,
-7.00789047781097));
#66907=CARTESIAN_POINT('Ctrl Pts',(-1.70095134460354,-1.71141205427608,
-6.81701781722792));
#66908=CARTESIAN_POINT('Ctrl Pts',(-1.73400263792802,-2.76722719324648,
-6.35744983994855));
#66909=CARTESIAN_POINT('Ctrl Pts',(-1.7670539312525,-3.82304233221688,-5.89788186266918));
#66910=CARTESIAN_POINT('Ctrl Pts',(-1.80010522457698,-4.76190161533643,
-5.1696185686935));
#66911=CARTESIAN_POINT('Ctrl Pts',(-1.83315651790145,-5.46959062995009,
-4.26125487940662));
#66912=CARTESIAN_POINT('Ctrl Pts',(-1.86620781122593,-6.17727964456378,
-3.35289119011972));
#66913=CARTESIAN_POINT('Ctrl Pts',(-1.89925910455042,-6.65379839067156,
-2.26442710552161));
#66914=CARTESIAN_POINT('Ctrl Pts',(-1.9323103978749,-6.84117725591047,-1.12827680988217));
#66915=CARTESIAN_POINT('Ctrl Pts',(-1.94314971071451,-6.90262895524085,
-0.755671466837037));
#66916=CARTESIAN_POINT('Ctrl Pts',(-1.95398902355412,-6.93298250252378,
-0.377937280835089));
#66917=CARTESIAN_POINT('Ctrl Pts',(-1.96482833639373,-6.93267455605571,
-0.000154115015024714));
#66918=CARTESIAN_POINT('Ctrl Pts',(-2.14417166360627,-6.93278353301175,
-0.000170174852231984));
#66919=CARTESIAN_POINT('Ctrl Pts',(-2.13449775009798,-6.93309429521638,
-0.337320405264556));
#66920=CARTESIAN_POINT('Ctrl Pts',(-2.12482383658969,-6.90894037892185,
-0.674426493780623));
#66921=CARTESIAN_POINT('Ctrl Pts',(-2.11514992308141,-6.8599479572671,-1.00788323781755));
#66922=CARTESIAN_POINT('Ctrl Pts',(-2.08209862975693,-6.69256348588433,
-2.14715088257655));
#66923=CARTESIAN_POINT('Ctrl Pts',(-2.04904733643245,-6.23524579673307,
-3.24382070704658));
#66924=CARTESIAN_POINT('Ctrl Pts',(-2.01599604310797,-5.54362864899564,
-4.16448027964133));
#66925=CARTESIAN_POINT('Ctrl Pts',(-1.98294474978349,-4.85201150125823,
-5.08513985223605));
#66926=CARTESIAN_POINT('Ctrl Pts',(-1.94989345645902,-3.92609489493467,
-5.82978917295552));
#66927=CARTESIAN_POINT('Ctrl Pts',(-1.91684216313454,-2.8785187359834,-6.30783992219835));
#66928=CARTESIAN_POINT('Ctrl Pts',(-1.88379086981006,-1.83094257703207,
-6.78589067144121));
#66929=CARTESIAN_POINT('Ctrl Pts',(-1.85073957648558,-0.661706865453005,
-6.9973428492074));
#66930=CARTESIAN_POINT('Ctrl Pts',(-1.8176882831611,0.48694815843834,-6.91647280689227));
#66931=CARTESIAN_POINT('Ctrl Pts',(-1.78463698983662,1.63560318232962,-6.83560276457714));
#66932=CARTESIAN_POINT('Ctrl Pts',(-1.75158569651214,2.76367751853319,-6.46241050218072));
#66933=CARTESIAN_POINT('Ctrl Pts',(-1.71853440318767,3.73393830366126,-5.84229572530679));
#66934=CARTESIAN_POINT('Ctrl Pts',(-1.68548310986319,4.70419908878935,-5.22218094843285));
#66935=CARTESIAN_POINT('Ctrl Pts',(-1.65243181653871,5.51664632284193,-4.35514365708138));
#66936=CARTESIAN_POINT('Ctrl Pts',(-1.61938052321423,6.07244391257379,-3.34666095177451));
#66937=CARTESIAN_POINT('Ctrl Pts',(-1.58632922988975,6.62824150230566,-2.33817824646763));
#66938=CARTESIAN_POINT('Ctrl Pts',(-1.55327793656527,6.92738944771679,-1.18825012720539));
#66939=CARTESIAN_POINT('Ctrl Pts',(-1.52022664324079,6.93349570636123,-0.0367680208484475));
#66940=CARTESIAN_POINT('Ctrl Pts',(-1.48717534991632,6.93960196500567,1.11471408550848));
#66941=CARTESIAN_POINT('Ctrl Pts',(-1.45412405659184,6.6526665368834,2.26775017896005));
#66942=CARTESIAN_POINT('Ctrl Pts',(-1.42107276326736,6.10759578334394,3.28207074036592));
#66943=CARTESIAN_POINT('Ctrl Pts',(-1.38802146994288,5.56252502980449,4.29639130177176));
#66944=CARTESIAN_POINT('Ctrl Pts',(-1.3549701766184,4.75931895084777,5.17199633113198));
#66945=CARTESIAN_POINT('Ctrl Pts',(-1.32191888329392,3.79568943173556,5.80236644269368));
#66946=CARTESIAN_POINT('Ctrl Pts',(-1.28886758996944,2.83205991262329,6.43273655425541));
#66947=CARTESIAN_POINT('Ctrl Pts',(-1.25581629664496,1.70800695335555,6.81787174801864));
#66948=CARTESIAN_POINT('Ctrl Pts',(-1.22276500332048,0.560274207474504,
6.9109194330368));
#66949=CARTESIAN_POINT('Ctrl Pts',(-1.18971370999601,-0.587458538406507,
7.00396711805494));
#66950=CARTESIAN_POINT('Ctrl Pts',(-1.15666241667153,-1.75887107090073,
6.80492729432799));
#66951=CARTESIAN_POINT('Ctrl Pts',(-1.12361112334705,-2.81145833437188,
6.33801361875924));
#66952=CARTESIAN_POINT('Ctrl Pts',(-1.09055983002257,-3.86404559784306,
5.87109994319048));
#66953=CARTESIAN_POINT('Ctrl Pts',(-1.05750853669809,-4.79780759229117,
5.13631241577991));
#66954=CARTESIAN_POINT('Ctrl Pts',(-1.02445724337361,-5.49915000206846,
4.22303964606504));
#66955=CARTESIAN_POINT('Ctrl Pts',(-0.99140595004913,-6.20049241184572,
3.30976687635023));
#66956=CARTESIAN_POINT('Ctrl Pts',(-0.958354656724652,-6.66941523695218,
2.21800886433114));
#66957=CARTESIAN_POINT('Ctrl Pts',(-0.925303363400175,-6.84887292645916,
1.08058050819984));
#66958=CARTESIAN_POINT('Ctrl Pts',(-0.914926130135541,-6.90521790173331,
0.723458042294939));
#66959=CARTESIAN_POINT('Ctrl Pts',(-0.904548896870907,-6.9330275729645,
0.361833420535273));
#66960=CARTESIAN_POINT('Ctrl Pts',(-0.894171663606273,-6.9327161513647,
0.000161366341133071));
#66961=CARTESIAN_POINT('Origin',(-3.775,0.,0.));
#66962=CARTESIAN_POINT('',(0.535171663606277,-6.9334003037143,-0.000124581990723627));
#66963=CARTESIAN_POINT('',(0.355828336393729,-6.93349343740785,-9.14711828918373E-5));
#66964=CARTESIAN_POINT('',(-3.775,-6.933,-8.4904762584886E-16));
#66965=CARTESIAN_POINT('Ctrl Pts',(0.535171663606277,-6.9334003037143,-0.000124581990723627));
#66966=CARTESIAN_POINT('Ctrl Pts',(0.505908682900044,-6.93255028157601,
1.01947227644454));
#66967=CARTESIAN_POINT('Ctrl Pts',(0.476645702193811,-6.7048358987811,2.03943623973099));
#66968=CARTESIAN_POINT('Ctrl Pts',(0.447382721487578,-6.26940839990456,
2.96128909796236));
#66969=CARTESIAN_POINT('Ctrl Pts',(0.414331428163099,-5.77761154122546,
4.00248273183317));
#66970=CARTESIAN_POINT('Ctrl Pts',(0.381280134838622,-5.02084040545093,
4.91851855368217));
#66971=CARTESIAN_POINT('Ctrl Pts',(0.348228841514143,-4.09115795914137,
5.5979586779342));
#66972=CARTESIAN_POINT('Ctrl Pts',(0.315177548189664,-3.16147551283182,
6.27739880218624));
#66973=CARTESIAN_POINT('Ctrl Pts',(0.282126254865185,-2.05888175598725,
6.72024322884129));
#66974=CARTESIAN_POINT('Ctrl Pts',(0.249074961540705,-0.917509780327954,
6.87261890471945));
#66975=CARTESIAN_POINT('Ctrl Pts',(0.216023668216227,0.223862195331312,
7.0249945805976));
#66976=CARTESIAN_POINT('Ctrl Pts',(0.182972374891749,1.40401238980529,6.88690150569888));
#66977=CARTESIAN_POINT('Ctrl Pts',(0.149921081567271,2.47937279058131,6.47513902335924));
#66978=CARTESIAN_POINT('Ctrl Pts',(0.116869788242791,3.55473319135739,6.06337654101958));
#66979=CARTESIAN_POINT('Ctrl Pts',(0.0838184949183126,4.52530379843548,
5.37794465123898));
#66980=CARTESIAN_POINT('Ctrl Pts',(0.0507672015938329,5.27301244293917,
4.50222773558971));
#66981=CARTESIAN_POINT('Ctrl Pts',(0.0177159082693552,6.02072108744283,
3.6265108199405));
#66982=CARTESIAN_POINT('Ctrl Pts',(-0.0153353850551226,6.54556776937211,
2.56050887842267));
#66983=CARTESIAN_POINT('Ctrl Pts',(-0.0483866783796008,6.78370367071106,
1.43390352342335));
#66984=CARTESIAN_POINT('Ctrl Pts',(-0.0814379717040799,7.02183957205002,
0.307298168423996));
#66985=CARTESIAN_POINT('Ctrl Pts',(-0.114489265028562,6.97326469279862,
-0.879910600056927));
#66986=CARTESIAN_POINT('Ctrl Pts',(-0.14754055835304,6.64388827985173,-1.98329607758234));
#66987=CARTESIAN_POINT('Ctrl Pts',(-0.180591851677519,6.31451186690483,
-3.08668155510775));
#66988=CARTESIAN_POINT('Ctrl Pts',(-0.213643145001997,5.70433392026246,
-4.10624374167772));
#66989=CARTESIAN_POINT('Ctrl Pts',(-0.246694438326475,4.88758400450776,
-4.91795052896881));
#66990=CARTESIAN_POINT('Ctrl Pts',(-0.279745731650954,4.07083408875305,
-5.72965731625989));
#66991=CARTESIAN_POINT('Ctrl Pts',(-0.312797024975433,3.04751220388602,
-6.33350870427208));
#66992=CARTESIAN_POINT('Ctrl Pts',(-0.345848318299913,1.94210783426131,
-6.65604476897545));
#66993=CARTESIAN_POINT('Ctrl Pts',(-0.378899611624392,0.836703464636607,
-6.97858083367883));
#66994=CARTESIAN_POINT('Ctrl Pts',(-0.411950904948871,-0.350783389745759,
-7.01980157507339));
#66995=CARTESIAN_POINT('Ctrl Pts',(-0.44500219827335,-1.47589219465302,
-6.77469239421739));
#66996=CARTESIAN_POINT('Ctrl Pts',(-0.47805349159783,-2.60100099956031,
-6.52958321336138));
#66997=CARTESIAN_POINT('Ctrl Pts',(-0.511104784922308,-3.66373175499246,
-5.99814411025479));
#66998=CARTESIAN_POINT('Ctrl Pts',(-0.544156078246788,-4.53480079594826,
-5.24502588626326));
#66999=CARTESIAN_POINT('Ctrl Pts',(-0.577207371571265,-5.40586983690397,
-4.49190766227179));
#67000=CARTESIAN_POINT('Ctrl Pts',(-0.610258664895742,-6.08527716338335,
-3.51711031739542));
#67001=CARTESIAN_POINT('Ctrl Pts',(-0.643309958220219,-6.49037129593408,
-2.43922021298191));
#67002=CARTESIAN_POINT('Ctrl Pts',(-0.66714941761139,-6.78256031945386,
-1.66175238078425));
#67003=CARTESIAN_POINT('Ctrl Pts',(-0.690988877002561,-6.93203665528496,
-0.830650071206651));
#67004=CARTESIAN_POINT('Ctrl Pts',(-0.714828336393731,-6.93283010606057,
0.00017441890636849));
#67005=CARTESIAN_POINT('Ctrl Pts',(-0.894171663606273,-6.9327161513647,
0.000161366341133071));
#67006=CARTESIAN_POINT('Ctrl Pts',(-0.871497603546429,-6.93203570100982,
-0.790085288970428));
#67007=CARTESIAN_POINT('Ctrl Pts',(-0.848823543486585,-6.79710113099127,
-1.58055839350899));
#67008=CARTESIAN_POINT('Ctrl Pts',(-0.826149483426741,-6.53223324953361,
-2.32478888744209));
#67009=CARTESIAN_POINT('Ctrl Pts',(-0.793098190102262,-6.14614332919358,
-3.40963122670925));
#67010=CARTESIAN_POINT('Ctrl Pts',(-0.760046896777782,-5.48397093460601,
-4.396217205));
#67011=CARTESIAN_POINT('Ctrl Pts',(-0.726995603453304,-4.62627087572379,
-5.16452634632805));
#67012=CARTESIAN_POINT('Ctrl Pts',(-0.693944310128825,-3.76857081684157,
-5.9328354876561));
#67013=CARTESIAN_POINT('Ctrl Pts',(-0.660893016804347,-2.7153430936647,
-6.48286779202144));
#67014=CARTESIAN_POINT('Ctrl Pts',(-0.627841723479869,-1.5947153052461,
-6.74771055193542));
#67015=CARTESIAN_POINT('Ctrl Pts',(-0.59479043015539,-0.474087516827503,
-7.01255331184939));
#67016=CARTESIAN_POINT('Ctrl Pts',(-0.561739136830911,0.713940336832824,
-6.992206527312));
#67017=CARTESIAN_POINT('Ctrl Pts',(-0.528687843506432,1.82484190768325,
-6.68914543192549));
#67018=CARTESIAN_POINT('Ctrl Pts',(-0.495636550181953,2.93574347853367,
-6.38608433653898));
#67019=CARTESIAN_POINT('Ctrl Pts',(-0.462585256857474,3.96951876657419,
-5.80030893030336));
#67020=CARTESIAN_POINT('Ctrl Pts',(-0.429533963532995,4.80040660667202,
-5.00308015207695));
#67021=CARTESIAN_POINT('Ctrl Pts',(-0.396482670208517,5.63129444676985,
-4.20585137385055));
#67022=CARTESIAN_POINT('Ctrl Pts',(-0.363431376884039,6.259294838925,-3.19716922363337));
#67023=CARTESIAN_POINT('Ctrl Pts',(-0.330380083559561,6.60801007665816,
-2.09974222805347));
#67024=CARTESIAN_POINT('Ctrl Pts',(-0.297328790235082,6.95672531439132,
-1.00231523247358));
#67025=CARTESIAN_POINT('Ctrl Pts',(-0.264277496910602,7.02615539770249,
0.183856608469029));
#67026=CARTESIAN_POINT('Ctrl Pts',(-0.231226203586123,6.80785399567866,
1.31447273498114));
#67027=CARTESIAN_POINT('Ctrl Pts',(-0.198174910261644,6.58955259365484,
2.44508886149324));
#67028=CARTESIAN_POINT('Ctrl Pts',(-0.165123616937165,6.08351970629602,
3.52014927357485));
#67029=CARTESIAN_POINT('Ctrl Pts',(-0.132072323612686,5.35131540980637,
4.40887037485291));
#67030=CARTESIAN_POINT('Ctrl Pts',(-0.0990210302882075,4.61911111331672,
5.29759147613098));
#67031=CARTESIAN_POINT('Ctrl Pts',(-0.0659697369637293,3.66073540769622,
5.9999732666055));
#67032=CARTESIAN_POINT('Ctrl Pts',(-0.0329184436392508,2.59277692373161,
6.43056936991209));
#67033=CARTESIAN_POINT('Ctrl Pts',(0.000132849685227725,1.524818439767,
6.86116547321868));
#67034=CARTESIAN_POINT('Ctrl Pts',(0.0331841430097067,0.347277177458266,
7.01997588935733));
#67035=CARTESIAN_POINT('Ctrl Pts',(0.0662354363341857,-0.796596233340036,
6.8876809623062));
#67036=CARTESIAN_POINT('Ctrl Pts',(0.0992867296586647,-1.94046964413834,
6.75538603525507));
#67037=CARTESIAN_POINT('Ctrl Pts',(0.132338022983144,-3.05067520342622,
6.33198576501416));
#67038=CARTESIAN_POINT('Ctrl Pts',(0.165389316307622,-3.99215382603479,
5.66898777796905));
#67039=CARTESIAN_POINT('Ctrl Pts',(0.198440609632101,-4.93363244864337,
5.00598979092394));
#67040=CARTESIAN_POINT('Ctrl Pts',(0.231491902956579,-5.70638413457265,
4.10339408707464));
#67041=CARTESIAN_POINT('Ctrl Pts',(0.264543196281057,-6.21640184621488,
3.07100353042177));
#67042=CARTESIAN_POINT('Ctrl Pts',(0.294971576318614,-6.68594512863285,
2.12054232163898));
#67043=CARTESIAN_POINT('Ctrl Pts',(0.325399956356172,-6.93280032536449,
1.06006957977906));
#67044=CARTESIAN_POINT('Ctrl Pts',(0.355828336393729,-6.93349343740785,
-9.14711828918373E-5));
#67045=CARTESIAN_POINT('Origin',(-3.775,0.,0.));
#67046=CARTESIAN_POINT('',(1.78517166360628,-6.93240903352825,8.51318353534136E-6));
#67047=CARTESIAN_POINT('',(1.60582833639373,-6.93241554159061,-2.91227924267906E-5));
#67048=CARTESIAN_POINT('',(-3.775,-6.933,-8.4904762584886E-16));
#67049=CARTESIAN_POINT('Ctrl Pts',(1.78517166360628,-6.93240903352825,8.51318353534136E-6));
#67050=CARTESIAN_POINT('Ctrl Pts',(1.7689088294516,-6.93243330175633,0.566880142059182));
#67051=CARTESIAN_POINT('Ctrl Pts',(1.75264599529692,-6.86369887729813,1.13374598789551));
#67052=CARTESIAN_POINT('Ctrl Pts',(1.73638316114225,-6.72613751527892,1.68338615060896));
#67053=CARTESIAN_POINT('Ctrl Pts',(1.70333186781777,-6.446568721613,2.8004311913427));
#67054=CARTESIAN_POINT('Ctrl Pts',(1.67028057449329,-5.88272216008265,3.84632852564582));
#67055=CARTESIAN_POINT('Ctrl Pts',(1.63722928116881,-5.10319107464959,4.69384231329956));
#67056=CARTESIAN_POINT('Ctrl Pts',(1.60417798784433,-4.32365998921648,5.54135610095335));
#67057=CARTESIAN_POINT('Ctrl Pts',(1.57112669451985,-3.32844437988063,6.19048634195776));
#67058=CARTESIAN_POINT('Ctrl Pts',(1.53807540119537,-2.23861453729065,6.56226483463869));
#67059=CARTESIAN_POINT('Ctrl Pts',(1.50502410787089,-1.14878469470068,6.93404332731963));
#67060=CARTESIAN_POINT('Ctrl Pts',(1.47197281454642,0.0356593811433296,
7.02847007167711));
#67061=CARTESIAN_POINT('Ctrl Pts',(1.43892152122194,1.17062731708598,6.83405783491746));
#67062=CARTESIAN_POINT('Ctrl Pts',(1.40587022789746,2.30559525302856,6.63964559815781));
#67063=CARTESIAN_POINT('Ctrl Pts',(1.37281893457298,3.39108704906978,6.156394380281));
#67064=CARTESIAN_POINT('Ctrl Pts',(1.3397676412485,4.29505010674682,5.44309281447954));
#67065=CARTESIAN_POINT('Ctrl Pts',(1.30671634792402,5.19901316442391,4.72979124867803));
#67066=CARTESIAN_POINT('Ctrl Pts',(1.27366505459954,5.92144748373691,3.7864393349518));
#67067=CARTESIAN_POINT('Ctrl Pts',(1.24061376127506,6.37446725160844,2.72779802490509));
#67068=CARTESIAN_POINT('Ctrl Pts',(1.20756246795058,6.82748701947995,1.66915671485844));
#67069=CARTESIAN_POINT('Ctrl Pts',(1.17451117462611,7.01109223591004,0.495226008491308));
#67070=CARTESIAN_POINT('Ctrl Pts',(1.14145988130163,6.90294689982591,-0.65118269685897));
#67071=CARTESIAN_POINT('Ctrl Pts',(1.10840858797715,6.79480156374177,-1.79759140220928));
#67072=CARTESIAN_POINT('Ctrl Pts',(1.07535729465267,6.39490567514344,-2.91647810654265));
#67073=CARTESIAN_POINT('Ctrl Pts',(1.0423060013282,5.7519074977916,-3.87172764323028));
#67074=CARTESIAN_POINT('Ctrl Pts',(1.00925470800372,5.10890932043973,-4.82697717991793));
#67075=CARTESIAN_POINT('Ctrl Pts',(0.976203414679236,4.22280885433436,-5.61858954895975));
#67076=CARTESIAN_POINT('Ctrl Pts',(0.943152121354756,3.20140227948802,-6.1502632668361));
#67077=CARTESIAN_POINT('Ctrl Pts',(0.910100828030278,2.17999570464171,-6.68193698471244));
#67078=CARTESIAN_POINT('Ctrl Pts',(0.877049534705799,1.02328302105442,-6.95367205142334));
#67079=CARTESIAN_POINT('Ctrl Pts',(0.843998241381321,-0.128018986403163,
-6.93241126489369));
#67080=CARTESIAN_POINT('Ctrl Pts',(0.810946948056843,-1.27932099386075,
-6.91115047836404));
#67081=CARTESIAN_POINT('Ctrl Pts',(0.777895654732364,-2.42521232518865,
-6.59689383859384));
#67082=CARTESIAN_POINT('Ctrl Pts',(0.744844361407885,-3.42629263815531,
-6.02787139579365));
#67083=CARTESIAN_POINT('Ctrl Pts',(0.711793068083405,-4.42737295112197,
-5.45884895299347));
#67084=CARTESIAN_POINT('Ctrl Pts',(0.678741774758925,-5.2836422457274,-4.63506070716328));
#67085=CARTESIAN_POINT('Ctrl Pts',(0.645690481434447,-5.89093337326648,
-3.65672241197494));
#67086=CARTESIAN_POINT('Ctrl Pts',(0.612639188109969,-6.49822450080554,
-2.67838411678662));
#67087=CARTESIAN_POINT('Ctrl Pts',(0.579587894785492,-6.85653746127826,
-1.54549577224014));
#67088=CARTESIAN_POINT('Ctrl Pts',(0.546536601461015,-6.92228265072279,
-0.395875877020612));
#67089=CARTESIAN_POINT('Ctrl Pts',(0.542748288842769,-6.92981831137959,
-0.26410737064204));
#67090=CARTESIAN_POINT('Ctrl Pts',(0.538959976224523,-6.9335103454638,-0.132119052516801));
#67091=CARTESIAN_POINT('Ctrl Pts',(0.535171663606277,-6.9334003037143,-0.000124581990723627));
#67092=CARTESIAN_POINT('Ctrl Pts',(0.355828336393729,-6.93349343740785,
-9.14711828918373E-5));
#67093=CARTESIAN_POINT('Ctrl Pts',(0.358451249680651,-6.93355318336822,
-0.0914768983207502));
#67094=CARTESIAN_POINT('Ctrl Pts',(0.361074162967572,-6.9317838549599,-0.182860009481177));
#67095=CARTESIAN_POINT('Ctrl Pts',(0.363697076254494,-6.92817041721913,
-0.27417014326238));
#67096=CARTESIAN_POINT('Ctrl Pts',(0.396748369578973,-6.88263753922595,
-1.42476785083719));
#67097=CARTESIAN_POINT('Ctrl Pts',(0.42979966290345,-6.54428804588444,-2.56377785653038));
#67098=CARTESIAN_POINT('Ctrl Pts',(0.462850956227928,-5.95428293900704,
-3.55263694735846));
#67099=CARTESIAN_POINT('Ctrl Pts',(0.495902249552406,-5.36427783212963,
-4.54149603818656));
#67100=CARTESIAN_POINT('Ctrl Pts',(0.528953542876885,-4.52261711171632,
-5.38020421414952));
#67101=CARTESIAN_POINT('Ctrl Pts',(0.562004836201364,-3.53169075948771,
-5.96673067741756));
#67102=CARTESIAN_POINT('Ctrl Pts',(0.595056129525843,-2.54076440725911,
-6.55325714068561));
#67103=CARTESIAN_POINT('Ctrl Pts',(0.628107422850322,-1.40057242321521,
-6.88760189125872));
#67104=CARTESIAN_POINT('Ctrl Pts',(0.661158716174801,-0.249821810751499,
-6.92909111358478));
#67105=CARTESIAN_POINT('Ctrl Pts',(0.69421000949928,0.900928801712209,-6.97058033591085));
#67106=CARTESIAN_POINT('Ctrl Pts',(0.727261302823757,2.0622380425957,-6.71921402998986));
#67107=CARTESIAN_POINT('Ctrl Pts',(0.760312596148236,3.09282994515598,-6.20557149083251));
#67108=CARTESIAN_POINT('Ctrl Pts',(0.793363889472715,4.12342184771625,-5.69192895167516));
#67109=CARTESIAN_POINT('Ctrl Pts',(0.826415182797194,5.02329641195328,-4.91601017928145));
#67110=CARTESIAN_POINT('Ctrl Pts',(0.859466476121673,5.68298180682118,-3.9722074946843));
#67111=CARTESIAN_POINT('Ctrl Pts',(0.892517769446152,6.34266720168907,-3.02840481008717));
#67112=CARTESIAN_POINT('Ctrl Pts',(0.925569062770629,6.76216342718784,-1.91671821328664));
#67113=CARTESIAN_POINT('Ctrl Pts',(0.958620356095107,6.89043779304345,-0.772386961105221));
#67114=CARTESIAN_POINT('Ctrl Pts',(0.991671649419586,7.01871215889905,0.371944291076227));
#67115=CARTESIAN_POINT('Ctrl Pts',(1.02472294274407,6.85576466511146,1.54892019863863));
#67116=CARTESIAN_POINT('Ctrl Pts',(1.05777423606855,6.42141825280848,2.61535890844541));
#67117=CARTESIAN_POINT('Ctrl Pts',(1.09082552939302,5.98707184050551,3.68179761825219));
#67118=CARTESIAN_POINT('Ctrl Pts',(1.1238768227175,5.28132650968716,4.63769913030343));
#67119=CARTESIAN_POINT('Ctrl Pts',(1.15692811604198,4.39003781921376,5.36677580520741));
#67120=CARTESIAN_POINT('Ctrl Pts',(1.18997940936646,3.49874912874037,6.09585248011138));
#67121=CARTESIAN_POINT('Ctrl Pts',(1.22303070269094,2.42191707861195,6.59810431786807));
#67122=CARTESIAN_POINT('Ctrl Pts',(1.25608199601542,1.29054078908523,6.81243121574038));
#67123=CARTESIAN_POINT('Ctrl Pts',(1.2891332893399,0.159164499558506,7.02675811361269));
#67124=CARTESIAN_POINT('Ctrl Pts',(1.32218458266438,-1.02675602936649,6.95316007160062));
#67125=CARTESIAN_POINT('Ctrl Pts',(1.35523587598886,-2.12295081058728,6.60059046247482));
#67126=CARTESIAN_POINT('Ctrl Pts',(1.38828716931333,-3.21914559180807,6.24802085334902));
#67127=CARTESIAN_POINT('Ctrl Pts',(1.42133846263781,-4.22561462532463,5.6164796771095));
#67128=CARTESIAN_POINT('Ctrl Pts',(1.45438975596229,-5.01991861529638,4.78279538484427));
#67129=CARTESIAN_POINT('Ctrl Pts',(1.48744104928677,-5.81422260526812,3.94911109257903));
#67130=CARTESIAN_POINT('Ctrl Pts',(1.52049234261125,-6.39636155169502,2.91328368428809));
#67131=CARTESIAN_POINT('Ctrl Pts',(1.55354363593573,-6.69551689950157,1.80132397029951));
#67132=CARTESIAN_POINT('Ctrl Pts',(1.57097186942173,-6.85326410772647,1.21497797372492));
#67133=CARTESIAN_POINT('Ctrl Pts',(1.58840010290773,-6.93232647210883,0.607463052115828));
#67134=CARTESIAN_POINT('Ctrl Pts',(1.60582833639373,-6.93241554159061,-2.91227924267906E-5));
#67135=CARTESIAN_POINT('Origin',(-3.775,0.,0.));
#67136=CARTESIAN_POINT('',(3.03517166360627,-6.93344508439855,0.000110442622268392));
#67137=CARTESIAN_POINT('',(2.85582833639373,-6.93334073279147,0.000139834461613099));
#67138=CARTESIAN_POINT('',(-3.775,-6.933,-8.4904762584886E-16));
#67139=CARTESIAN_POINT('Ctrl Pts',(3.03517166360627,-6.93344508439855,0.000110442622268392));
#67140=CARTESIAN_POINT('Ctrl Pts',(3.03190897600315,-6.93353152368877,0.113788670324413));
#67141=CARTESIAN_POINT('Ctrl Pts',(3.02864628840003,-6.93079336343887,0.227462733245047));
#67142=CARTESIAN_POINT('Ctrl Pts',(3.02538360079691,-6.92520297852914,0.340996352887752));
#67143=CARTESIAN_POINT('Ctrl Pts',(2.99233230747244,-6.86857192035748,1.49110124230881));
#67144=CARTESIAN_POINT('Ctrl Pts',(2.95928101414796,-6.51924966455837,2.62679404428279));
#67145=CARTESIAN_POINT('Ctrl Pts',(2.92622972082349,-5.91973207498778,3.60991509136462));
#67146=CARTESIAN_POINT('Ctrl Pts',(2.89317842749901,-5.32021448541714,4.59303613844651));
#67147=CARTESIAN_POINT('Ctrl Pts',(2.86012713417452,-4.470501562075,5.42358543063623));
#67148=CARTESIAN_POINT('Ctrl Pts',(2.82707584085004,-3.47396285587152,6.0005247172669));
#67149=CARTESIAN_POINT('Ctrl Pts',(2.79402454752556,-2.47742414966807,6.57746400389754));
#67150=CARTESIAN_POINT('Ctrl Pts',(2.76097325420109,-1.3340596606033,6.90079328496915));
#67151=CARTESIAN_POINT('Ctrl Pts',(2.72792196087661,-0.182962334678425,
6.93117880238228));
#67152=CARTESIAN_POINT('Ctrl Pts',(2.69487066755213,0.968134991246454,6.9615643197954));
#67153=CARTESIAN_POINT('Ctrl Pts',(2.66181937422765,2.12696515403145,6.69900607355004));
#67154=CARTESIAN_POINT('Ctrl Pts',(2.62876808090317,3.15255377254311,6.17544488419488));
#67155=CARTESIAN_POINT('Ctrl Pts',(2.59571678757869,4.17814239105477,5.65188369483972));
#67156=CARTESIAN_POINT('Ctrl Pts',(2.56266549425421,5.07048946529311,4.86731956237475));
#67157=CARTESIAN_POINT('Ctrl Pts',(2.52961420092973,5.72103890085591,3.91719653596781));
#67158=CARTESIAN_POINT('Ctrl Pts',(2.49656290760526,6.37158833641871,2.96707350956087));
#67159=CARTESIAN_POINT('Ctrl Pts',(2.46351161428078,6.78034013330596,1.85139158921196));
#67160=CARTESIAN_POINT('Ctrl Pts',(2.4304603209563,6.8975686859424,0.705876072133954));
#67161=CARTESIAN_POINT('Ctrl Pts',(2.39740902763182,7.01479723857884,-0.43963944494405));
#67162=CARTESIAN_POINT('Ctrl Pts',(2.36435773430734,6.84050254696446,-1.61498855875114));
#67163=CARTESIAN_POINT('Ctrl Pts',(2.33130644098286,6.39588796520089,-2.6771873193901));
#67164=CARTESIAN_POINT('Ctrl Pts',(2.29825514765838,5.95127338343732,-3.73938608002905));
#67165=CARTESIAN_POINT('Ctrl Pts',(2.26520385433391,5.23633891152456,-4.68843448749987));
#67166=CARTESIAN_POINT('Ctrl Pts',(2.23215256100943,4.33805798868245,-5.408878598502));
#67167=CARTESIAN_POINT('Ctrl Pts',(2.19910126768495,3.43977706584034,-6.12932270950414));
#67168=CARTESIAN_POINT('Ctrl Pts',(2.16604997436047,2.35814969206887,-6.62116252403759));
#67169=CARTESIAN_POINT('Ctrl Pts',(2.13299868103599,1.22475834988496,-6.8245645861763));
#67170=CARTESIAN_POINT('Ctrl Pts',(2.09994738771151,0.0913670077010516,
-7.02796664831501));
#67171=CARTESIAN_POINT('Ctrl Pts',(2.06689609438703,-1.09378830289531,-6.94293095805898));
#67172=CARTESIAN_POINT('Ctrl Pts',(2.03384480106255,-2.1865306853888,-6.57980230465611));
#67173=CARTESIAN_POINT('Ctrl Pts',(2.00079350773808,-3.27927306788225,-6.21667365125325));
#67174=CARTESIAN_POINT('Ctrl Pts',(1.9677422144136,-4.27960252227285,-5.57545203470356));
#67175=CARTESIAN_POINT('Ctrl Pts',(1.93469092108912,-5.0658266467822,-4.73414355414536));
#67176=CARTESIAN_POINT('Ctrl Pts',(1.90163962776464,-5.85205077129157,-3.89283507358712));
#67177=CARTESIAN_POINT('Ctrl Pts',(1.86858833444016,-6.42416956591969,-2.85143972902036));
#67178=CARTESIAN_POINT('Ctrl Pts',(1.83553704111568,-6.71258345033301,-1.73664568315478));
#67179=CARTESIAN_POINT('Ctrl Pts',(1.81874858194588,-6.85908376047037,-1.17038420170491));
#67180=CARTESIAN_POINT('Ctrl Pts',(1.80196012277608,-6.9323839809358,-0.585184762809014));
#67181=CARTESIAN_POINT('Ctrl Pts',(1.78517166360628,-6.93240903352825,8.51318353534136E-6));
#67182=CARTESIAN_POINT('Ctrl Pts',(1.60582833639373,-6.93241554159061,-2.91227924267906E-5));
#67183=CARTESIAN_POINT('Ctrl Pts',(1.62145139623221,-6.93249538547409,-0.544598749290784));
#67184=CARTESIAN_POINT('Ctrl Pts',(1.63707445607069,-6.86911440472784,-1.08915009714958));
#67185=CARTESIAN_POINT('Ctrl Pts',(1.65269751590916,-6.74206481620649,-1.61841793476135));
#67186=CARTESIAN_POINT('Ctrl Pts',(1.68574880923364,-6.47328563591869,-2.73810810614741));
#67187=CARTESIAN_POINT('Ctrl Pts',(1.71880010255812,-5.91955552615691,-3.78939642923338));
#67188=CARTESIAN_POINT('Ctrl Pts',(1.7518513958826,-5.14823704102586,-4.64439123749239));
#67189=CARTESIAN_POINT('Ctrl Pts',(1.78490268920708,-4.37691855589478,-5.49938604575143));
#67190=CARTESIAN_POINT('Ctrl Pts',(1.81795398253156,-3.38801169539442,-6.15808733918351));
#67191=CARTESIAN_POINT('Ctrl Pts',(1.85100527585604,-2.30181927622303,-6.54036257535428));
#67192=CARTESIAN_POINT('Ctrl Pts',(1.88405656918051,-1.21562685705165,-6.92263781152505));
#67193=CARTESIAN_POINT('Ctrl Pts',(1.91710786250499,-0.0321488792092285,
-7.02848699043451));
#67194=CARTESIAN_POINT('Ctrl Pts',(1.95015915582947,1.10464181221467,-6.8450333135927));
#67195=CARTESIAN_POINT('Ctrl Pts',(1.98321044915395,2.24143250363856,-6.66157963675089));
#67196=CARTESIAN_POINT('Ctrl Pts',(2.01626174247843,3.33153590864396,-6.1888231041578));
#67197=CARTESIAN_POINT('Ctrl Pts',(2.04931303580291,4.24233841582545,-5.48427564616316));
#67198=CARTESIAN_POINT('Ctrl Pts',(2.08236432912739,5.15314092300694,-4.77972818816852));
#67199=CARTESIAN_POINT('Ctrl Pts',(2.11541562245186,5.88464253236454,-3.84338980477231));
#67200=CARTESIAN_POINT('Ctrl Pts',(2.14846691577634,6.34785437392469,-2.78916823532248));
#67201=CARTESIAN_POINT('Ctrl Pts',(2.18151820910082,6.81106621548483,-1.73494666587266));
#67202=CARTESIAN_POINT('Ctrl Pts',(2.2145695024253,7.00598828924752,-0.562841910369289));
#67203=CARTESIAN_POINT('Ctrl Pts',(2.24762079574978,6.90890787215769,0.584556765014494));
#67204=CARTESIAN_POINT('Ctrl Pts',(2.28067208907426,6.81182745506786,1.73195544039831));
#67205=CARTESIAN_POINT('Ctrl Pts',(2.31372338239873,6.42274454712547,2.85464803566247));
#67206=CARTESIAN_POINT('Ctrl Pts',(2.34677467572321,5.78899198787716,3.81605638870559));
#67207=CARTESIAN_POINT('Ctrl Pts',(2.37982596904769,5.15523942862888,4.77746474174866));
#67208=CARTESIAN_POINT('Ctrl Pts',(2.41287726237217,4.2768172180747,5.57758885257073));
#67209=CARTESIAN_POINT('Ctrl Pts',(2.44592855569665,3.26058745860362,6.11909176449279));
#67210=CARTESIAN_POINT('Ctrl Pts',(2.47897984902113,2.24435769913248,6.66059467641489));
#67211=CARTESIAN_POINT('Ctrl Pts',(2.51203114234561,1.09032039074442,6.94347638943696));
#67212=CARTESIAN_POINT('Ctrl Pts',(2.54508243567009,-0.0611331472974662,
6.93332368606776));
#67213=CARTESIAN_POINT('Ctrl Pts',(2.57813372899457,-1.21258668533932,6.92317098269856));
#67214=CARTESIAN_POINT('Ctrl Pts',(2.61118502231905,-2.361456453035,6.6199838629381));
#67215=CARTESIAN_POINT('Ctrl Pts',(2.64423631564353,-3.36797977445027,6.06064574417451));
#67216=CARTESIAN_POINT('Ctrl Pts',(2.67728760896801,-4.37450309586553,5.50130762541093));
#67217=CARTESIAN_POINT('Ctrl Pts',(2.71033890229248,-5.23867997100039,4.68581850764421));
#67218=CARTESIAN_POINT('Ctrl Pts',(2.74339019561696,-5.85538127560987,3.71338453633933));
#67219=CARTESIAN_POINT('Ctrl Pts',(2.77644148894144,-6.47208258021935,2.74095056503446));
#67220=CARTESIAN_POINT('Ctrl Pts',(2.80949278226592,-6.84130831430346,1.61157174019143));
#67221=CARTESIAN_POINT('Ctrl Pts',(2.8425440755904,-6.91814130964143,0.462639619271227));
#67222=CARTESIAN_POINT('Ctrl Pts',(2.84697216252484,-6.928435102972,0.308710050970712));
#67223=CARTESIAN_POINT('Ctrl Pts',(2.85140024945929,-6.93348055652585,0.154429508353912));
#67224=CARTESIAN_POINT('Ctrl Pts',(2.85582833639373,-6.93334073279147,0.000139834461613099));
#67225=CARTESIAN_POINT('Origin',(-3.775,0.,0.));
#67226=CARTESIAN_POINT('',(4.28517166360628,-6.93277727477507,-0.000169494543622584));
#67227=CARTESIAN_POINT('',(4.10582833639373,-6.93289696494239,-0.00017817873250203));
#67228=CARTESIAN_POINT('',(-3.775,-6.933,-8.4904762584886E-16));
#67229=CARTESIAN_POINT('Ctrl Pts',(4.28517166360628,-6.93277727477507,-0.000169494543622584));
#67230=CARTESIAN_POINT('Ctrl Pts',(4.26185782923023,-6.93203240702967,0.812354315076479));
#67231=CARTESIAN_POINT('Ctrl Pts',(4.23854399485419,-6.78921230528412,1.62513310006042));
#67232=CARTESIAN_POINT('Ctrl Pts',(4.21523016047815,-6.50950105747068,2.38769989929238));
#67233=CARTESIAN_POINT('Ctrl Pts',(4.18217886715367,-6.1129631757768,3.46876698394251));
#67234=CARTESIAN_POINT('Ctrl Pts',(4.14912757382919,-5.44130358377228,4.44891879543591));
#67235=CARTESIAN_POINT('Ctrl Pts',(4.11607628050472,-4.57623123673602,5.20891759062465));
#67236=CARTESIAN_POINT('Ctrl Pts',(4.08302498718024,-3.71115888969976,5.9689163858134));
#67237=CARTESIAN_POINT('Ctrl Pts',(4.04997369385575,-2.65267378763176,6.50876216469748));
#67238=CARTESIAN_POINT('Ctrl Pts',(4.01692240053127,-1.52954309898529,6.76278143350002));
#67239=CARTESIAN_POINT('Ctrl Pts',(3.9838711072068,-0.406412410338816,7.01680070230257));
#67240=CARTESIAN_POINT('Ctrl Pts',(3.95081981388232,0.781363864886133,6.98499346102357));
#67241=CARTESIAN_POINT('Ctrl Pts',(3.91776852055784,1.88928998221405,6.67122913484938));
#67242=CARTESIAN_POINT('Ctrl Pts',(3.88471722723336,2.99721609954198,6.35746480867518));
#67243=CARTESIAN_POINT('Ctrl Pts',(3.85166593390889,4.02529205897287,5.7617433976058));
#67244=CARTESIAN_POINT('Ctrl Pts',(3.81861464058441,4.8484500327254,4.95653579488448));
#67245=CARTESIAN_POINT('Ctrl Pts',(3.78556334725993,5.67160800647792,4.15132819216316));
#67246=CARTESIAN_POINT('Ctrl Pts',(3.75251205393545,6.28984799455207,3.13663439778989));
#67247=CARTESIAN_POINT('Ctrl Pts',(3.71946076061097,6.62795966589096,2.03589426897532));
#67248=CARTESIAN_POINT('Ctrl Pts',(3.68640946728649,6.96607133722985,0.93515414016076));
#67249=CARTESIAN_POINT('Ctrl Pts',(3.65335817396201,7.02405469183348,-0.251632323095101));
#67250=CARTESIAN_POINT('Ctrl Pts',(3.62030688063753,6.79485592013532,-1.38008979082198));
#67251=CARTESIAN_POINT('Ctrl Pts',(3.58725558731305,6.56565714843717,-2.50854725854886));
#67252=CARTESIAN_POINT('Ctrl Pts',(3.55420429398857,6.04927625043723,-3.57867573074675));
#67253=CARTESIAN_POINT('Ctrl Pts',(3.52115300066409,5.30853216176314,-4.4602915929574));
#67254=CARTESIAN_POINT('Ctrl Pts',(3.48810170733961,4.56778807308904,-5.34190745516806));
#67255=CARTESIAN_POINT('Ctrl Pts',(3.45505041401514,3.60268079374078,-6.03501070739147));
#67256=CARTESIAN_POINT('Ctrl Pts',(3.42199912069066,2.53061786614165,-6.45528372900915));
#67257=CARTESIAN_POINT('Ctrl Pts',(3.38894782736618,1.45855493854251,-6.87555675062682));
#67258=CARTESIAN_POINT('Ctrl Pts',(3.3558965340417,0.279536362692491,-7.02299954163876));
#67259=CARTESIAN_POINT('Ctrl Pts',(3.32284524071722,-0.863007512958787,
-6.87967534401792));
#67260=CARTESIAN_POINT('Ctrl Pts',(3.28979394739274,-2.00555138861006,-6.73635114639708));
#67261=CARTESIAN_POINT('Ctrl Pts',(3.25674265406826,-3.1116205640626,-6.30225996014347));
#67262=CARTESIAN_POINT('Ctrl Pts',(3.22369136074378,-4.04665915483455,-5.63020998641329));
#67263=CARTESIAN_POINT('Ctrl Pts',(3.19064006741931,-4.98169774560653,-4.95816001268309));
#67264=CARTESIAN_POINT('Ctrl Pts',(3.15758877409483,-5.74570575169792,-4.04815125147631));
#67265=CARTESIAN_POINT('Ctrl Pts',(3.12453748077035,-6.24573982447149,-3.01088838243881));
#67266=CARTESIAN_POINT('Ctrl Pts',(3.09474887504899,-6.6964125922468,-2.07601983336822));
#67267=CARTESIAN_POINT('Ctrl Pts',(3.06496026932763,-6.93265588658114,-1.03778111061277));
#67268=CARTESIAN_POINT('Ctrl Pts',(3.03517166360627,-6.93344508439855,0.000110442622268392));
#67269=CARTESIAN_POINT('Ctrl Pts',(2.85582833639373,-6.93334073279147,0.000139834461613099));
#67270=CARTESIAN_POINT('Ctrl Pts',(2.88445154278377,-6.93243691051637,-0.997190444968419));
#67271=CARTESIAN_POINT('Ctrl Pts',(2.9130747491738,-6.71487431850579,-1.99490226058369));
#67272=CARTESIAN_POINT('Ctrl Pts',(2.94169795556383,-6.29768542292325,-2.90066766648421));
#67273=CARTESIAN_POINT('Ctrl Pts',(2.97474924888831,-5.81595628427528,-3.94655741432206));
#67274=CARTESIAN_POINT('Ctrl Pts',(3.00780054221279,-5.06805775038753,-4.86985149300039));
#67275=CARTESIAN_POINT('Ctrl Pts',(3.04085183553727,-4.14497341519097,-5.55822903314057));
#67276=CARTESIAN_POINT('Ctrl Pts',(3.07390312886175,-3.2218890799944,-6.24660657328076));
#67277=CARTESIAN_POINT('Ctrl Pts',(3.10695442218623,-2.12361894348903,-6.7000675748828));
#67278=CARTESIAN_POINT('Ctrl Pts',(3.14000571551071,-0.983770118937337,
-6.86344745376349));
#67279=CARTESIAN_POINT('Ctrl Pts',(3.17305700883518,0.156078705614327,-7.02682733264417));
#67280=CARTESIAN_POINT('Ctrl Pts',(3.20610830215966,1.33750621821232,-6.90012608880352));
#67281=CARTESIAN_POINT('Ctrl Pts',(3.23915959548414,2.41678901762657,-6.49875722286713));
#67282=CARTESIAN_POINT('Ctrl Pts',(3.27221088880862,3.49607181704081,-6.09738835693074));
#67283=CARTESIAN_POINT('Ctrl Pts',(3.3052621821331,4.47320990327132,-5.4213518688986));
#67284=CARTESIAN_POINT('Ctrl Pts',(3.33831347545757,5.2293321583483,-4.55288916789631));
#67285=CARTESIAN_POINT('Ctrl Pts',(3.37136476878205,5.98545441342532,-3.68442646689396));
#67286=CARTESIAN_POINT('Ctrl Pts',(3.40441606210653,6.52056083734878,-2.62353755292144));
#67287=CARTESIAN_POINT('Ctrl Pts',(3.43746735543101,6.76955449065496,-1.49928202668714));
#67288=CARTESIAN_POINT('Ctrl Pts',(3.47051864875549,7.01854814396113,-0.375026500452875));
#67289=CARTESIAN_POINT('Ctrl Pts',(3.50356994207997,6.98142902665003,0.812595638043157));
#67290=CARTESIAN_POINT('Ctrl Pts',(3.53662123540445,6.66271276556983,1.91910739693977));
#67291=CARTESIAN_POINT('Ctrl Pts',(3.56967252872893,6.34399650448963,3.02561915583639));
#67292=CARTESIAN_POINT('Ctrl Pts',(3.60272382205341,5.74368309964034,4.05102053513359));
#67293=CARTESIAN_POINT('Ctrl Pts',(3.63577511537789,4.93480207117444,4.87056907515219));
#67294=CARTESIAN_POINT('Ctrl Pts',(3.66882640870237,4.12592104270852,5.69011761517081));
#67295=CARTESIAN_POINT('Ctrl Pts',(3.70187770202685,3.10847239062599,6.3038133159108));
#67296=CARTESIAN_POINT('Ctrl Pts',(3.73492899535132,2.0062311068846,6.63699866982526));
#67297=CARTESIAN_POINT('Ctrl Pts',(3.7679802886758,0.903989823143268,6.9701840237397));
#67298=CARTESIAN_POINT('Ctrl Pts',(3.80103158200028,-0.283044092256907,
7.02285903082863));
#67299=CARTESIAN_POINT('Ctrl Pts',(3.83408287532476,-1.41046520618992,6.7886156541341));
#67300=CARTESIAN_POINT('Ctrl Pts',(3.86713416864924,-2.53788632012296,6.55437227743956));
#67301=CARTESIAN_POINT('Ctrl Pts',(3.90018546197372,-3.60569463258884,6.03321051696155));
#67302=CARTESIAN_POINT('Ctrl Pts',(3.9332367552982,-4.48398878192539,5.28853091143765));
#67303=CARTESIAN_POINT('Ctrl Pts',(3.96628804862267,-5.36228293126194,4.54385130591376));
#67304=CARTESIAN_POINT('Ctrl Pts',(3.99933934194715,-6.05106291746916,3.57565385534399));
#67305=CARTESIAN_POINT('Ctrl Pts',(4.03239063527163,-6.4665370553702,2.50172202864973));
#67306=CARTESIAN_POINT('Ctrl Pts',(4.056869868979,-6.77425537734927,1.70632113727346));
#67307=CARTESIAN_POINT('Ctrl Pts',(4.08134910268637,-6.93205091289159,0.852919319868787));
#67308=CARTESIAN_POINT('Ctrl Pts',(4.10582833639373,-6.93289696494239,-0.00017817873250203));
#67309=CARTESIAN_POINT('Origin',(-3.775,0.,0.));
#67310=CARTESIAN_POINT('',(5.53517166360628,-6.93272540515737,0.000163154062267218));
#67311=CARTESIAN_POINT('',(5.35582833639373,-6.93262081645922,0.000142250729870931));
#67312=CARTESIAN_POINT('',(-3.775,-6.933,-8.4904762584886E-16));
#67313=CARTESIAN_POINT('Ctrl Pts',(5.53517166360628,-6.93272540515737,0.000163154062267218));
#67314=CARTESIAN_POINT('Ctrl Pts',(5.52485797578179,-6.93303262791813,0.359618454679378));
#67315=CARTESIAN_POINT('Ctrl Pts',(5.51454428795731,-6.9055597149569,0.719026621772691));
#67316=CARTESIAN_POINT('Ctrl Pts',(5.50423060013282,-6.8498977578155,1.07401516670493));
#67317=CARTESIAN_POINT('Ctrl Pts',(5.47117930680834,-6.67152318377348,2.21161315542136));
#67318=CARTESIAN_POINT('Ctrl Pts',(5.43812801348386,-6.20366145138839,3.30382387055088));
#67319=CARTESIAN_POINT('Ctrl Pts',(5.40507672015939,-5.50319805732819,4.21776921297274));
#67320=CARTESIAN_POINT('Ctrl Pts',(5.37202542683491,-4.802734663268,5.1317145553946));
#67321=CARTESIAN_POINT('Ctrl Pts',(5.33897413351042,-3.86966960753269,5.86739452510881));
#67322=CARTESIAN_POINT('Ctrl Pts',(5.30592284018595,-2.817528404932,6.33531613923483));
#67323=CARTESIAN_POINT('Ctrl Pts',(5.27287154686147,-1.7653872023313,6.80323775336085));
#67324=CARTESIAN_POINT('Ctrl Pts',(5.23982025353699,-0.59416985286522,7.00340101189867));
#67325=CARTESIAN_POINT('Ctrl Pts',(5.20676896021251,0.553650582751667,6.91145342449458));
#67326=CARTESIAN_POINT('Ctrl Pts',(5.17371766688803,1.70147101836855,6.81950583709048));
#67327=CARTESIAN_POINT('Ctrl Pts',(5.14066637356355,2.82589454013615,6.4354474037445));
#67328=CARTESIAN_POINT('Ctrl Pts',(5.10761508023908,3.79012815577094,5.80600084257848));
#67329=CARTESIAN_POINT('Ctrl Pts',(5.0745637869146,4.75436177140573,5.17655428141245));
#67330=CARTESIAN_POINT('Ctrl Pts',(5.04151249359012,5.55840548090767,4.30171959242633));
#67331=CARTESIAN_POINT('Ctrl Pts',(5.00846120026564,6.10444769783574,3.28792187076906));
#67332=CARTESIAN_POINT('Ctrl Pts',(4.97540990694116,6.65048991476382,2.27412414911179));
#67333=CARTESIAN_POINT('Ctrl Pts',(4.94235861361668,6.9385306391181,1.12136339478331));
#67334=CARTESIAN_POINT('Ctrl Pts',(4.9093073202922,6.93352791278986,-0.0301240709127577));
#67335=CARTESIAN_POINT('Ctrl Pts',(4.87625602696772,6.92852518646162,-1.18161153660883));
#67336=CARTESIAN_POINT('Ctrl Pts',(4.84320473364324,6.63047900945084,-2.3318257136725));
#67337=CARTESIAN_POINT('Ctrl Pts',(4.81015344031876,6.07564797737095,-3.34084052937886));
#67338=CARTESIAN_POINT('Ctrl Pts',(4.77710214699428,5.52081694529103,-4.34985534508526));
#67339=CARTESIAN_POINT('Ctrl Pts',(4.74405085366981,4.70920105814205,-5.21767079943428));
#67340=CARTESIAN_POINT('Ctrl Pts',(4.71099956034533,3.73953497146248,-5.83871504720933));
#67341=CARTESIAN_POINT('Ctrl Pts',(4.67794826702085,2.76986888478297,-6.45975929498434));
#67342=CARTESIAN_POINT('Ctrl Pts',(4.64489697369637,1.64215259857284,-6.83403233618537));
#67343=CARTESIAN_POINT('Ctrl Pts',(4.61184568037189,0.493575574722173,-6.91600302692225));
#67344=CARTESIAN_POINT('Ctrl Pts',(4.57879438704741,-0.655001449128527,
-6.99797371765914));
#67345=CARTESIAN_POINT('Ctrl Pts',(4.54574309372293,-1.82443921061986,-6.78764205793191));
#67346=CARTESIAN_POINT('Ctrl Pts',(4.51269180039845,-2.87247297018407,-6.31059536157588));
#67347=CARTESIAN_POINT('Ctrl Pts',(4.47964050707397,-3.92050672974827,-5.83354866521985));
#67348=CARTESIAN_POINT('Ctrl Pts',(4.4465892137495,-4.84713648738534,-5.08978693223501));
#67349=CARTESIAN_POINT('Ctrl Pts',(4.41353792042502,-5.53963553902198,-4.16979051602946));
#67350=CARTESIAN_POINT('Ctrl Pts',(4.38048662710054,-6.23213459065862,-3.2497940998239));
#67351=CARTESIAN_POINT('Ctrl Pts',(4.34743533377606,-6.69050293629485,-2.15356300039762));
#67352=CARTESIAN_POINT('Ctrl Pts',(4.31438404045158,-6.85897902342132,-1.01445627178106));
#67353=CARTESIAN_POINT('Ctrl Pts',(4.30464658150315,-6.90861487173992,-0.678856545050398));
#67354=CARTESIAN_POINT('Ctrl Pts',(4.29490912255471,-6.93308838271965,-0.339535259659124));
#67355=CARTESIAN_POINT('Ctrl Pts',(4.28517166360628,-6.93277727477507,-0.000169494543622584));
#67356=CARTESIAN_POINT('Ctrl Pts',(4.10582833639373,-6.93289696494239,-0.00017817873250203));
#67357=CARTESIAN_POINT('Ctrl Pts',(4.11440039601084,-6.9331932327384,-0.298913127082497));
#67358=CARTESIAN_POINT('Ctrl Pts',(4.12297245562795,-6.91424376032206,-0.597610758708019));
#67359=CARTESIAN_POINT('Ctrl Pts',(4.13154451524506,-6.87574682128536,-0.893767446093456));
#67360=CARTESIAN_POINT('Ctrl Pts',(4.16459580856954,-6.72731415970462,-2.03565889132375));
#67361=CARTESIAN_POINT('Ctrl Pts',(4.19764710189402,-6.28828054694824,-3.13977557896555));
#67362=CARTESIAN_POINT('Ctrl Pts',(4.2306983952185,-5.61205544221947,-4.07179914905405));
#67363=CARTESIAN_POINT('Ctrl Pts',(4.26374968854298,-4.93583033749073,-5.0038227191425));
#67364=CARTESIAN_POINT('Ctrl Pts',(4.29680098186746,-4.02241374078962,-5.76375317167767));
#67365=CARTESIAN_POINT('Ctrl Pts',(4.32985227519194,-2.98292490212011,-6.25914320221618));
#67366=CARTESIAN_POINT('Ctrl Pts',(4.36290356851642,-1.94343606345054,-6.75453323275473));
#67367=CARTESIAN_POINT('Ctrl Pts',(4.3959548618409,-0.777874982812544,-6.98538284129659));
#67368=CARTESIAN_POINT('Ctrl Pts',(4.42900615516538,0.371965125420105,-6.92360863606738));
#67369=CARTESIAN_POINT('Ctrl Pts',(4.46205744848986,1.52180523365269,-6.86183443083818));
#67370=CARTESIAN_POINT('Ctrl Pts',(4.49510874181433,2.65592436947993,-6.50743641183794));
#67371=CARTESIAN_POINT('Ctrl Pts',(4.52816003513881,3.6363543084025,-5.90352792257827));
#67372=CARTESIAN_POINT('Ctrl Pts',(4.56121132846329,4.6167842473251,-5.29961943331858));
#67373=CARTESIAN_POINT('Ctrl Pts',(4.59426262178776,5.44352498934302,-4.44620047379944));
#67374=CARTESIAN_POINT('Ctrl Pts',(4.62731391511224,6.01600159733496,-3.44709144037499));
#67375=CARTESIAN_POINT('Ctrl Pts',(4.66036520843672,6.5884782053269,-2.44798240695053));
#67376=CARTESIAN_POINT('Ctrl Pts',(4.69341650176121,6.90669067929286,-1.30318329962076));
#67377=CARTESIAN_POINT('Ctrl Pts',(4.72646779508568,6.93192774311814,-0.15196159380743));
#67378=CARTESIAN_POINT('Ctrl Pts',(4.75951908841016,6.95716480694343,0.999260112005898));
#67379=CARTESIAN_POINT('Ctrl Pts',(4.79257038173464,6.68942646062803,2.15690441630278));
#67380=CARTESIAN_POINT('Ctrl Pts',(4.82562167505912,6.16128367556587,3.18014120963901));
#67381=CARTESIAN_POINT('Ctrl Pts',(4.8586729683836,5.63314089050373,4.20337800297521));
#67382=CARTESIAN_POINT('Ctrl Pts',(4.89172426170808,4.84459366669486,5.09220728535076));
#67383=CARTESIAN_POINT('Ctrl Pts',(4.92477555503256,3.89157064504942,5.73850089200341));
#67384=CARTESIAN_POINT('Ctrl Pts',(4.95782684835704,2.93854762340393,6.38479449865609));
#67385=CARTESIAN_POINT('Ctrl Pts',(4.99087814168152,1.82104880392187,6.78855242958583));
#67386=CARTESIAN_POINT('Ctrl Pts',(5.023929435006,0.675020437465834,6.90065662929625));
#67387=CARTESIAN_POINT('Ctrl Pts',(5.05698072833047,-0.471007928990167,
7.01276082900667));
#67388=CARTESIAN_POINT('Ctrl Pts',(5.09003202165495,-1.64556584242014,6.83321129749778));
#67389=CARTESIAN_POINT('Ctrl Pts',(5.12308331497943,-2.70576545644266,6.3838505851852));
#67390=CARTESIAN_POINT('Ctrl Pts',(5.15613460830391,-3.7659650704652,5.93448987287263));
#67391=CARTESIAN_POINT('Ctrl Pts',(5.18918590162839,-4.71180638508021,5.21531797975642));
#67392=CARTESIAN_POINT('Ctrl Pts',(5.22223719495287,-5.42822589358189,4.31382396725108));
#67393=CARTESIAN_POINT('Ctrl Pts',(5.25528848827735,-6.14464540208356,3.41232995474574));
#67394=CARTESIAN_POINT('Ctrl Pts',(5.28833978160182,-6.63164310447184,2.32851382285121));
#67395=CARTESIAN_POINT('Ctrl Pts',(5.3213910749263,-6.82997404460943,1.19422406973633));
#67396=CARTESIAN_POINT('Ctrl Pts',(5.33287016208211,-6.89885661828612,0.800272438006842));
#67397=CARTESIAN_POINT('Ctrl Pts',(5.34434924923792,-6.93291872661601,0.400232419221871));
#67398=CARTESIAN_POINT('Ctrl Pts',(5.35582833639373,-6.93262081645922,0.000142250729870931));
#67399=CARTESIAN_POINT('Origin',(-15.9277445817596,0.,0.));
#67400=CARTESIAN_POINT('',(5.94725541824039,-6.21900367460334,0.000146357406630245));
#67401=CARTESIAN_POINT('',(6.,-6.21925,-5.19709976349859E-13));
#67402=CARTESIAN_POINT('',(-15.9277445817596,-6.21925,-5.19709976349859E-13));
#67403=CARTESIAN_POINT('',(6.,-6.00216240205941,-1.62981090527758));
#67404=CARTESIAN_POINT('Ctrl Pts',(5.94725541824039,-6.21900367460334,0.000146357406630437));
#67405=CARTESIAN_POINT('Ctrl Pts',(5.96483694549359,-6.21853387481332,-0.54952653898896));
#67406=CARTESIAN_POINT('Ctrl Pts',(5.9824184727468,-6.14564776188864,-1.09932230145161));
#67407=CARTESIAN_POINT('Ctrl Pts',(6.,-6.00216240205941,-1.62981090527758));
#67408=CARTESIAN_POINT('Origin',(6.,0.,0.));
#67409=CARTESIAN_POINT('Origin',(-15.9277445817596,0.,0.));
#67410=CARTESIAN_POINT('',(4.69725541824038,-6.21905020426149,-0.000152045137862922));
#67411=CARTESIAN_POINT('',(4.94374458175965,-6.21890985327621,0.000127606064774521));
#67412=CARTESIAN_POINT('',(-15.9277445817596,-6.21925,-5.19709976349859E-13));
#67413=CARTESIAN_POINT('Ctrl Pts',(4.69725541824038,-6.21905020426149,-0.00015204513786251));
#67414=CARTESIAN_POINT('Ctrl Pts',(4.70699287718881,-6.21932928374862,-0.304580219765699));
#67415=CARTESIAN_POINT('Ctrl Pts',(4.74978162946173,-6.1228582182286,-1.64213599516804));
#67416=CARTESIAN_POINT('Ctrl Pts',(4.82562167505912,-5.17935896716503,-3.89860337811007));
#67417=CARTESIAN_POINT('Ctrl Pts',(4.92477555503255,-2.68565835263266,-5.90017852214549));
#67418=CARTESIAN_POINT('Ctrl Pts',(5.02392943500599,0.461475268377732,-6.46621278210156));
#67419=CARTESIAN_POINT('Ctrl Pts',(5.12308331497942,3.49633009875934,-5.45898750668426));
#67420=CARTESIAN_POINT('Ctrl Pts',(5.22223719495286,5.68051101877298,-3.1235650642522));
#67421=CARTESIAN_POINT('Ctrl Pts',(5.3213910749263,6.48259829111145,-0.0281650120223385));
#67422=CARTESIAN_POINT('Ctrl Pts',(5.42054495489973,5.70743720286374,3.07408826420326));
#67423=CARTESIAN_POINT('Ctrl Pts',(5.51969883487318,3.54363415642518,5.42840052706632));
#67424=CARTESIAN_POINT('Ctrl Pts',(5.6188527148466,0.51764065242096,6.46195977050514));
#67425=CARTESIAN_POINT('Ctrl Pts',(5.71800659482005,-2.63428210857727,5.92329021374989));
#67426=CARTESIAN_POINT('Ctrl Pts',(5.81716047479348,-5.14530108213061,3.94346431515829));
#67427=CARTESIAN_POINT('Ctrl Pts',(5.89357674926693,-6.11565852522162,1.67819078777056));
#67428=CARTESIAN_POINT('Ctrl Pts',(5.9369417304159,-6.21927926888502,0.322595856665736));
#67429=CARTESIAN_POINT('Ctrl Pts',(5.94725541824039,-6.21900367460334,0.000146357406630437));
#67430=CARTESIAN_POINT('',(6.,-3.49587713861109,5.14372565308808));
#67431=CARTESIAN_POINT('Origin',(6.,0.,0.));
#67432=CARTESIAN_POINT('Ctrl Pts',(4.94374458175965,-6.21890985327621,0.000127606064774174));
#67433=CARTESIAN_POINT('Ctrl Pts',(4.96531678792832,-6.21840763867658,-0.674341253668515));
#67434=CARTESIAN_POINT('Ctrl Pts',(5.01994028742146,-5.94150400537597,-2.38258228935399));
#67435=CARTESIAN_POINT('Ctrl Pts',(5.10761508023907,-4.40502769148852,-4.75611250736834));
#67436=CARTESIAN_POINT('Ctrl Pts',(5.20676896021251,-1.59561249292064,-6.28322342394515));
#67437=CARTESIAN_POINT('Ctrl Pts',(5.30592284018595,1.60200834941566,-6.28159039988369));
#67438=CARTESIAN_POINT('Ctrl Pts',(5.40507672015938,4.40988078716951,-4.75162981867586));
#67439=CARTESIAN_POINT('Ctrl Pts',(5.50423060013282,6.14475515867778,-2.06555128428737));
#67440=CARTESIAN_POINT('Ctrl Pts',(5.60338448010625,6.38468584605272,1.12303831208186));
#67441=CARTESIAN_POINT('Ctrl Pts',(5.7025383600797,5.07099150144849,4.03847901383656));
#67442=CARTESIAN_POINT('Ctrl Pts',(5.80169224005312,2.52389427730921,5.97115958776782));
#67443=CARTESIAN_POINT('Ctrl Pts',(5.90084612002658,-0.638069512693321,
6.45139792173227));
#67444=CARTESIAN_POINT('Ctrl Pts',(5.96694870667552,-2.64132982999147,5.72450942764096));
#67445=CARTESIAN_POINT('Ctrl Pts',(6.,-3.49587713861109,5.14372565308808));
#67446=CARTESIAN_POINT('Origin',(-15.9277445817596,0.,0.));
#67447=CARTESIAN_POINT('',(3.44725541824037,-6.21964926311058,9.90725915984747E-5));
#67448=CARTESIAN_POINT('',(3.69374458175965,-6.21915757236664,-0.000159835292970756));
#67449=CARTESIAN_POINT('',(-15.9277445817596,-6.21925,-5.19709976349859E-13));
#67450=CARTESIAN_POINT('Ctrl Pts',(3.44725541824037,-6.21964926311058,9.90725915984633E-5));
#67451=CARTESIAN_POINT('Ctrl Pts',(3.47704402396173,-6.21894131294095,-0.930941897040162));
#67452=CARTESIAN_POINT('Ctrl Pts',(3.53988392300757,-5.77188564316155,-2.89565589622528));
#67453=CARTESIAN_POINT('Ctrl Pts',(3.63577511537788,-3.78348001045424,-5.26404278768421));
#67454=CARTESIAN_POINT('Ctrl Pts',(3.73492899535132,-0.806880824200139,
-6.43224772498744));
#67455=CARTESIAN_POINT('Ctrl Pts',(3.83408287532476,2.36603621511411,-6.03545690802462));
#67456=CARTESIAN_POINT('Ctrl Pts',(3.93323675529819,4.96328565132639,-4.17021138600364));
#67457=CARTESIAN_POINT('Ctrl Pts',(4.03239063527163,6.35294463007415,-1.29033405986049));
#67458=CARTESIAN_POINT('Ctrl Pts',(4.13154451524507,6.1969026663707,1.90348753754495));
#67459=CARTESIAN_POINT('Ctrl Pts',(4.2306983952185,4.53312549379163,4.63418177409014));
#67460=CARTESIAN_POINT('Ctrl Pts',(4.32985227519194,1.76641783014358,6.23735805526417));
#67461=CARTESIAN_POINT('Ctrl Pts',(4.42900615516537,-1.430067500749,6.32295614497614));
#67462=CARTESIAN_POINT('Ctrl Pts',(4.52816003513881,-4.27861075952717,4.87014962817609));
#67463=CARTESIAN_POINT('Ctrl Pts',(4.61757645616381,-5.90863799280524,2.4914533890396));
#67464=CARTESIAN_POINT('Ctrl Pts',(4.67394158386433,-6.218382020398,0.728722713693786));
#67465=CARTESIAN_POINT('Ctrl Pts',(4.69725541824038,-6.21905020426149,-0.00015204513786251));
#67466=CARTESIAN_POINT('Ctrl Pts',(3.69374458175965,-6.21915757236664,-0.000159835292970999));
#67467=CARTESIAN_POINT('Ctrl Pts',(3.70231664137676,-6.21942333949345,-0.268140121968968));
#67468=CARTESIAN_POINT('Ctrl Pts',(3.74393999431834,-6.13688308256028,-1.56920955113219));
#67469=CARTESIAN_POINT('Ctrl Pts',(3.8186146405844,-5.24706894496936,-3.80698499626393));
#67470=CARTESIAN_POINT('Ctrl Pts',(3.91776852055784,-2.78892694192586,-5.85207260635886));
#67471=CARTESIAN_POINT('Ctrl Pts',(4.01692240053128,0.347773945463821,-6.47332376513164));
#67472=CARTESIAN_POINT('Ctrl Pts',(4.11607628050471,3.3998598111037,-5.51958517592035));
#67473=CARTESIAN_POINT('Ctrl Pts',(4.21523016047815,5.62474399967788,-3.2229058751893));
#67474=CARTESIAN_POINT('Ctrl Pts',(4.31438404045158,6.48110182257391,-0.142078593380259));
#67475=CARTESIAN_POINT('Ctrl Pts',(4.41353792042502,5.76057749963056,2.97331705330878));
#67476=CARTESIAN_POINT('Ctrl Pts',(4.51269180039846,3.63847783642259,5.36529088040279));
#67477=CARTESIAN_POINT('Ctrl Pts',(4.6118456803719,0.631119752015993,6.45186444679596));
#67478=CARTESIAN_POINT('Ctrl Pts',(4.71099956034532,-2.5297929710906,5.96866954249621));
#67479=CARTESIAN_POINT('Ctrl Pts',(4.81015344031878,-5.07519478672013,4.03326937102785));
#67480=CARTESIAN_POINT('Ctrl Pts',(4.88773511412354,-6.10064460767951,1.75112501397285));
#67481=CARTESIAN_POINT('Ctrl Pts',(4.93226549460384,-6.21917709368338,0.359028627324734));
#67482=CARTESIAN_POINT('Ctrl Pts',(4.94374458175965,-6.21890985327621,0.000127606064774174));
#67483=CARTESIAN_POINT('Origin',(-15.9277445817596,0.,0.));
#67484=CARTESIAN_POINT('',(2.19725541824037,-6.21871987332621,7.63675412254265E-6));
#67485=CARTESIAN_POINT('',(2.44374458175965,-6.21955565446608,0.000125438550603943));
#67486=CARTESIAN_POINT('',(-15.9277445817596,-6.21925,-5.19709976349859E-13));
#67487=CARTESIAN_POINT('Ctrl Pts',(2.19725541824037,-6.21871987332621,7.6367541225128E-6));
#67488=CARTESIAN_POINT('Ctrl Pts',(2.21404387741017,-6.21869739988965,-0.524940189831289));
#67489=CARTESIAN_POINT('Ctrl Pts',(2.26388362990446,-6.02349410963766,-2.08336464204647));
#67490=CARTESIAN_POINT('Ctrl Pts',(2.34677467572321,-4.7363647693443,-4.42625306910482));
#67491=CARTESIAN_POINT('Ctrl Pts',(2.44592855569665,-2.04432714095016,-6.15187727452525));
#67492=CARTESIAN_POINT('Ctrl Pts',(2.54508243567009,1.14510477831697,-6.38072115882848));
#67493=CARTESIAN_POINT('Ctrl Pts',(2.64423631564352,4.05592738512275,-5.05710594180675));
#67494=CARTESIAN_POINT('Ctrl Pts',(2.74339019561696,5.97992401621031,-2.50307335497727));
#67495=CARTESIAN_POINT('Ctrl Pts',(2.84254407559039,6.44897735278439,0.659968607828769));
#67496=CARTESIAN_POINT('Ctrl Pts',(2.94169795556383,5.3489645389414,3.6624371422857));
#67497=CARTESIAN_POINT('Ctrl Pts',(3.04085183553727,2.94752380269873,5.77381770517306));
#67498=CARTESIAN_POINT('Ctrl Pts',(3.1400057155107,-0.171063168266469,6.48040159654536));
#67499=CARTESIAN_POINT('Ctrl Pts',(3.23915959548414,-3.2480296756728,5.61027367300375));
#67500=CARTESIAN_POINT('Ctrl Pts',(3.33831347545758,-5.53473547337747,3.37514010076197));
#67501=CARTESIAN_POINT('Ctrl Pts',(3.40767874970965,-6.1923883436481,1.23702373810622));
#67502=CARTESIAN_POINT('Ctrl Pts',(3.44399273063725,-6.21972680350518,0.10207416528405));
#67503=CARTESIAN_POINT('Ctrl Pts',(3.44725541824037,-6.21964926311058,9.90725915984633E-5));
#67504=CARTESIAN_POINT('Ctrl Pts',(2.44374458175965,-6.21955565446608,0.000125438550604151));
#67505=CARTESIAN_POINT('Ctrl Pts',(2.47236778814968,-6.21874488038776,-0.894530026665607));
#67506=CARTESIAN_POINT('Ctrl Pts',(2.53404228786418,-5.7982231990549,-2.82298402379256));
#67507=CARTESIAN_POINT('Ctrl Pts',(2.62876808090318,-3.87540028951621,-5.19674319871096));
#67508=CARTESIAN_POINT('Ctrl Pts',(2.7279219608766,-0.919789494855471,-6.41707523428578));
#67509=CARTESIAN_POINT('Ctrl Pts',(2.82707584085005,2.25961035703773,-6.07610305308455));
#67510=CARTESIAN_POINT('Ctrl Pts',(2.92622972082348,4.88923651142507,-4.25678677087163));
#67511=CARTESIAN_POINT('Ctrl Pts',(3.02538360079692,6.32928870830338,-1.40177449124226));
#67512=CARTESIAN_POINT('Ctrl Pts',(3.12453748077035,6.22939555800606,1.79429603443556));
#67513=CARTESIAN_POINT('Ctrl Pts',(3.22369136074379,4.61386152810167,4.55380599903706));
#67514=CARTESIAN_POINT('Ctrl Pts',(3.32284524071722,1.87575355343092,6.20535380813579));
#67515=CARTESIAN_POINT('Ctrl Pts',(3.42199912069066,-1.31873397506443,6.34711020702708));
#67516=CARTESIAN_POINT('Ctrl Pts',(3.5211530006641,-4.19236740098541,4.94458520535987));
#67517=CARTESIAN_POINT('Ctrl Pts',(3.61173482102043,-5.88572982976849,2.56427622532341));
#67518=CARTESIAN_POINT('Ctrl Pts',(3.66926534805228,-6.21839862108777,0.76511156499223));
#67519=CARTESIAN_POINT('Ctrl Pts',(3.69374458175965,-6.21915757236664,-0.000159835292970999));
#67520=CARTESIAN_POINT('Origin',(-15.9277445817596,0.,0.));
#67521=CARTESIAN_POINT('',(0.947255418240376,-6.2196090925826,-0.000111756317149322));
#67522=CARTESIAN_POINT('',(1.19374458175965,-6.21872571138575,-2.6124611402778E-5));
#67523=CARTESIAN_POINT('',(-15.9277445817596,-6.21925,-5.19709976349859E-13));
#67524=CARTESIAN_POINT('Ctrl Pts',(0.947255418240376,-6.2196090925826,-0.000111756317148926));
#67525=CARTESIAN_POINT('Ctrl Pts',(0.95104373085862,-6.21970780557128,-0.11851744084317));
#67526=CARTESIAN_POINT('Ctrl Pts',(0.987883336801342,-6.18750070111082,
-1.26990484747838));
#67527=CARTESIAN_POINT('Ctrl Pts',(1.05777423606854,-5.50780972843139,-3.4189032533025));
#67528=CARTESIAN_POINT('Ctrl Pts',(1.15692811604198,-3.20345974553442,-5.63584182875872));
#67529=CARTESIAN_POINT('Ctrl Pts',(1.25608199601542,-0.119693124002174,
-6.48155390443623));
#67530=CARTESIAN_POINT('Ctrl Pts',(1.35523587598885,2.99319539066687,-5.75027380333636));
#67531=CARTESIAN_POINT('Ctrl Pts',(1.45438975596229,5.3778255610804,-3.61992537141806));
#67532=CARTESIAN_POINT('Ctrl Pts',(1.55354363593573,6.45400578832633,-0.608832279282255));
#67533=CARTESIAN_POINT('Ctrl Pts',(1.65269751590916,5.95989642342674,2.55039253489949));
#67534=CARTESIAN_POINT('Ctrl Pts',(1.7518513958826,4.01571657038161,5.08909499679543));
#67535=CARTESIAN_POINT('Ctrl Pts',(1.85100527585604,1.09449421965509,6.38959700319101));
#67536=CARTESIAN_POINT('Ctrl Pts',(1.95015915582947,-2.09302365948521,6.13548037409304));
#67537=CARTESIAN_POINT('Ctrl Pts',(2.04931303580291,-4.77129915855997,4.38857286592929));
#67538=CARTESIAN_POINT('Ctrl Pts',(2.13167845660654,-6.03177409386706,2.05047689312513));
#67539=CARTESIAN_POINT('Ctrl Pts',(2.1809925840857,-6.21874164314844,0.508520023583037));
#67540=CARTESIAN_POINT('Ctrl Pts',(2.19725541824037,-6.21871987332621,7.6367541225128E-6));
#67541=CARTESIAN_POINT('Ctrl Pts',(1.19374458175965,-6.21872571138575,-2.61246114025351E-5));
#67542=CARTESIAN_POINT('Ctrl Pts',(1.20936764159813,-6.21879733536845,-0.488532492648138));
#67543=CARTESIAN_POINT('Ctrl Pts',(1.25804199476107,-6.04166009992344,-2.0104452049757));
#67544=CARTESIAN_POINT('Ctrl Pts',(1.3397676412485,-4.81341550856989,-4.34233789785988));
#67545=CARTESIAN_POINT('Ctrl Pts',(1.43892152122194,-2.15211780533888,-6.11500255349699));
#67546=CARTESIAN_POINT('Ctrl Pts',(1.53807540119537,1.03280015818185,-6.39985867895463));
#67547=CARTESIAN_POINT('Ctrl Pts',(1.63722928116881,3.96643304506188,-5.12759945553204));
#67548=CARTESIAN_POINT('Ctrl Pts',(1.73638316114225,5.93501434493084,-2.60777146291548));
#67549=CARTESIAN_POINT('Ctrl Pts',(1.83553704111568,6.45957908194884,0.546539441742633));
#67550=CARTESIAN_POINT('Ctrl Pts',(1.93469092108912,5.41249821859067,3.56787476112659));
#67551=CARTESIAN_POINT('Ctrl Pts',(2.03384480106256,3.0485313934114,5.72112957559227));
#67552=CARTESIAN_POINT('Ctrl Pts',(2.13299868103599,-0.0571572825696857,
6.48240698524711));
#67553=CARTESIAN_POINT('Ctrl Pts',(2.23215256100943,-3.14893932616178,5.66648465960009));
#67554=CARTESIAN_POINT('Ctrl Pts',(2.33130644098286,-5.47456980244149,3.471880291071));
#67555=CARTESIAN_POINT('Ctrl Pts',(2.40183711456627,-6.18137274724245,1.30992838602558));
#67556=CARTESIAN_POINT('Ctrl Pts',(2.4393164948252,-6.21968108339441,0.13853104281368));
#67557=CARTESIAN_POINT('Ctrl Pts',(2.44374458175965,-6.21955565446608,0.000125438550604151));
#67558=CARTESIAN_POINT('Origin',(-15.9277445817596,0.,0.));
#67559=CARTESIAN_POINT('',(-0.30274458175963,-6.21909759658405,0.000156462538848766));
#67560=CARTESIAN_POINT('',(-0.0562554182403474,-6.21969263819396,-8.20542562895987E-5));
#67561=CARTESIAN_POINT('',(-15.9277445817596,-6.21925,-5.19709976349859E-13));
#67562=CARTESIAN_POINT('Ctrl Pts',(-0.30274458175963,-6.21909759658405,
0.000156462538848587));
#67563=CARTESIAN_POINT('Ctrl Pts',(-0.278905122368461,-6.21838583129681,
-0.745134927932084));
#67564=CARTESIAN_POINT('Ctrl Pts',(-0.222014369652814,-5.89839721002363,
-2.52430138060163));
#67565=CARTESIAN_POINT('Ctrl Pts',(-0.132072323612687,-4.2398747970514,
-4.9039095796491));
#67566=CARTESIAN_POINT('Ctrl Pts',(-0.0329184436392546,-1.37990584390503,
-6.33409246238185));
#67567=CARTESIAN_POINT('Ctrl Pts',(0.0662354363341833,1.81580061179276,
-6.22316122226147));
#67568=CARTESIAN_POINT('Ctrl Pts',(0.165389316307621,4.56971434284393,-4.59810594537058));
#67569=CARTESIAN_POINT('Ctrl Pts',(0.264543196281055,6.21179534442574,-1.85431013021464));
#67570=CARTESIAN_POINT('Ctrl Pts',(0.363697076254493,6.34251768011774,1.34064795432643));
#67571=CARTESIAN_POINT('Ctrl Pts',(0.462850956227929,4.93007599833982,4.20942016323384));
#67572=CARTESIAN_POINT('Ctrl Pts',(0.562004836201364,2.31812392215191,6.05402089041596));
#67573=CARTESIAN_POINT('Ctrl Pts',(0.6611587161748,-0.857838473773044,6.42565020935318));
#67574=CARTESIAN_POINT('Ctrl Pts',(0.76031259614824,-3.82508478370621,5.23388898024262));
#67575=CARTESIAN_POINT('Ctrl Pts',(0.855678163503428,-5.78385960214847,
2.86288430550369));
#67576=CARTESIAN_POINT('Ctrl Pts',(0.917992437534142,-6.21884657993534,
0.914517951143361));
#67577=CARTESIAN_POINT('Ctrl Pts',(0.947255418240376,-6.2196090925826,-0.000111756317148926));
#67578=CARTESIAN_POINT('Ctrl Pts',(-0.0562554182403475,-6.21969263819397,
-8.20542562896334E-5));
#67579=CARTESIAN_POINT('Ctrl Pts',(-0.0536325049534321,-6.21974623332796,
-0.0820593826459758));
#67580=CARTESIAN_POINT('Ctrl Pts',(-0.0179582983420387,-6.19815906612472,
-1.197003612836));
#67581=CARTESIAN_POINT('Ctrl Pts',(0.0507672015938321,-5.56703928211486,
-3.32158710689955));
#67582=CARTESIAN_POINT('Ctrl Pts',(0.149921081567268,-3.30200317851016,
-5.5786774675043));
#67583=CARTESIAN_POINT('Ctrl Pts',(0.249074961540705,-0.233574361216745,
-6.47844968299619));
#67584=CARTESIAN_POINT('Ctrl Pts',(0.348228841514139,2.89168418329416,-5.8019849932086));
#67585=CARTESIAN_POINT('Ctrl Pts',(0.447382721487577,5.31338253190132,-3.71387039986819));
#67586=CARTESIAN_POINT('Ctrl Pts',(0.546536601461015,6.44231022572788,-0.722153884441094));
#67587=CARTESIAN_POINT('Ctrl Pts',(0.645690481434449,6.00379391212401,2.44526602603354));
#67588=CARTESIAN_POINT('Ctrl Pts',(0.744844361407886,4.10452664743683,5.01774135222336));
#67589=CARTESIAN_POINT('Ctrl Pts',(0.843998241381322,1.20660898072922,6.36937689613002));
#67590=CARTESIAN_POINT('Ctrl Pts',(0.943152121354761,-1.9848822566212,6.17131345052912));
#67591=CARTESIAN_POINT('Ctrl Pts',(1.04230600132819,-4.69344241962331,4.47174077189317));
#67592=CARTESIAN_POINT('Ctrl Pts',(1.12583682146316,-6.0132230713283,2.12339252898828));
#67593=CARTESIAN_POINT('Ctrl Pts',(1.17631634827365,-6.21864581157698,0.544924936804922));
#67594=CARTESIAN_POINT('Ctrl Pts',(1.19374458175965,-6.21872571138575,-2.61246114025351E-5));
#67595=CARTESIAN_POINT('Origin',(-15.9277445817596,0.,0.));
#67596=CARTESIAN_POINT('',(-1.55274458175964,-6.21895806039946,-0.000138248926431941));
#67597=CARTESIAN_POINT('',(-1.30625541824035,-6.2189953734855,0.000144753730515756));
#67598=CARTESIAN_POINT('',(-15.9277445817596,-6.21925,-5.19709976349859E-13));
#67599=CARTESIAN_POINT('Ctrl Pts',(-1.55274458175964,-6.21895806039946,
-0.000138248926431564));
#67600=CARTESIAN_POINT('Ctrl Pts',(-1.54190526892002,-6.21923430388303,
-0.339028765878233));
#67601=CARTESIAN_POINT('Ctrl Pts',(-1.49801466275593,-6.10897986203804,
-1.71108823079692));
#67602=CARTESIAN_POINT('Ctrl Pts',(-1.42107276326736,-5.11386949628186,
-3.98411925462125));
#67603=CARTESIAN_POINT('Ctrl Pts',(-1.32191888329392,-2.58725738181136,
-5.9439857587572));
#67604=CARTESIAN_POINT('Ctrl Pts',(-1.22276500332049,0.568846473464286,
-6.45765291337906));
#67605=CARTESIAN_POINT('Ctrl Pts',(-1.12361112334705,3.58654733901449,-5.40014311338634));
#67606=CARTESIAN_POINT('Ctrl Pts',(-1.02445724337361,5.73162457469774,-3.02875340606772));
#67607=CARTESIAN_POINT('Ctrl Pts',(-0.925303363400179,6.4821709235304,0.0795460758479203));
#67608=CARTESIAN_POINT('Ctrl Pts',(-0.826149483426742,5.65557497197356,
3.16849162795677));
#67609=CARTESIAN_POINT('Ctrl Pts',(-0.726995603453303,3.45295135521813,
5.4865284468909));
#67610=CARTESIAN_POINT('Ctrl Pts',(-0.627841723479869,0.410208632109992,
6.46966740553085));
#67611=CARTESIAN_POINT('Ctrl Pts',(-0.528687843506432,-2.73233975692668,
5.87870622779908));
#67612=CARTESIAN_POINT('Ctrl Pts',(-0.429533963532995,-5.21009718927287,
3.85742851370921));
#67613=CARTESIAN_POINT('Ctrl Pts',(-0.354219542950729,-6.1292667586287,
1.60924393406421));
#67614=CARTESIAN_POINT('Ctrl Pts',(-0.31195641569294,-6.21937263065751,
0.288145397534895));
#67615=CARTESIAN_POINT('Ctrl Pts',(-0.30274458175963,-6.21909759658405,
0.000156462538848587));
#67616=CARTESIAN_POINT('Ctrl Pts',(-1.30625541824035,-6.2189953734855,0.000144753730515756));
#67617=CARTESIAN_POINT('Ctrl Pts',(-1.28358135818052,-6.21838497526395,
-0.708746276277476));
#67618=CARTESIAN_POINT('Ctrl Pts',(-1.2278560047962,-5.92090099563265,-2.4514656171939));
#67619=CARTESIAN_POINT('Ctrl Pts',(-1.1390793580874,-4.32539601471359,-4.82864542011847));
#67620=CARTESIAN_POINT('Ctrl Pts',(-1.03992547811397,-1.49100115648436,
-6.30886541532577));
#67621=CARTESIAN_POINT('Ctrl Pts',(-0.940771598140529,1.70616120997042,
-6.25410914542779));
#67622=CARTESIAN_POINT('Ctrl Pts',(-0.841617718167091,4.48820662760173,
-4.67769906527593));
#67623=CARTESIAN_POINT('Ctrl Pts',(-0.742463838193658,6.17825052154845,
-1.96318307101446));
#67624=CARTESIAN_POINT('Ctrl Pts',(-0.643309958220219,6.36509736085303,
1.22898448492769));
#67625=CARTESIAN_POINT('Ctrl Pts',(-0.544156078246782,5.00328644146473,
4.12213440610403));
#67626=CARTESIAN_POINT('Ctrl Pts',(-0.445002198273347,2.42415268673505,
6.01234987577457));
#67627=CARTESIAN_POINT('Ctrl Pts',(-0.34584831829991,-0.744788678740318,
6.43973268865655));
#67628=CARTESIAN_POINT('Ctrl Pts',(-0.246694438326474,-3.73251949855906,
5.3002986208522));
#67629=CARTESIAN_POINT('Ctrl Pts',(-0.150163471639955,-5.7570996405633,
2.93553207094277));
#67630=CARTESIAN_POINT('Ctrl Pts',(-0.0866837982779112,-6.21907088180063,
0.950935775860047));
#67631=CARTESIAN_POINT('Ctrl Pts',(-0.0562554182403475,-6.21969263819397,
-8.20542562896334E-5));
#67632=CARTESIAN_POINT('Origin',(-15.9277445817596,0.,0.));
#67633=CARTESIAN_POINT('',(-2.80274458175963,-6.21971960642536,6.88125055054123E-5));
#67634=CARTESIAN_POINT('',(-2.55625541824035,-6.21905581821482,-0.000152655409548785));
#67635=CARTESIAN_POINT('',(-15.9277445817596,-6.21925,-5.19709976349859E-13));
#67636=CARTESIAN_POINT('Ctrl Pts',(-2.80274458175963,-6.21971960642536,
6.88125055054584E-5));
#67637=CARTESIAN_POINT('Ctrl Pts',(-2.7718541221471,-6.21917464400886,-0.965378845559518));
#67638=CARTESIAN_POINT('Ctrl Pts',(-2.70791236921008,-5.74627529022682,
-2.96432394809749));
#67639=CARTESIAN_POINT('Ctrl Pts',(-2.61091932294859,-3.69549673468289,
-5.3261779301854));
#67640=CARTESIAN_POINT('Ctrl Pts',(-2.51176544297515,-0.699898932068888,
-6.4447660116512));
#67641=CARTESIAN_POINT('Ctrl Pts',(-2.41261156300172,2.46598753228901,-5.99531258156246));
#67642=CARTESIAN_POINT('Ctrl Pts',(-2.31345768302828,5.03188777362273,-4.0871717475183));
#67643=CARTESIAN_POINT('Ctrl Pts',(-2.21430380305485,6.37350634262576,-1.18460303923088));
#67644=CARTESIAN_POINT('Ctrl Pts',(-2.11514992308141,6.16442120860435,2.00618509189823));
#67645=CARTESIAN_POINT('Ctrl Pts',(-2.01599604310798,4.45550375602798,4.708859069888));
#67646=CARTESIAN_POINT('Ctrl Pts',(-1.91684216313454,1.66254154035103,6.26584575988373));
#67647=CARTESIAN_POINT('Ctrl Pts',(-1.8176882831611,-1.53492475588388,6.29832306680283));
#67648=CARTESIAN_POINT('Ctrl Pts',(-1.71853440318767,-4.35893672810028,
4.79838911098967));
#67649=CARTESIAN_POINT('Ctrl Pts',(-1.63021983605385,-5.929620799522,2.42258033937297));
#67650=CARTESIAN_POINT('Ctrl Pts',(-1.5749565622445,-6.21839198070816,0.694318093502356));
#67651=CARTESIAN_POINT('Ctrl Pts',(-1.55274458175964,-6.21895806039946,
-0.000138248926431564));
#67652=CARTESIAN_POINT('Ctrl Pts',(-2.55625541824035,-6.21905581821482,
-0.000152655409548716));
#67653=CARTESIAN_POINT('Ctrl Pts',(-2.54658150473207,-6.21933458755579,
-0.302593383880689));
#67654=CARTESIAN_POINT('Ctrl Pts',(-2.50385629789931,-6.12364022690166,
-1.63815947675647));
#67655=CARTESIAN_POINT('Ctrl Pts',(-2.42807979774207,-5.18309236738467,
-3.8936385025436));
#67656=CARTESIAN_POINT('Ctrl Pts',(-2.32892591776863,-2.69131095073478,
-5.89760227921367));
#67657=CARTESIAN_POINT('Ctrl Pts',(-2.2297720377952,0.455278923448612,-6.46665202242975));
#67658=CARTESIAN_POINT('Ctrl Pts',(-2.13061815782176,3.49109732043444,-5.4623352859914));
#67659=CARTESIAN_POINT('Ctrl Pts',(-2.03146427784832,5.67751552051297,-3.12900699770163));
#67660=CARTESIAN_POINT('Ctrl Pts',(-1.93231039787489,6.48256781800243,-0.0343767702148776));
#67661=CARTESIAN_POINT('Ctrl Pts',(-1.83315651790145,5.71038124883349,3.06861748517184));
#67662=CARTESIAN_POINT('Ctrl Pts',(-1.73400263792802,3.54883239268839,5.42500285031601));
#67663=CARTESIAN_POINT('Ctrl Pts',(-1.63484875795458,0.523836128332554,
6.46145981864663));
#67664=CARTESIAN_POINT('Ctrl Pts',(-1.53569487798115,-2.62861189967033,
5.92581359462503));
#67665=CARTESIAN_POINT('Ctrl Pts',(-1.43654099800771,-5.14150644054926,
3.94838939304646));
#67666=CARTESIAN_POINT('Ctrl Pts',(-1.36006117809411,-6.11487336731535,
1.68217183221436));
#67667=CARTESIAN_POINT('Ctrl Pts',(-1.31663265150499,-6.21927473433717,
0.324582792537371));
#67668=CARTESIAN_POINT('Ctrl Pts',(-1.30625541824035,-6.2189953734855,0.000144753730515756));
#67669=CARTESIAN_POINT('Origin',(-15.9277445817596,0.,0.));
#67670=CARTESIAN_POINT('',(-4.05274458175964,-6.21873391926796,3.92816190650305E-5));
#67671=CARTESIAN_POINT('',(-3.80625541824035,-6.21964459475637,0.000100671161871041));
#67672=CARTESIAN_POINT('',(-15.9277445817596,-6.21925,-5.19709976349859E-13));
#67673=CARTESIAN_POINT('Ctrl Pts',(-4.05274458175964,-6.21873391926796,
3.92816190651624E-5));
#67674=CARTESIAN_POINT('Ctrl Pts',(-4.03485426869866,-6.21861039758982,
-0.559358110548367));
#67675=CARTESIAN_POINT('Ctrl Pts',(-3.9839126623132,-6.00567259807345,-2.15230124746295));
#67676=CARTESIAN_POINT('Ctrl Pts',(-3.89991976260326,-4.66216967103227,
-4.50433584655415));
#67677=CARTESIAN_POINT('Ctrl Pts',(-3.80076588262983,-1.94183273665795,
-6.18499418616455));
#67678=CARTESIAN_POINT('Ctrl Pts',(-3.70161200265638,1.25096112385931,-6.36081470620222));
#67679=CARTESIAN_POINT('Ctrl Pts',(-3.60245812268296,4.13939033126021,-4.98901945731978));
#67680=CARTESIAN_POINT('Ctrl Pts',(-3.50330424270952,6.02068664039774,-2.40337259661961));
#67681=CARTESIAN_POINT('Ctrl Pts',(-3.40415036273608,6.43712191918314,0.767025982361597));
#67682=CARTESIAN_POINT('Ctrl Pts',(-3.30499648276265,5.28737552962418,3.75080357640562));
#67683=CARTESIAN_POINT('Ctrl Pts',(-3.20584260278921,2.85118610976127,5.82199323492824));
#67684=CARTESIAN_POINT('Ctrl Pts',(-3.10668872281577,-0.278710136569954,
6.47666489173394));
#67685=CARTESIAN_POINT('Ctrl Pts',(-3.00753484284234,-3.34079491184971,
5.55553389126599));
#67686=CARTESIAN_POINT('Ctrl Pts',(-2.9083809628689,-5.59004876450166,3.28271568530374));
#67687=CARTESIAN_POINT('Ctrl Pts',(-2.840117542508,-6.20220553006854,1.16810013092565));
#67688=CARTESIAN_POINT('Ctrl Pts',(-2.80490541547158,-6.21975772735901,
0.0676033158062671));
#67689=CARTESIAN_POINT('Ctrl Pts',(-2.80274458175963,-6.21971960642536,
6.88125055054584E-5));
#67690=CARTESIAN_POINT('Ctrl Pts',(-3.80625541824035,-6.21964459475637,
0.000100671161871058));
#67691=CARTESIAN_POINT('Ctrl Pts',(-3.77653035795915,-6.21892929456546,
-0.928956203119842));
#67692=CARTESIAN_POINT('Ctrl Pts',(-3.71375400435347,-5.77334154366877,
-2.89169444538626));
#67693=CARTESIAN_POINT('Ctrl Pts',(-3.6179263574233,-3.78852249476445,-5.26041486804939));
#67694=CARTESIAN_POINT('Ctrl Pts',(-3.51877247744987,-0.813044105235338,
-6.43147157035411));
#67695=CARTESIAN_POINT('Ctrl Pts',(-3.41961859747643,2.36025169231589,-6.03772136043487));
#67696=CARTESIAN_POINT('Ctrl Pts',(-3.32046471750299,4.95928728793312,-4.17496549363898));
#67697=CARTESIAN_POINT('Ctrl Pts',(-3.22131083752956,6.35170524667332,-1.29642112629886));
#67698=CARTESIAN_POINT('Ctrl Pts',(-3.12215695755612,6.19872381031724,1.89754852394804));
#67699=CARTESIAN_POINT('Ctrl Pts',(-3.02300307758268,4.53756407304736,4.62983580273871));
#67700=CARTESIAN_POINT('Ctrl Pts',(-2.92384919760925,1.77239391631247,6.23566252155694));
#67701=CARTESIAN_POINT('Ctrl Pts',(-2.82469531763581,-1.42400791440103,
6.32432357940788));
#67702=CARTESIAN_POINT('Ctrl Pts',(-2.72554143766238,-4.27394200392325,
4.87424732901725));
#67703=CARTESIAN_POINT('Ctrl Pts',(-2.63606147119722,-5.90740787501663,
2.49542479295947));
#67704=CARTESIAN_POINT('Ctrl Pts',(-2.57963279805655,-6.21838216150297,
0.730706864401547));
#67705=CARTESIAN_POINT('Ctrl Pts',(-2.55625541824035,-6.21905581821482,
-0.000152655409548716));
#67706=CARTESIAN_POINT('Origin',(-15.9277445817596,0.,0.));
#67707=CARTESIAN_POINT('',(-5.30274458175963,-6.2195145656829,-0.000134032925609376));
#67708=CARTESIAN_POINT('',(-5.05625541824036,-6.21871962902234,5.79115600640723E-6));
#67709=CARTESIAN_POINT('',(-15.9277445817596,-6.21925,-5.19709976349859E-13));
#67710=CARTESIAN_POINT('Ctrl Pts',(-5.30274458175963,-6.2195145656829,-0.000134032925609619));
#67711=CARTESIAN_POINT('Ctrl Pts',(-5.29785441525021,-6.21965942650832,
-0.152985454681894));
#67712=CARTESIAN_POINT('Ctrl Pts',(-5.25991295541631,-6.17682437695265,
-1.3388366666538));
#67713=CARTESIAN_POINT('Ctrl Pts',(-5.18892020225794,-5.45024505989854,
-3.50994248487028));
#67714=CARTESIAN_POINT('Ctrl Pts',(-5.08976632228449,-3.10937916608465,
-5.68828872874475));
#67715=CARTESIAN_POINT('Ctrl Pts',(-4.99061244231106,-0.0119868756926444,
-6.48264789841751));
#67716=CARTESIAN_POINT('Ctrl Pts',(-4.89145856233762,3.08832187724368,-5.69974871749482));
#67717=CARTESIAN_POINT('Ctrl Pts',(-4.79230468236419,5.43722756980429,-3.53007419386704));
#67718=CARTESIAN_POINT('Ctrl Pts',(-4.69315080239075,6.46323053450655,-0.501516218948075));
#67719=CARTESIAN_POINT('Ctrl Pts',(-4.59399692241732,5.91669948346157,2.64906298197146));
#67720=CARTESIAN_POINT('Ctrl Pts',(-4.49484304244388,3.93060796044775,5.15511285243209));
#67721=CARTESIAN_POINT('Ctrl Pts',(-4.39568916247044,0.988181259944745,
6.40689981641197));
#67722=CARTESIAN_POINT('Ctrl Pts',(-4.29653528249701,-2.19467453196863,
6.09985829005677));
#67723=CARTESIAN_POINT('Ctrl Pts',(-4.19738140252357,-4.84355581429439,
4.30869290317386));
#67724=CARTESIAN_POINT('Ctrl Pts',(-4.11611783561112,-6.04866960539269,
1.98153115056918));
#67725=CARTESIAN_POINT('Ctrl Pts',(-4.06790556202314,-6.21883859657115,
0.474095425477252));
#67726=CARTESIAN_POINT('Ctrl Pts',(-4.05274458175964,-6.21873391926796,
3.92816190651624E-5));
#67727=CARTESIAN_POINT('Ctrl Pts',(-5.05625541824036,-6.21871962902234,
5.79115600630314E-6));
#67728=CARTESIAN_POINT('Ctrl Pts',(-5.03953050451071,-6.21870265207545,
-0.522955127194714));
#67729=CARTESIAN_POINT('Ctrl Pts',(-4.98975429745658,-6.02450268975374,
-2.07938874875887));
#67730=CARTESIAN_POINT('Ctrl Pts',(-4.90692679707797,-4.74060400838073,
-4.42171244124443));
#67731=CARTESIAN_POINT('Ctrl Pts',(-4.80777291710454,-2.05022118826812,
-6.14991547555801));
#67732=CARTESIAN_POINT('Ctrl Pts',(-4.7086190371311,1.13898997181236,-6.38181550355714));
#67733=CARTESIAN_POINT('Ctrl Pts',(-4.60946515715766,4.05107958026204,-5.06099017107475));
#67734=CARTESIAN_POINT('Ctrl Pts',(-4.51031127718423,5.9775227064379,-2.50880241775846));
#67735=CARTESIAN_POINT('Ctrl Pts',(-4.41115739721079,6.44960678792389,0.653788619124958));
#67736=CARTESIAN_POINT('Ctrl Pts',(-4.31200351723735,5.35247157449903,3.65730984762178));
#67737=CARTESIAN_POINT('Ctrl Pts',(-4.21284963726392,2.9530551606307,5.77099059916091));
#67738=CARTESIAN_POINT('Ctrl Pts',(-4.11369575729048,-0.164853293042968,
6.48056252721199));
#67739=CARTESIAN_POINT('Ctrl Pts',(-4.01454187731705,-3.24265217464831,
5.61338348517005));
#67740=CARTESIAN_POINT('Ctrl Pts',(-3.91538799734361,-5.53149871753584,
3.3804421626809));
#67741=CARTESIAN_POINT('Ctrl Pts',(-3.84595917765138,-6.19180447005486,
1.24099882977293));
#67742=CARTESIAN_POINT('Ctrl Pts',(-3.80958165128363,-6.2197246368188,0.104062097819437));
#67743=CARTESIAN_POINT('Ctrl Pts',(-3.80625541824035,-6.21964459475637,
0.000100671161871058));
#67744=CARTESIAN_POINT('Origin',(-15.9277445817596,0.,0.));
#67745=CARTESIAN_POINT('',(-6.55274458175964,-6.21920212302629,0.000160857331407452));
#67746=CARTESIAN_POINT('',(-6.30625541824035,-6.21961412857971,-0.000110289616846448));
#67747=CARTESIAN_POINT('',(-15.9277445817596,-6.21925,-5.19709976349859E-13));
#67748=CARTESIAN_POINT('Ctrl Pts',(-6.55274458175964,-6.21920212302629,
0.000160857331407242));
#67749=CARTESIAN_POINT('Ctrl Pts',(-6.52780326847729,-6.21841381317065,
-0.779540053029137));
#67750=CARTESIAN_POINT('Ctrl Pts',(-6.46981066187046,-5.87644188319325,
-2.59314334766061));
#67751=CARTESIAN_POINT('Ctrl Pts',(-6.37876676193917,-4.1578120641639,-4.97367734167979));
#67752=CARTESIAN_POINT('Ctrl Pts',(-6.27961288196573,-1.27447568419159,
-6.3561449944483));
#67753=CARTESIAN_POINT('Ctrl Pts',(-6.18045900199229,1.91894655066922,-6.19213304086084));
#67754=CARTESIAN_POINT('Ctrl Pts',(-6.08130512201886,4.64548017476219,-4.52154635118754));
#67755=CARTESIAN_POINT('Ctrl Pts',(-5.98215124204542,6.24174689048921,-1.75084642819241));
#67756=CARTESIAN_POINT('Ctrl Pts',(-5.88299736207198,6.31936759002112,1.44584256481697));
#67757=CARTESIAN_POINT('Ctrl Pts',(-5.78384348209855,4.85945679655365,4.29075134475004));
#67758=CARTESIAN_POINT('Ctrl Pts',(-5.68468960212512,2.21721758855159,6.09170038864876));
#67759=CARTESIAN_POINT('Ctrl Pts',(-5.58553572215167,-0.964480959434654,
6.41051042733211));
#67760=CARTESIAN_POINT('Ctrl Pts',(-5.48638184217824,-3.91151680923086,
5.16961349726944));
#67761=CARTESIAN_POINT('Ctrl Pts',(-5.39211812871423,-5.80845407019422,
2.7941582823786));
#67762=CARTESIAN_POINT('Ctrl Pts',(-5.33090570857469,-6.21868035194655,
0.880095354692622));
#67763=CARTESIAN_POINT('Ctrl Pts',(-5.30274458175963,-6.2195145656829,-0.000134032925609619));
#67764=CARTESIAN_POINT('Ctrl Pts',(-6.30625541824035,-6.21961412857971,
-0.000110289616846275));
#67765=CARTESIAN_POINT('Ctrl Pts',(-6.30253065106226,-6.21971023156661,
-0.116529554341081));
#67766=CARTESIAN_POINT('Ctrl Pts',(-6.26575459055969,-6.18809861508296,
-1.26592961559787));
#67767=CARTESIAN_POINT('Ctrl Pts',(-6.19592723673265,-5.51108332618975,
-3.41362385876426));
#67768=CARTESIAN_POINT('Ctrl Pts',(-6.0967733567592,-3.20885877105538,-5.63276953769212));
#67769=CARTESIAN_POINT('Ctrl Pts',(-5.99761947678577,-0.125903969293837,
-6.48143621953093));
#67770=CARTESIAN_POINT('Ctrl Pts',(-5.89846559681233,2.98768385311816,-5.75313935787656));
#67771=CARTESIAN_POINT('Ctrl Pts',(-5.7993117168389,5.37435431396556,-3.62507696267142));
#67772=CARTESIAN_POINT('Ctrl Pts',(-5.70015783686546,6.45341940219507,-0.615016501163695));
#67773=CARTESIAN_POINT('Ctrl Pts',(-5.60100395689203,5.96233756874898,2.5446803323042));
#67774=CARTESIAN_POINT('Ctrl Pts',(-5.50185007691858,4.02059130515946,5.08524461891535));
#67775=CARTESIAN_POINT('Ctrl Pts',(-5.40269619694516,1.10061649827017,6.38854526485231));
#67776=CARTESIAN_POINT('Ctrl Pts',(-5.30354231697171,-2.08714341586264,
6.1374831681197));
#67777=CARTESIAN_POINT('Ctrl Pts',(-5.20438843699829,-4.76709164052158,
4.39314290323005));
#67778=CARTESIAN_POINT('Ctrl Pts',(-5.12195947075449,-6.03078064977054,
2.0544529265738));
#67779=CARTESIAN_POINT('Ctrl Pts',(-5.07258179783519,-6.21873620142945,
0.510505193680209));
#67780=CARTESIAN_POINT('Ctrl Pts',(-5.05625541824036,-6.21871962902234,
5.79115600630314E-6));
#67781=CARTESIAN_POINT('Origin',(-15.9277445817596,0.,0.));
#67782=CARTESIAN_POINT('',(-7.80274458175964,-6.21887801778165,-0.000118905825011546));
#67783=CARTESIAN_POINT('',(-7.55625541824036,-6.21909175420816,0.000156006089798849));
#67784=CARTESIAN_POINT('',(-15.9277445817596,-6.21925,-5.19709976349859E-13));
#67785=CARTESIAN_POINT('Ctrl Pts',(-7.80274458175964,-6.21887801778165,
-0.000118905825011589));
#67786=CARTESIAN_POINT('Ctrl Pts',(-7.79080341502885,-6.21913509997953,
-0.373472596954706));
#67787=CARTESIAN_POINT('Ctrl Pts',(-7.74581095497358,-6.09449665494633,
-1.7800416268261));
#67788=CARTESIAN_POINT('Ctrl Pts',(-7.66776720159383,-5.0469682541968,-4.06853522796294));
#67789=CARTESIAN_POINT('Ctrl Pts',(-7.5686133216204,-2.48814211006943,-5.98615204452285));
#67790=CARTESIAN_POINT('Ctrl Pts',(-7.46945944164697,0.676060568781244,
-6.44731025834689));
#67791=CARTESIAN_POINT('Ctrl Pts',(-7.37030556167352,3.6757745704235,-5.3398079335753));
#67792=CARTESIAN_POINT('Ctrl Pts',(-7.2711516817001,5.78115554226751,-2.93310553102942));
#67793=CARTESIAN_POINT('Ctrl Pts',(-7.17199780172665,6.47995451274163,0.187235073758361));
#67794=CARTESIAN_POINT('Ctrl Pts',(-7.07284392175322,5.60215044586807,3.26202051524908));
#67795=CARTESIAN_POINT('Ctrl Pts',(-6.97369004177978,3.36131714919565,5.54314121077292));
#67796=CARTESIAN_POINT('Ctrl Pts',(-6.87453616180634,0.302659774207504,
6.47558989754003));
#67797=CARTESIAN_POINT('Ctrl Pts',(-6.77538228183291,-2.82963612993394,
5.83249747811505));
#67798=CARTESIAN_POINT('Ctrl Pts',(-6.67622840185946,-5.27346841781536,
3.77033132580544));
#67799=CARTESIAN_POINT('Ctrl Pts',(-6.60201583516839,-6.14225880651794,
1.54029520057943));
#67800=CARTESIAN_POINT('Ctrl Pts',(-6.56085456180177,-6.219458451838,0.253690362785901));
#67801=CARTESIAN_POINT('Ctrl Pts',(-6.55274458175964,-6.21920212302629,
0.000160857331407242));
#67802=CARTESIAN_POINT('Ctrl Pts',(-7.55625541824035,-6.21909175420816,
0.00015600608979878));
#67803=CARTESIAN_POINT('Ctrl Pts',(-7.53247950428934,-6.21838504441926,
-0.743150766835367));
#67804=CARTESIAN_POINT('Ctrl Pts',(-7.47565229701384,-5.89964322201078,
-2.52033047309439));
#67805=CARTESIAN_POINT('Ctrl Pts',(-7.38577379641388,-4.2445719758881,-4.89984448925031));
#67806=CARTESIAN_POINT('Ctrl Pts',(-7.28661991644044,-1.38597480405236,
-6.33276725609456));
#67807=CARTESIAN_POINT('Ctrl Pts',(-7.187466036467,1.80983647653362,-6.22489832893194));
#67808=CARTESIAN_POINT('Ctrl Pts',(-7.08831215649357,4.56530613428956,-4.6024827188757));
#67809=CARTESIAN_POINT('Ctrl Pts',(-6.98915827652013,6.21001560019695,-1.86026168122711));
#67810=CARTESIAN_POINT('Ctrl Pts',(-6.89000439654669,6.34379942025369,1.3345696658175));
#67811=CARTESIAN_POINT('Ctrl Pts',(-6.79085051657326,4.93410736951075,4.204694013061));
#67812=CARTESIAN_POINT('Ctrl Pts',(-6.69169663659982,2.3239240730231,6.05179677287292));
#67813=CARTESIAN_POINT('Ctrl Pts',(-6.59254275662638,-0.851680746854733,
6.42646926257087));
#67814=CARTESIAN_POINT('Ctrl Pts',(-6.49338887665295,-3.8200676843074,5.23755192476806));
#67815=CARTESIAN_POINT('Ctrl Pts',(-6.39795976385761,-5.78242031070725,
2.86684669246173));
#67816=CARTESIAN_POINT('Ctrl Pts',(-6.33558194438674,-6.21885747276121,
0.916503406659185));
#67817=CARTESIAN_POINT('Ctrl Pts',(-6.30625541824035,-6.21961412857971,
-0.000110289616846275));
#67818=CARTESIAN_POINT('Origin',(-15.9277445817596,0.,0.));
#67819=CARTESIAN_POINT('',(-9.05274458175964,-6.21976606909926,3.47298191171853E-5));
#67820=CARTESIAN_POINT('',(-8.80625541824036,-6.21896305789945,-0.000139202748639933));
#67821=CARTESIAN_POINT('',(-15.9277445817596,-6.21925,-5.19709976349859E-13));
#67822=CARTESIAN_POINT('Ctrl Pts',(-9.05274458175964,-6.21976606909926,
3.47298191171689E-5));
#67823=CARTESIAN_POINT('Ctrl Pts',(-9.02075226825592,-6.21945831059647,
-0.999828447687547));
#67824=CARTESIAN_POINT('Ctrl Pts',(-8.95570866142774,-5.71997014190296,
-3.03294779101907));
#67825=CARTESIAN_POINT('Ctrl Pts',(-8.85761376127506,-3.60649324070849,
-5.38684267124721));
#67826=CARTESIAN_POINT('Ctrl Pts',(-8.75845988130164,-0.592723818367459,
-6.45550508753466));
#67827=CARTESIAN_POINT('Ctrl Pts',(-8.65930600132819,2.56525806264267,-5.95351312521376));
#67828=CARTESIAN_POINT('Ctrl Pts',(-8.56015212135476,5.09910073940523,-4.00300376085795));
#67829=CARTESIAN_POINT('Ctrl Pts',(-8.46099824138133,6.39230851700605,-1.07854498443864));
#67830=CARTESIAN_POINT('Ctrl Pts',(-8.36184436140788,6.13023793520507,2.10832879736973));
#67831=CARTESIAN_POINT('Ctrl Pts',(-8.26269048143445,4.37665198407491,4.78223638796107));
#67832=CARTESIAN_POINT('Ctrl Pts',(-8.16353660146101,1.55820627228779,6.29260364817686));
#67833=CARTESIAN_POINT('Ctrl Pts',(-8.06438272148758,-1.63935826461956,
6.27195120678321));
#67834=CARTESIAN_POINT('Ctrl Pts',(-7.96522884151414,-4.43805931965865,
4.72530389871772));
#67835=CARTESIAN_POINT('Ctrl Pts',(-7.87801612827149,-5.94995159800372,
2.35368967431146));
#67836=CARTESIAN_POINT('Ctrl Pts',(-7.82385470835333,-6.21842353641775,
0.659912384387782));
#67837=CARTESIAN_POINT('Ctrl Pts',(-7.80274458175964,-6.21887801778165,
-0.000118905825011589));
#67838=CARTESIAN_POINT('Ctrl Pts',(-8.80625541824036,-6.21896305789945,
-0.000139202748640176));
#67839=CARTESIAN_POINT('Ctrl Pts',(-8.7954796508409,-6.21923989921398,-0.337042195846759));
#67840=CARTESIAN_POINT('Ctrl Pts',(-8.75165259011697,-6.10979663044418,
-1.707111614424));
#67841=CARTESIAN_POINT('Ctrl Pts',(-8.67477423606854,-5.11768488976202,
-3.97921708963369));
#67842=CARTESIAN_POINT('Ctrl Pts',(-8.57562035609511,-2.5929519681933,-5.94150379684923));
#67843=CARTESIAN_POINT('Ctrl Pts',(-8.47646647612167,0.56265821350308,-6.45819502741354));
#67844=CARTESIAN_POINT('Ctrl Pts',(-8.37731259614824,3.58137103787181,-5.40357740450012));
#67845=CARTESIAN_POINT('Ctrl Pts',(-8.2781587161748,5.72871965048953,-3.0342442952779));
#67846=CARTESIAN_POINT('Ctrl Pts',(-8.17900483620137,6.48224415781214,0.0733345473956177));
#67847=CARTESIAN_POINT('Ctrl Pts',(-8.07985095622792,5.65860854650426,3.16307075399211));
#67848=CARTESIAN_POINT('Ctrl Pts',(-7.98069707625449,3.45820718722118,5.48321715123368));
#67849=CARTESIAN_POINT('Ctrl Pts',(-7.88154319628105,0.416407953241648,
6.46927134179796));
#67850=CARTESIAN_POINT('Ctrl Pts',(-7.78238931630763,-2.72670527029838,
5.88132176013677));
#67851=CARTESIAN_POINT('Ctrl Pts',(-7.68323543633418,-5.20639843392111,
3.86241927094858));
#67852=CARTESIAN_POINT('Ctrl Pts',(-7.60785747031176,-6.12849923849585,
1.61322038691257));
#67853=CARTESIAN_POINT('Ctrl Pts',(-7.56553079761382,-6.21936745344784,
0.290132337765249));
#67854=CARTESIAN_POINT('Ctrl Pts',(-7.55625541824035,-6.21909175420816,
0.00015600608979878));
#67855=CARTESIAN_POINT('Origin',(-15.9277445817596,0.,0.));
#67856=CARTESIAN_POINT('',(-10.3027445817596,-6.21876660816596,6.94236083599781E-5));
#67857=CARTESIAN_POINT('',(-10.0562554182404,-6.21971612434898,7.06762300196201E-5));
#67858=CARTESIAN_POINT('',(-15.9277445817596,-6.21925,-5.19709976349859E-13));
#67859=CARTESIAN_POINT('Ctrl Pts',(-10.3027445817596,-6.21876660816596,
6.94236083600974E-5));
#67860=CARTESIAN_POINT('Ctrl Pts',(-10.2837524148075,-6.21853335738712,
-0.593771994205459));
#67861=CARTESIAN_POINT('Ctrl Pts',(-10.2317089545308,-5.98721839491704,
-2.22122932514984));
#67862=CARTESIAN_POINT('Ctrl Pts',(-10.1466142009297,-4.58668748447852,
-4.58117510904947));
#67863=CARTESIAN_POINT('Ctrl Pts',(-10.0474603209563,-1.83880224932734,
-6.21640360239859));
#67864=CARTESIAN_POINT('Ctrl Pts',(-9.94830644098286,1.35647211574301,-6.33915221928435));
#67865=CARTESIAN_POINT('Ctrl Pts',(-9.84915256100943,4.22171051319157,-4.91955565095604));
#67866=CARTESIAN_POINT('Ctrl Pts',(-9.749998681036,6.05978712967198,-2.30300833761142));
#67867=CARTESIAN_POINT('Ctrl Pts',(-9.65084480106255,6.42348938510785,0.873871603528));
#67868=CARTESIAN_POINT('Ctrl Pts',(-9.55169092108912,5.22432683107353,3.83813452371996));
#67869=CARTESIAN_POINT('Ctrl Pts',(-9.45253704111568,2.75406128800256,5.86856148318917));
#67870=CARTESIAN_POINT('Ctrl Pts',(-9.35338316114225,-0.386280161182942,
6.47114016979406));
#67871=CARTESIAN_POINT('Ctrl Pts',(-9.25422928116881,-3.43263785258272,
5.49926038963988));
#67872=CARTESIAN_POINT('Ctrl Pts',(-9.15507540119538,-5.6438188071929,3.18938500837096));
#67873=CARTESIAN_POINT('Ctrl Pts',(-9.08791383472565,-6.2114446770495,1.09918238554259));
#67874=CARTESIAN_POINT('Ctrl Pts',(-9.0538035615804,-6.21977625623512,0.0331312712238126));
#67875=CARTESIAN_POINT('Ctrl Pts',(-9.05274458175964,-6.21976606909926,
3.47298191171689E-5));
#67876=CARTESIAN_POINT('Ctrl Pts',(-10.0562554182404,-6.21971612434898,
7.06762300198109E-5));
#67877=CARTESIAN_POINT('Ctrl Pts',(-10.025428504068,-6.21915984463267,-0.963392497100496));
#67878=CARTESIAN_POINT('Ctrl Pts',(-9.96155029657112,-5.74777108715391,
-2.96036492166516));
#67879=CARTESIAN_POINT('Ctrl Pts',(-9.86462079574977,-3.70059880012039,
-5.32263429120195));
#67880=CARTESIAN_POINT('Ctrl Pts',(-9.76546691577635,-0.706074257995519,
-6.44409236584388));
#67881=CARTESIAN_POINT('Ctrl Pts',(-9.66631303580289,2.46024143136038,-5.99767283008577));
#67882=CARTESIAN_POINT('Ctrl Pts',(-9.56715915582948,5.02796895074312,-4.0919916309414));
#67883=CARTESIAN_POINT('Ctrl Pts',(-9.46800527585603,6.37236826560774,-1.1907098575248));
#67884=CARTESIAN_POINT('Ctrl Pts',(-9.36885139588261,6.16634077687366,2.00027715599528));
#67885=CARTESIAN_POINT('Ctrl Pts',(-9.26969751590915,4.4600139297068,4.70458744462813));
#67886=CARTESIAN_POINT('Ctrl Pts',(-9.17054363593573,1.66854497323006,6.2642497515377));
#67887=CARTESIAN_POINT('Ctrl Pts',(-9.07138975596228,-1.52888872691469,
6.29979099161586));
#67888=CARTESIAN_POINT('Ctrl Pts',(-8.97223587598886,-4.35433669693118,
4.80256381603513));
#67889=CARTESIAN_POINT('Ctrl Pts',(-8.88385776341487,-5.92842844484179,
2.42655284231093));
#67890=CARTESIAN_POINT('Ctrl Pts',(-8.82853094416538,-6.21839077514218,
0.696302273646909));
#67891=CARTESIAN_POINT('Ctrl Pts',(-8.80625541824036,-6.21896305789945,
-0.000139202748640176));
#67892=CARTESIAN_POINT('Origin',(-15.9277445817596,0.,0.));
#67893=CARTESIAN_POINT('',(-11.5527445817596,-6.21941055513622,-0.000149866139592504));
#67894=CARTESIAN_POINT('',(-11.3062554182404,-6.21873258297641,3.7485977482099E-5));
#67895=CARTESIAN_POINT('',(-15.9277445817596,-6.21925,-5.19709976349859E-13));
#67896=CARTESIAN_POINT('Ctrl Pts',(-11.5527445817596,-6.21941055513622,
-0.000149866139592288));
#67897=CARTESIAN_POINT('Ctrl Pts',(-11.546752561359,-6.21960006073928,-0.187450862764453));
#67898=CARTESIAN_POINT('Ctrl Pts',(-11.507709247634,-6.16556255002488,-1.40777360244643));
#67899=CARTESIAN_POINT('Ctrl Pts',(-11.4356146405844,-5.39117573865922,
-3.60001272395876));
#67900=CARTESIAN_POINT('Ctrl Pts',(-11.336460760611,-3.01444017827433,-5.73916525930964));
#67901=CARTESIAN_POINT('Ctrl Pts',(-11.2373068806375,0.0957226818348403,
-6.48195222344366));
#67902=CARTESIAN_POINT('Ctrl Pts',(-11.1381530006641,3.18259576877592,-5.64765009833173));
#67903=CARTESIAN_POINT('Ctrl Pts',(-11.0389991206906,5.49512851954185,-3.43924846639081));
#67904=CARTESIAN_POINT('Ctrl Pts',(-10.9398452407172,6.47067097239111,-0.394061704715005));
#67905=CARTESIAN_POINT('Ctrl Pts',(-10.8406913607438,5.87186911638537,2.7470021004937));
#67906=CARTESIAN_POINT('Ctrl Pts',(-10.7415374807704,3.84441422499412,5.219707532676));
#67907=CARTESIAN_POINT('Ctrl Pts',(-10.6423836007969,0.881595492385054,
6.42243387259649));
#67908=CARTESIAN_POINT('Ctrl Pts',(-10.5432297208235,-2.29571951921329,
6.062552214137));
#67909=CARTESIAN_POINT('Ctrl Pts',(-10.44407584085,-4.9144753063956,4.22762343674055));
#67910=CARTESIAN_POINT('Ctrl Pts',(-10.3639141278288,-6.06494378424448,
1.91258134226202));
#67911=CARTESIAN_POINT('Ctrl Pts',(-10.316803708132,-6.21893927420161,0.439665998301346));
#67912=CARTESIAN_POINT('Ctrl Pts',(-10.3027445817596,-6.21876660816596,
6.94236083600974E-5));
#67913=CARTESIAN_POINT('Ctrl Pts',(-11.3062554182404,-6.21873258297641,
3.74859774820643E-5));
#67914=CARTESIAN_POINT('Ctrl Pts',(-11.2884286506195,-6.21861515675503,
-0.557373294400618));
#67915=CARTESIAN_POINT('Ctrl Pts',(-11.2375505896742,-6.00671752297004,
-2.14832578591357));
#67916=CARTESIAN_POINT('Ctrl Pts',(-11.1536212354044,-4.66648376653058,
-4.49986627956914));
#67917=CARTESIAN_POINT('Ctrl Pts',(-11.054467355431,-1.94775856528816,-6.18313058641824));
#67918=CARTESIAN_POINT('Ctrl Pts',(-10.9553134754576,1.24486534373372,-6.36201049616318));
#67919=CARTESIAN_POINT('Ctrl Pts',(-10.8561595954841,4.13460773126303,-4.99298369573902));
#67920=CARTESIAN_POINT('Ctrl Pts',(-10.7570057155107,6.01838084932733,-2.40914076587077));
#67921=CARTESIAN_POINT('Ctrl Pts',(-10.6578518355373,6.43785394671903,0.760857304653864));
#67922=CARTESIAN_POINT('Ctrl Pts',(-10.5586979555638,5.2909672700661,3.74573525818645));
#67923=CARTESIAN_POINT('Ctrl Pts',(-10.4595440755904,2.85676367597327,5.81925842156633));
#67924=CARTESIAN_POINT('Ctrl Pts',(-10.360390195617,-0.272503792359383,
6.4769289760257));
#67925=CARTESIAN_POINT('Ctrl Pts',(-10.2612363156435,-3.33546982202023,
5.55873262027628));
#67926=CARTESIAN_POINT('Ctrl Pts',(-10.1620824356701,-5.58690054814797,
3.28807079340383));
#67927=CARTESIAN_POINT('Ctrl Pts',(-10.093755469869,-6.20165507982626,1.17207489074341));
#67928=CARTESIAN_POINT('Ctrl Pts',(-10.0584797973925,-6.21975626385165,
0.0695913355015432));
#67929=CARTESIAN_POINT('Ctrl Pts',(-10.0562554182404,-6.21971612434898,
7.06762300198109E-5));
#67930=CARTESIAN_POINT('Origin',(-15.9277445817596,0.,0.));
#67931=CARTESIAN_POINT('',(-12.8027445817596,-6.21931067987726,0.000159553896288647));
#67932=CARTESIAN_POINT('',(-12.5562554182404,-6.21952031151783,-0.000132913339471741));
#67933=CARTESIAN_POINT('',(-15.9277445817596,-6.21925,-5.19709976349859E-13));
#67934=CARTESIAN_POINT('Ctrl Pts',(-12.8027445817596,-6.21931067987726,
0.000159553896288585));
#67935=CARTESIAN_POINT('Ctrl Pts',(-12.7767014145861,-6.21847181659383,
-0.813946089195492));
#67936=CARTESIAN_POINT('Ctrl Pts',(-12.7176069540881,-5.8538214760635,-2.66196229397221));
#67937=CARTESIAN_POINT('Ctrl Pts',(-12.6254612002656,-4.07460155155841,
-5.04207103051742));
#67938=CARTESIAN_POINT('Ctrl Pts',(-12.5263073202922,-1.16869364290732,
-6.37644329080494));
#67939=CARTESIAN_POINT('Ctrl Pts',(-12.4271534403188,2.02156270600836,-6.15939513026191));
#67940=CARTESIAN_POINT('Ctrl Pts',(-12.3279995603453,4.71996353557397,-4.4437386264808));
#67941=CARTESIAN_POINT('Ctrl Pts',(-12.2288456803719,6.26997526840712,-1.6468992987736));
#67942=CARTESIAN_POINT('Ctrl Pts',(-12.1296918003985,6.29447291053824,1.55063798442858));
#67943=CARTESIAN_POINT('Ctrl Pts',(-12.030537920425,4.78749604001144,4.37089799439875));
#67944=CARTESIAN_POINT('Ctrl Pts',(-11.9313840404516,2.11569914692158,6.12769813751704));
#67945=CARTESIAN_POINT('Ctrl Pts',(-11.8322301604782,-1.07085718055863,
6.39360089646495));
#67946=CARTESIAN_POINT('Ctrl Pts',(-11.7330762805047,-3.99686897955958,
5.10391083313569));
#67947=CARTESIAN_POINT('Ctrl Pts',(-11.6399144209319,-5.83236767530601,
2.72539768871601));
#67948=CARTESIAN_POINT('Ctrl Pts',(-11.5798038546835,-6.21855476969312,
0.845679828645856));
#67949=CARTESIAN_POINT('Ctrl Pts',(-11.5527445817596,-6.21941055513622,
-0.000149866139592288));
#67950=CARTESIAN_POINT('Ctrl Pts',(-12.5562554182404,-6.21952031151782,
-0.000132913339471047));
#67951=CARTESIAN_POINT('Ctrl Pts',(-12.5514287971711,-6.21966250851912,
-0.150997695672446));
#67952=CARTESIAN_POINT('Ctrl Pts',(-12.5135508827773,-6.17745595899215,
-1.33486110651861));
#67953=CARTESIAN_POINT('Ctrl Pts',(-12.4426216750591,-5.45360592369372,
-3.50471822801767));
#67954=CARTESIAN_POINT('Ctrl Pts',(-12.3434677950857,-3.11482849091286,
-5.68530655580378));
#67955=CARTESIAN_POINT('Ctrl Pts',(-12.2443139151122,-0.0181988194650487,
-6.4826334267188));
#67956=CARTESIAN_POINT('Ctrl Pts',(-12.1451600351388,3.08285871135025,-5.70270544700054));
#67957=CARTESIAN_POINT('Ctrl Pts',(-12.0460061551654,5.43384239437673,-3.5352827494326));
#67958=CARTESIAN_POINT('Ctrl Pts',(-11.9468522751919,6.46274697899828,-0.507709329187834));
#67959=CARTESIAN_POINT('Ctrl Pts',(-11.8476983952185,5.91923519889273,2.64339212664902));
#67960=CARTESIAN_POINT('Ctrl Pts',(-11.7485445152451,3.93554599561895,5.15134399897086));
#67961=CARTESIAN_POINT('Ctrl Pts',(-11.6493906352716,0.994320167882758,
6.4059499435945));
#67962=CARTESIAN_POINT('Ctrl Pts',(-11.5502367552982,-2.18882837604633,
6.10195850675201));
#67963=CARTESIAN_POINT('Ctrl Pts',(-11.4510828753248,-4.83942480730361,
4.3133322166964));
#67964=CARTESIAN_POINT('Ctrl Pts',(-11.3697557629721,-6.04771213056323,
1.98550746867938));
#67965=CARTESIAN_POINT('Ctrl Pts',(-11.321479943944,-6.21883286804007,0.476080868258791));
#67966=CARTESIAN_POINT('Ctrl Pts',(-11.3062554182404,-6.21873258297641,
3.74859774820643E-5));
#67967=CARTESIAN_POINT('Origin',(-14.,0.,0.));
#67968=CARTESIAN_POINT('',(-14.25,5.55,-6.79678973526781E-16));
#67969=CARTESIAN_POINT('Origin',(-14.25,0.,0.));
#67970=CARTESIAN_POINT('',(-13.75,5.05,6.18446633569413E-16));
#67971=CARTESIAN_POINT('',(-14.,5.3,-6.49062803548097E-16));
#67972=CARTESIAN_POINT('',(-13.75,-5.05,-6.18446633569413E-16));
#67973=CARTESIAN_POINT('Origin',(-13.75,0.,0.));
#67974=CARTESIAN_POINT('Origin',(-13.75,0.,0.));
#67975=CARTESIAN_POINT('Origin',(1.375,0.,0.));
#67976=CARTESIAN_POINT('',(16.5,5.05,-6.18446633569413E-16));
#67977=CARTESIAN_POINT('',(16.5,-5.05,-6.18446633569413E-16));
#67978=CARTESIAN_POINT('Origin',(16.5,0.,0.));
#67979=CARTESIAN_POINT('Origin',(16.5,0.,0.));
#67980=CARTESIAN_POINT('',(1.375,-5.05,-6.18446633569413E-16));
#67981=CARTESIAN_POINT('',(9.12159512479098,5.,-0.708872343937891));
#67982=CARTESIAN_POINT('',(8.95,5.05,-1.8164630073276E-16));
#67983=CARTESIAN_POINT('Ctrl Pts',(9.12159512479098,5.,-0.708872343937891));
#67984=CARTESIAN_POINT('Ctrl Pts',(9.10247449902065,5.00527119275577,-0.671692216931588));
#67985=CARTESIAN_POINT('Ctrl Pts',(9.08480986974434,5.01024201937277,-0.633637055570846));
#67986=CARTESIAN_POINT('Ctrl Pts',(8.98942081262808,5.03746706515582,-0.404140998411014));
#67987=CARTESIAN_POINT('Ctrl Pts',(8.95,5.05,-0.195962800871854));
#67988=CARTESIAN_POINT('Ctrl Pts',(8.95,5.05,-1.73472347597681E-16));
#67989=CARTESIAN_POINT('',(9.12159512479098,5.,0.708872343937891));
#67990=CARTESIAN_POINT('Ctrl Pts',(8.95,5.05,-1.73472347597681E-16));
#67991=CARTESIAN_POINT('Ctrl Pts',(8.95,5.05,0.195962800871854));
#67992=CARTESIAN_POINT('Ctrl Pts',(8.98942081262808,5.03746706515582,0.404140998411014));
#67993=CARTESIAN_POINT('Ctrl Pts',(9.08480986974434,5.01024201937277,0.633637055570845));
#67994=CARTESIAN_POINT('Ctrl Pts',(9.10247449902065,5.00527119275577,0.671692216931588));
#67995=CARTESIAN_POINT('Ctrl Pts',(9.12159512479098,5.,0.708872343937891));
#67996=CARTESIAN_POINT('',(11.878404875209,5.,0.708872343937891));
#67997=CARTESIAN_POINT('',(1.375,5.,0.708872343937891));
#67998=CARTESIAN_POINT('',(11.878404875209,5.,-0.708872343937891));
#67999=CARTESIAN_POINT('Ctrl Pts',(11.878404875209,5.,0.708872343937891));
#68000=CARTESIAN_POINT('Ctrl Pts',(11.8975255009794,5.00527119275577,0.671692216931588));
#68001=CARTESIAN_POINT('Ctrl Pts',(11.9151901302557,5.01024201937277,0.633637055570845));
#68002=CARTESIAN_POINT('Ctrl Pts',(12.0105791873719,5.03746706515582,0.404140998411014));
#68003=CARTESIAN_POINT('Ctrl Pts',(12.05,5.05,0.195962800871854));
#68004=CARTESIAN_POINT('Ctrl Pts',(12.05,5.05,-0.195962800871853));
#68005=CARTESIAN_POINT('Ctrl Pts',(12.0105791873719,5.03746706515582,-0.404140998411013));
#68006=CARTESIAN_POINT('Ctrl Pts',(11.9151901302557,5.01024201937277,-0.633637055570844));
#68007=CARTESIAN_POINT('Ctrl Pts',(11.8975255009794,5.00527119275577,-0.671692216931587));
#68008=CARTESIAN_POINT('Ctrl Pts',(11.878404875209,5.,-0.708872343937891));
#68009=CARTESIAN_POINT('',(1.375,5.,-0.708872343937891));
#68010=CARTESIAN_POINT('Origin',(-14.25,6.3,0.));
#68011=CARTESIAN_POINT('',(-14.25,-6.3,-7.71527483462833E-16));
#68012=CARTESIAN_POINT('Origin',(-14.25,0.,0.));
#68013=CARTESIAN_POINT('Origin',(16.75,0.,0.));
#68014=CARTESIAN_POINT('',(17.,5.55,6.79678973526781E-16));
#68015=CARTESIAN_POINT('',(16.75,5.3,-6.49062803548097E-16));
#68016=CARTESIAN_POINT('Origin',(17.,0.,0.));
#68017=CARTESIAN_POINT('Origin',(17.,5.05,0.));
#68018=CARTESIAN_POINT('',(17.,-7.6,-9.30731567351989E-16));
#68019=CARTESIAN_POINT('Origin',(17.,0.,0.));
#68020=CARTESIAN_POINT('Ctrl Pts',(10.5,11.8245760568039,-2.04435835333739));
#68021=CARTESIAN_POINT('Ctrl Pts',(10.7582304278698,11.8245760568039,-2.04435835333739));
#68022=CARTESIAN_POINT('Ctrl Pts',(11.3081516759042,11.8433355261774,-1.94148312624803));
#68023=CARTESIAN_POINT('Ctrl Pts',(11.7686177715371,11.8905905388006,-1.62853836082025));
#68024=CARTESIAN_POINT('Ctrl Pts',(12.1310271901565,11.9342839542065,-1.26813573971222));
#68025=CARTESIAN_POINT('Ctrl Pts',(12.4471177841003,11.981691241836,-0.802237030533718));
#68026=CARTESIAN_POINT('Ctrl Pts',(12.573833144828,12.0043367284087,-0.12872161701368));
#68027=CARTESIAN_POINT('Ctrl Pts',(12.501821965583,11.9916659712442,0.655782750176622));
#68028=CARTESIAN_POINT('Ctrl Pts',(12.2256409941389,11.9460677454848,1.17959764711775));
#68029=CARTESIAN_POINT('Ctrl Pts',(11.769637233635,11.8905834208578,1.62938507413833));
#68030=CARTESIAN_POINT('Ctrl Pts',(11.5402696174063,11.8672568247713,1.78727577115204));
#68031=CARTESIAN_POINT('Ctrl Pts',(11.0342336769945,11.8338577790529,1.99483160104378));
#68032=CARTESIAN_POINT('Ctrl Pts',(10.7590524777073,11.8246005449034,2.04641526111906));
#68033=CARTESIAN_POINT('Ctrl Pts',(10.2419038685047,11.8246359138644,2.04555244927938));
#68034=CARTESIAN_POINT('Ctrl Pts',(9.76152674270748,11.8410305581576,1.95718242696326));
#68035=CARTESIAN_POINT('Ctrl Pts',(9.2872402918347,11.8849211742903,1.66633669567092));
#68036=CARTESIAN_POINT('Ctrl Pts',(8.80831114863381,11.9403112406462,1.23618144218895));
#68037=CARTESIAN_POINT('Ctrl Pts',(8.53046789037361,11.9865603322116,0.729866720037598));
#68038=CARTESIAN_POINT('Ctrl Pts',(8.46006855397992,11.9984238321423,0.229180604878363));
#68039=CARTESIAN_POINT('Ctrl Pts',(8.45066730819559,12.0000222095556,0.0975454104158677));
#68040=CARTESIAN_POINT('Ctrl Pts',(8.44002425265866,12.0019480576085,-0.288216463181939));
#68041=CARTESIAN_POINT('Ctrl Pts',(8.58689532600872,11.9752818489509,-0.880228435298227));
#68042=CARTESIAN_POINT('Ctrl Pts',(8.99410238797636,11.9173755533414,-1.41710240312987));
#68043=CARTESIAN_POINT('Ctrl Pts',(9.34406991814095,11.8790166897006,-1.70485788162001));
#68044=CARTESIAN_POINT('Ctrl Pts',(9.83136405381611,11.8382527878677,-1.96874089736921));
#68045=CARTESIAN_POINT('Ctrl Pts',(10.2417708031704,11.8245760568039,-2.04435835333739));
#68046=CARTESIAN_POINT('Ctrl Pts',(10.5,11.8245760568039,-2.04435835333739));
#68047=CARTESIAN_POINT('Ctrl Pts',(10.5,11.6828756306444,-1.87957223555826));
#68048=CARTESIAN_POINT('Ctrl Pts',(10.7398027760933,11.6829069804735,-1.87967019655954));
#68049=CARTESIAN_POINT('Ctrl Pts',(11.2505600171714,11.699146809745,-1.78220242363967));
#68050=CARTESIAN_POINT('Ctrl Pts',(11.6737064964281,11.7398399156241,-1.4904193266981));
#68051=CARTESIAN_POINT('Ctrl Pts',(12.0049140807901,11.7773485944662,-1.15671595176948));
#68052=CARTESIAN_POINT('Ctrl Pts',(12.2910542687146,11.8177655371996,-0.728963555699616));
#68053=CARTESIAN_POINT('Ctrl Pts',(12.4045816142874,11.8370021724303,-0.116752087098428));
#68054=CARTESIAN_POINT('Ctrl Pts',(12.3400974998438,11.8262599163346,0.595201711882176));
#68055=CARTESIAN_POINT('Ctrl Pts',(12.0912278889217,11.787426402354,1.07451743336628));
#68056=CARTESIAN_POINT('Ctrl Pts',(11.6749144056302,11.7399000722776,1.49146106495459));
#68057=CARTESIAN_POINT('Ctrl Pts',(11.4639499848756,11.7197556690285,1.63828893506523));
#68058=CARTESIAN_POINT('Ctrl Pts',(10.9962576770092,11.6909565881495,1.8331120645509));
#68059=CARTESIAN_POINT('Ctrl Pts',(10.7406079241326,11.6828973823575,1.88145785991136));
#68060=CARTESIAN_POINT('Ctrl Pts',(10.2603645125265,11.6829578323396,1.88097023487898));
#68061=CARTESIAN_POINT('Ctrl Pts',(9.81417055101731,11.6971628557272,1.79707772775124));
#68062=CARTESIAN_POINT('Ctrl Pts',(9.37753152881029,11.7349932027385,1.52567415133084));
#68063=CARTESIAN_POINT('Ctrl Pts',(8.93924111117345,11.7825597062905,1.12661882189384));
#68064=CARTESIAN_POINT('Ctrl Pts',(8.68891806495232,11.8219474983071,0.662730723367097));
#68065=CARTESIAN_POINT('Ctrl Pts',(8.62561972670899,11.8320403251539,0.208365587035192));
#68066=CARTESIAN_POINT('Ctrl Pts',(8.6171018952244,11.8334177518436,0.0886180256498179));
#68067=CARTESIAN_POINT('Ctrl Pts',(8.60807558809857,11.8348997741416,-0.261658779614536));
#68068=CARTESIAN_POINT('Ctrl Pts',(8.73914827441268,11.8123885442958,-0.799850727292736));
#68069=CARTESIAN_POINT('Ctrl Pts',(9.10913830169419,11.7628090930054,-1.29430484284161));
#68070=CARTESIAN_POINT('Ctrl Pts',(9.42978691918065,11.7298811826287,-1.56142921347393));
#68071=CARTESIAN_POINT('Ctrl Pts',(9.87903805739242,11.6947195019836,-1.80813827520343));
#68072=CARTESIAN_POINT('Ctrl Pts',(10.2602598473556,11.6828949702791,-1.87963186326188));
#68073=CARTESIAN_POINT('Ctrl Pts',(10.5,11.6828756306444,-1.87957223555826));
#68074=CARTESIAN_POINT('Ctrl Pts',(10.5,11.5411752044848,-1.71478611777913));
#68075=CARTESIAN_POINT('Ctrl Pts',(10.7214715587286,11.5411438546557,-1.71468815677786));
#68076=CARTESIAN_POINT('Ctrl Pts',(11.1928739297933,11.5549205780978,-1.62336308521331));
#68077=CARTESIAN_POINT('Ctrl Pts',(11.5790873321378,11.5891311971719,-1.35148921845341));
#68078=CARTESIAN_POINT('Ctrl Pts',(11.8789049510917,11.6203680543884,-1.0453393213789));
#68079=CARTESIAN_POINT('Ctrl Pts',(12.1354850996937,11.6539745700422,-0.654632815392126));
#68080=CARTESIAN_POINT('Ctrl Pts',(12.235459123101,11.6696685204615,-0.104671223272519));
#68081=CARTESIAN_POINT('Ctrl Pts',(12.1785311912426,11.6608817102649,0.535319205819066));
#68082=CARTESIAN_POINT('Ctrl Pts',(11.9570548103486,11.6288249810861,0.969991925022837));
#68083=CARTESIAN_POINT('Ctrl Pts',(11.5795643809747,11.5890385606483,1.35211162816705));
#68084=CARTESIAN_POINT('Ctrl Pts',(11.3875459523367,11.5722428144048,1.48911191242604));
#68085=CARTESIAN_POINT('Ctrl Pts',(10.9579127537214,11.5479295617558,1.67029625018663));
#68086=CARTESIAN_POINT('Ctrl Pts',(10.7221443818625,11.5411913571738,1.71640740577542));
#68087=CARTESIAN_POINT('Ctrl Pts',(10.278600155584,11.5411826549977,1.71544744258993));
#68088=CARTESIAN_POINT('Ctrl Pts',(9.86678553559699,11.5532267637952,1.63688927133756));
#68089=CARTESIAN_POINT('Ctrl Pts',(9.46792380300963,11.5849776467071,1.38455066231656));
#68090=CARTESIAN_POINT('Ctrl Pts',(9.07028237660262,11.6247208601492,1.01726046285402));
#68091=CARTESIAN_POINT('Ctrl Pts',(8.84748056075628,11.6572783761553,0.596330563124787));
#68092=CARTESIAN_POINT('Ctrl Pts',(8.79154265363212,11.6655159168803,0.187037243054655));
#68093=CARTESIAN_POINT('Ctrl Pts',(8.78410590418262,11.6666169288766,0.0796337437952312));
#68094=CARTESIAN_POINT('Ctrl Pts',(8.77522139956891,11.6681056405353,-0.235179054312069));
#68095=CARTESIAN_POINT('Ctrl Pts',(8.89145925390984,11.6494496025653,-0.719393697895783));
#68096=CARTESIAN_POINT('Ctrl Pts',(9.2236096687965,11.6083855638654,-1.17137711112015));
#68097=CARTESIAN_POINT('Ctrl Pts',(9.51543333718696,11.5807480684238,-1.41804950400415));
#68098=CARTESIAN_POINT('Ctrl Pts',(9.92659698779092,11.5512199541647,-1.64755889631587));
#68099=CARTESIAN_POINT('Ctrl Pts',(10.2784680168167,11.5411558648501,-1.71472649007551));
#68100=CARTESIAN_POINT('Ctrl Pts',(10.5,11.5411752044848,-1.71478611777913));
#68101=CARTESIAN_POINT('Ctrl Pts',(10.5,11.3994747783253,-1.55));
#68102=CARTESIAN_POINT('Ctrl Pts',(10.7030439069521,11.3994747783253,-1.55));
#68103=CARTESIAN_POINT('Ctrl Pts',(11.1352822710605,11.4107318616654,-1.46408238260495));
#68104=CARTESIAN_POINT('Ctrl Pts',(11.4841760570289,11.4383805739953,-1.21337018433126));
#68105=CARTESIAN_POINT('Ctrl Pts',(11.7527918417253,11.4634326946481,-0.933919533436165));
#68106=CARTESIAN_POINT('Ctrl Pts',(11.9794215843079,11.4900488654058,-0.581359340558024));
#68107=CARTESIAN_POINT('Ctrl Pts',(12.0662075925604,11.5023339644831,-0.0927016933572669));
#68108=CARTESIAN_POINT('Ctrl Pts',(12.0168067255034,11.4954756553553,0.47473816752462));
#68109=CARTESIAN_POINT('Ctrl Pts',(11.8226417051315,11.4701836379553,0.864911711271363));
#68110=CARTESIAN_POINT('Ctrl Pts',(11.4848415529699,11.4383552120681,1.21418761898331));
#68111=CARTESIAN_POINT('Ctrl Pts',(11.311226319806,11.4247416586619,1.34012507633923));
#68112=CARTESIAN_POINT('Ctrl Pts',(10.9199367537361,11.4050283708524,1.50857671369375));
#68113=CARTESIAN_POINT('Ctrl Pts',(10.7036998282878,11.399488194628,1.55145000456772));
#68114=CARTESIAN_POINT('Ctrl Pts',(10.2970607996058,11.3995045734729,1.55086522818953));
#68115=CARTESIAN_POINT('Ctrl Pts',(9.91942934390681,11.4093590613647,1.47678457212554));
#68116=CARTESIAN_POINT('Ctrl Pts',(9.55821503998522,11.4350496751553,1.24388811797647));
#68117=CARTESIAN_POINT('Ctrl Pts',(9.20121233914227,11.4669693257936,0.907697842558912));
#68118=CARTESIAN_POINT('Ctrl Pts',(9.00593073533499,11.4926655422508,0.529194566454286));
#68119=CARTESIAN_POINT('Ctrl Pts',(8.95709382636119,11.4991324098919,0.166222225211484));
#68120=CARTESIAN_POINT('Ctrl Pts',(8.95054049121143,11.5000124711646,0.0707063590291814));
#68121=CARTESIAN_POINT('Ctrl Pts',(8.94327273500882,11.5010573570684,-0.208621370744666));
#68122=CARTESIAN_POINT('Ctrl Pts',(9.04371220231381,11.4865562979102,-0.639015989890292));
#68123=CARTESIAN_POINT('Ctrl Pts',(9.33864558251432,11.4538191035294,-1.04857955083189));
#68124=CARTESIAN_POINT('Ctrl Pts',(9.60115033822666,11.4316125613519,-1.27462083585808));
#68125=CARTESIAN_POINT('Ctrl Pts',(9.97427099136723,11.4076866682806,-1.4869562741501));
#68126=CARTESIAN_POINT('Ctrl Pts',(10.296957061002,11.3994747783253,-1.55));
#68127=CARTESIAN_POINT('Ctrl Pts',(10.5,11.3994747783253,-1.55));
#68128=CARTESIAN_POINT('',(10.5,11.8245760568039,-2.04435835333739));
#68129=CARTESIAN_POINT('',(10.5,11.3994747783253,-1.55));
#68130=CARTESIAN_POINT('',(10.5,11.8245760568039,-2.04435835333739));
#68131=CARTESIAN_POINT('',(8.94931572037071,11.5001882310673,0.00068897024722115));
#68132=CARTESIAN_POINT('Ctrl Pts',(10.5,11.3994747783253,-1.55));
#68133=CARTESIAN_POINT('Ctrl Pts',(10.7030439069521,11.3994747783253,-1.55));
#68134=CARTESIAN_POINT('Ctrl Pts',(11.1352822710605,11.4107318616654,-1.46408238260495));
#68135=CARTESIAN_POINT('Ctrl Pts',(11.4841760570289,11.4383805739953,-1.21337018433126));
#68136=CARTESIAN_POINT('Ctrl Pts',(11.7527918417253,11.4634326946481,-0.933919533436165));
#68137=CARTESIAN_POINT('Ctrl Pts',(11.9794215843079,11.4900488654058,-0.581359340558024));
#68138=CARTESIAN_POINT('Ctrl Pts',(12.0662075925604,11.5023339644831,-0.0927016933572669));
#68139=CARTESIAN_POINT('Ctrl Pts',(12.0168067255034,11.4954756553553,0.47473816752462));
#68140=CARTESIAN_POINT('Ctrl Pts',(11.8226417051315,11.4701836379553,0.864911711271363));
#68141=CARTESIAN_POINT('Ctrl Pts',(11.4848415529699,11.4383552120681,1.21418761898331));
#68142=CARTESIAN_POINT('Ctrl Pts',(11.311226319806,11.4247416586619,1.34012507633923));
#68143=CARTESIAN_POINT('Ctrl Pts',(10.9199367537361,11.4050283708524,1.50857671369375));
#68144=CARTESIAN_POINT('Ctrl Pts',(10.7036998282878,11.399488194628,1.55145000456772));
#68145=CARTESIAN_POINT('Ctrl Pts',(10.2970607996058,11.3995045734729,1.55086522818953));
#68146=CARTESIAN_POINT('Ctrl Pts',(9.91942934390681,11.4093590613647,1.47678457212554));
#68147=CARTESIAN_POINT('Ctrl Pts',(9.55821503998522,11.4350496751553,1.24388811797647));
#68148=CARTESIAN_POINT('Ctrl Pts',(9.20121233914227,11.4669693257936,0.907697842558912));
#68149=CARTESIAN_POINT('Ctrl Pts',(9.00593073533499,11.4926655422508,0.529194566454286));
#68150=CARTESIAN_POINT('Ctrl Pts',(8.95709382636119,11.4991324098919,0.166222225211484));
#68151=CARTESIAN_POINT('Ctrl Pts',(8.95054049121143,11.5000124711646,0.0707063590291814));
#68152=CARTESIAN_POINT('Ctrl Pts',(8.94932919851099,11.5001866188152,0.0241517374002067));
#68153=CARTESIAN_POINT('Ctrl Pts',(8.94931572037071,11.5001882310673,0.00068897024722007));
#68154=CARTESIAN_POINT('Ctrl Pts',(8.94931572037071,11.5001882310673,0.00068897024722007));
#68155=CARTESIAN_POINT('Ctrl Pts',(8.94918093896793,11.5002043535885,-0.233938701282644));
#68156=CARTESIAN_POINT('Ctrl Pts',(9.04371220231381,11.4865562979102,-0.639015989890292));
#68157=CARTESIAN_POINT('Ctrl Pts',(9.33864558251432,11.4538191035294,-1.04857955083189));
#68158=CARTESIAN_POINT('Ctrl Pts',(9.60115033822666,11.4316125613519,-1.27462083585808));
#68159=CARTESIAN_POINT('Ctrl Pts',(9.97427099136723,11.4076866682806,-1.4869562741501));
#68160=CARTESIAN_POINT('Ctrl Pts',(10.296957061002,11.3994747783253,-1.55));
#68161=CARTESIAN_POINT('Ctrl Pts',(10.5,11.3994747783253,-1.55));
#68162=CARTESIAN_POINT('Ctrl Pts',(10.5,11.8245760568039,-2.04435835333739));
#68163=CARTESIAN_POINT('Ctrl Pts',(10.2417708031704,11.8245760568039,-2.04435835333739));
#68164=CARTESIAN_POINT('Ctrl Pts',(9.83136405381611,11.8382527878677,-1.96874089736921));
#68165=CARTESIAN_POINT('Ctrl Pts',(9.34406991814095,11.8790166897006,-1.70485788162001));
#68166=CARTESIAN_POINT('Ctrl Pts',(8.99410238797636,11.9173755533414,-1.41710240312987));
#68167=CARTESIAN_POINT('Ctrl Pts',(8.58689532600872,11.9752818489509,-0.880228435298227));
#68168=CARTESIAN_POINT('Ctrl Pts',(8.44002425265866,12.0019480576085,-0.288216463181939));
#68169=CARTESIAN_POINT('Ctrl Pts',(8.45066730819559,12.0000222095556,0.0975454104158677));
#68170=CARTESIAN_POINT('Ctrl Pts',(8.46006855397992,11.9984238321423,0.229180604878363));
#68171=CARTESIAN_POINT('Ctrl Pts',(8.53046789037361,11.9865603322116,0.729866720037598));
#68172=CARTESIAN_POINT('Ctrl Pts',(8.80831114863381,11.9403112406462,1.23618144218895));
#68173=CARTESIAN_POINT('Ctrl Pts',(9.2872402918347,11.8849211742903,1.66633669567092));
#68174=CARTESIAN_POINT('Ctrl Pts',(9.76152674270748,11.8410305581576,1.95718242696326));
#68175=CARTESIAN_POINT('Ctrl Pts',(10.2419038685047,11.8246359138644,2.04555244927938));
#68176=CARTESIAN_POINT('Ctrl Pts',(10.7590524777073,11.8246005449034,2.04641526111906));
#68177=CARTESIAN_POINT('Ctrl Pts',(11.0342336769945,11.8338577790529,1.99483160104378));
#68178=CARTESIAN_POINT('Ctrl Pts',(11.5402696174063,11.8672568247713,1.78727577115204));
#68179=CARTESIAN_POINT('Ctrl Pts',(11.769637233635,11.8905834208578,1.62938507413833));
#68180=CARTESIAN_POINT('Ctrl Pts',(12.2256409941389,11.9460677454848,1.17959764711775));
#68181=CARTESIAN_POINT('Ctrl Pts',(12.501821965583,11.9916659712442,0.655782750176622));
#68182=CARTESIAN_POINT('Ctrl Pts',(12.573833144828,12.0043367284087,-0.12872161701368));
#68183=CARTESIAN_POINT('Ctrl Pts',(12.4471177841003,11.981691241836,-0.802237030533718));
#68184=CARTESIAN_POINT('Ctrl Pts',(12.1310271901565,11.9342839542065,-1.26813573971222));
#68185=CARTESIAN_POINT('Ctrl Pts',(11.7686177715371,11.8905905388006,-1.62853836082025));
#68186=CARTESIAN_POINT('Ctrl Pts',(11.3081516759042,11.8433355261774,-1.94148312624803));
#68187=CARTESIAN_POINT('Ctrl Pts',(10.7582304278698,11.8245760568039,-2.04435835333739));
#68188=CARTESIAN_POINT('Ctrl Pts',(10.5,11.8245760568039,-2.04435835333739));
#68189=CARTESIAN_POINT('Origin',(10.5,12.5,0.));
#68190=CARTESIAN_POINT('',(8.95,12.5,-1.8982025386784E-16));
#68191=CARTESIAN_POINT('Origin',(10.5,5.,0.));
#68192=CARTESIAN_POINT('Origin',(10.5,5.,0.));
#68193=CARTESIAN_POINT('Origin',(10.5,0.,0.));
#68194=CARTESIAN_POINT('',(14.5,-12.,-1.46957615897682E-15));
#68195=CARTESIAN_POINT('Origin',(14.5,0.,0.));
#68196=CARTESIAN_POINT('',(6.5,-12.,-1.46957615897682E-15));
#68197=CARTESIAN_POINT('',(10.5,-12.,-1.46957615897682E-15));
#68198=CARTESIAN_POINT('Origin',(6.5,0.,0.));
#68199=CARTESIAN_POINT('Ctrl Pts',(-14.0290837546341,-2.70929682014932,
5.59810515289136));
#68200=CARTESIAN_POINT('Ctrl Pts',(-13.9960324613096,-3.63933197645688,
5.14799905041672));
#68201=CARTESIAN_POINT('Ctrl Pts',(-13.9299298746607,-5.26981959467749,
3.77580048295898));
#68202=CARTESIAN_POINT('Ctrl Pts',(-13.8307759946872,-6.43349921927399,
0.79679165484266));
#68203=CARTESIAN_POINT('Ctrl Pts',(-13.7316221147138,-6.03180256523361,
-2.37521059424263));
#68204=CARTESIAN_POINT('Ctrl Pts',(-13.6324682347403,-4.1625811938585,-4.96974307260698));
#68205=CARTESIAN_POINT('Ctrl Pts',(-13.5333143547669,-1.28056321092969,
-6.35489385677935));
#68206=CARTESIAN_POINT('Ctrl Pts',(-13.4341604747935,1.91301075045669,-6.193982915654));
#68207=CARTESIAN_POINT('Ctrl Pts',(-13.33500659482,4.64114599103167,-4.52598857637084));
#68208=CARTESIAN_POINT('Ctrl Pts',(-13.2358527148466,6.24006591576224,-1.75683043852266));
#68209=CARTESIAN_POINT('Ctrl Pts',(-13.1366988348732,6.3207503286919,1.43978832745216));
#68210=CARTESIAN_POINT('Ctrl Pts',(-13.0375449548997,4.86356603929123,4.28609183779942));
#68211=CARTESIAN_POINT('Ctrl Pts',(-12.9383910749263,2.2230539416448,6.08957345749443));
#68212=CARTESIAN_POINT('Ctrl Pts',(-12.8392371949529,-0.958337716508845,
6.41143141299502));
#68213=CARTESIAN_POINT('Ctrl Pts',(-12.7400833149794,-3.90656124824087,
5.17335943056773));
#68214=CARTESIAN_POINT('Ctrl Pts',(-12.640929435006,-5.90430033493565,2.67658449074433));
#68215=CARTESIAN_POINT('Ctrl Pts',(-12.5417755550326,-6.46549569135999,
-0.471415594223555));
#68216=CARTESIAN_POINT('Ctrl Pts',(-12.4426216750591,-5.45360592369372,
-3.50471822801767));
#68217=CARTESIAN_POINT('Ctrl Pts',(-12.3434677950857,-3.11482849091286,
-5.68530655580378));
#68218=CARTESIAN_POINT('Ctrl Pts',(-12.2443139151122,-0.0181988194650487,
-6.4826334267188));
#68219=CARTESIAN_POINT('Ctrl Pts',(-12.1451600351388,3.08285871135025,-5.70270544700054));
#68220=CARTESIAN_POINT('Ctrl Pts',(-12.0460061551654,5.43384239437673,-3.5352827494326));
#68221=CARTESIAN_POINT('Ctrl Pts',(-11.9468522751919,6.46274697899828,-0.507709329187834));
#68222=CARTESIAN_POINT('Ctrl Pts',(-11.8476983952185,5.91923519889273,2.64339212664902));
#68223=CARTESIAN_POINT('Ctrl Pts',(-11.7485445152451,3.93554599561895,5.15134399897086));
#68224=CARTESIAN_POINT('Ctrl Pts',(-11.6493906352716,0.994320167882758,
6.4059499435945));
#68225=CARTESIAN_POINT('Ctrl Pts',(-11.5502367552982,-2.18882837604633,
6.10195850675201));
#68226=CARTESIAN_POINT('Ctrl Pts',(-11.4510828753248,-4.83942480730361,
4.3133322166964));
#68227=CARTESIAN_POINT('Ctrl Pts',(-11.3519289953513,-6.31256670006456,
1.47525215966285));
#68228=CARTESIAN_POINT('Ctrl Pts',(-11.2527751153779,-6.2498317879533,-1.72176360155833));
#68229=CARTESIAN_POINT('Ctrl Pts',(-11.1536212354044,-4.66648376653058,
-4.49986627956914));
#68230=CARTESIAN_POINT('Ctrl Pts',(-11.054467355431,-1.94775856528816,-6.18313058641824));
#68231=CARTESIAN_POINT('Ctrl Pts',(-10.9553134754576,1.24486534373372,-6.36201049616318));
#68232=CARTESIAN_POINT('Ctrl Pts',(-10.8561595954841,4.13460773126303,-4.99298369573902));
#68233=CARTESIAN_POINT('Ctrl Pts',(-10.7570057155107,6.01838084932733,-2.40914076587077));
#68234=CARTESIAN_POINT('Ctrl Pts',(-10.6578518355373,6.43785394671903,0.760857304653864));
#68235=CARTESIAN_POINT('Ctrl Pts',(-10.5586979555638,5.2909672700661,3.74573525818645));
#68236=CARTESIAN_POINT('Ctrl Pts',(-10.4595440755904,2.85676367597327,5.81925842156633));
#68237=CARTESIAN_POINT('Ctrl Pts',(-10.360390195617,-0.272503792359383,
6.4769289760257));
#68238=CARTESIAN_POINT('Ctrl Pts',(-10.2612363156435,-3.33546982202023,
5.55873262027628));
#68239=CARTESIAN_POINT('Ctrl Pts',(-10.1620824356701,-5.58690054814797,
3.28807079340383));
#68240=CARTESIAN_POINT('Ctrl Pts',(-10.0629285556967,-6.47901241543966,
0.217406066865759));
#68241=CARTESIAN_POINT('Ctrl Pts',(-9.96377467572322,-5.79475046203404,
-2.90615456575997));
#68242=CARTESIAN_POINT('Ctrl Pts',(-9.86462079574977,-3.70059880012039,
-5.32263429120195));
#68243=CARTESIAN_POINT('Ctrl Pts',(-9.76546691577635,-0.706074257995519,
-6.44409236584388));
#68244=CARTESIAN_POINT('Ctrl Pts',(-9.66631303580289,2.46024143136038,-5.99767283008577));
#68245=CARTESIAN_POINT('Ctrl Pts',(-9.56715915582948,5.02796895074312,-4.0919916309414));
#68246=CARTESIAN_POINT('Ctrl Pts',(-9.46800527585603,6.37236826560774,-1.1907098575248));
#68247=CARTESIAN_POINT('Ctrl Pts',(-9.36885139588261,6.16634077687366,2.00027715599528));
#68248=CARTESIAN_POINT('Ctrl Pts',(-9.26969751590915,4.4600139297068,4.70458744462813));
#68249=CARTESIAN_POINT('Ctrl Pts',(-9.17054363593573,1.66854497323006,6.2642497515377));
#68250=CARTESIAN_POINT('Ctrl Pts',(-9.07138975596228,-1.52888872691469,
6.29979099161586));
#68251=CARTESIAN_POINT('Ctrl Pts',(-8.97223587598886,-4.35433669693118,
4.80256381603513));
#68252=CARTESIAN_POINT('Ctrl Pts',(-8.87308199601541,-6.1203543193245,2.13685055239179));
#68253=CARTESIAN_POINT('Ctrl Pts',(-8.77392811604199,-6.39726130204945,
-1.04876837797101));
#68254=CARTESIAN_POINT('Ctrl Pts',(-8.67477423606854,-5.11768488976202,
-3.97921708963369));
#68255=CARTESIAN_POINT('Ctrl Pts',(-8.57562035609511,-2.5929519681933,-5.94150379684923));
#68256=CARTESIAN_POINT('Ctrl Pts',(-8.47646647612167,0.56265821350308,-6.45819502741354));
#68257=CARTESIAN_POINT('Ctrl Pts',(-8.37731259614824,3.58137103787181,-5.40357740450012));
#68258=CARTESIAN_POINT('Ctrl Pts',(-8.2781587161748,5.72871965048953,-3.0342442952779));
#68259=CARTESIAN_POINT('Ctrl Pts',(-8.17900483620137,6.48224415781214,0.0733345473956177));
#68260=CARTESIAN_POINT('Ctrl Pts',(-8.07985095622792,5.65860854650426,3.16307075399211));
#68261=CARTESIAN_POINT('Ctrl Pts',(-7.98069707625449,3.45820718722118,5.48321715123368));
#68262=CARTESIAN_POINT('Ctrl Pts',(-7.88154319628105,0.416407953241648,
6.46927134179796));
#68263=CARTESIAN_POINT('Ctrl Pts',(-7.78238931630763,-2.72670527029838,
5.88132176013677));
#68264=CARTESIAN_POINT('Ctrl Pts',(-7.68323543633418,-5.20639843392111,
3.86241927094858));
#68265=CARTESIAN_POINT('Ctrl Pts',(-7.58408155636075,-6.41935067082568,
0.903772229215514));
#68266=CARTESIAN_POINT('Ctrl Pts',(-7.48492767638731,-6.07044506667244,
-2.27476679460632));
#68267=CARTESIAN_POINT('Ctrl Pts',(-7.38577379641388,-4.2445719758881,-4.89984448925031));
#68268=CARTESIAN_POINT('Ctrl Pts',(-7.28661991644044,-1.38597480405236,
-6.33276725609456));
#68269=CARTESIAN_POINT('Ctrl Pts',(-7.187466036467,1.80983647653362,-6.22489832893194));
#68270=CARTESIAN_POINT('Ctrl Pts',(-7.08831215649357,4.56530613428956,-4.6024827188757));
#68271=CARTESIAN_POINT('Ctrl Pts',(-6.98915827652013,6.21001560019695,-1.86026168122711));
#68272=CARTESIAN_POINT('Ctrl Pts',(-6.89000439654669,6.34379942025369,1.3345696658175));
#68273=CARTESIAN_POINT('Ctrl Pts',(-6.79085051657326,4.93410736951075,4.204694013061));
#68274=CARTESIAN_POINT('Ctrl Pts',(-6.69169663659982,2.3239240730231,6.05179677287292));
#68275=CARTESIAN_POINT('Ctrl Pts',(-6.59254275662638,-0.851680746854733,
6.42646926257087));
#68276=CARTESIAN_POINT('Ctrl Pts',(-6.49338887665295,-3.8200676843074,5.23755192476806));
#68277=CARTESIAN_POINT('Ctrl Pts',(-6.39423499667952,-5.85901440700082,
2.77431387119195));
#68278=CARTESIAN_POINT('Ctrl Pts',(-6.29508111670607,-6.47243570482011,
-0.363927636077572));
#68279=CARTESIAN_POINT('Ctrl Pts',(-6.19592723673265,-5.51108332618975,
-3.41362385876426));
#68280=CARTESIAN_POINT('Ctrl Pts',(-6.0967733567592,-3.20885877105538,-5.63276953769212));
#68281=CARTESIAN_POINT('Ctrl Pts',(-5.99761947678577,-0.125903969293837,
-6.48143621953093));
#68282=CARTESIAN_POINT('Ctrl Pts',(-5.89846559681233,2.98768385311816,-5.75313935787656));
#68283=CARTESIAN_POINT('Ctrl Pts',(-5.7993117168389,5.37435431396556,-3.62507696267142));
#68284=CARTESIAN_POINT('Ctrl Pts',(-5.70015783686546,6.45341940219507,-0.615016501163695));
#68285=CARTESIAN_POINT('Ctrl Pts',(-5.60100395689203,5.96233756874898,2.5446803323042));
#68286=CARTESIAN_POINT('Ctrl Pts',(-5.50185007691858,4.02059130515946,5.08524461891535));
#68287=CARTESIAN_POINT('Ctrl Pts',(-5.40269619694516,1.10061649827017,6.38854526485231));
#68288=CARTESIAN_POINT('Ctrl Pts',(-5.30354231697171,-2.08714341586264,
6.1374831681197));
#68289=CARTESIAN_POINT('Ctrl Pts',(-5.20438843699829,-4.76709164052158,
4.39314290323005));
#68290=CARTESIAN_POINT('Ctrl Pts',(-5.10523455702484,-6.28718432221605,
1.57993056043994));
#68291=CARTESIAN_POINT('Ctrl Pts',(-5.00608067705141,-6.27757584948428,
-1.61768622770392));
#68292=CARTESIAN_POINT('Ctrl Pts',(-4.90692679707797,-4.74060400838073,
-4.42171244124443));
#68293=CARTESIAN_POINT('Ctrl Pts',(-4.80777291710454,-2.05022118826812,
-6.14991547555801));
#68294=CARTESIAN_POINT('Ctrl Pts',(-4.7086190371311,1.13898997181236,-6.38181550355714));
#68295=CARTESIAN_POINT('Ctrl Pts',(-4.60946515715766,4.05107958026204,-5.06099017107475));
#68296=CARTESIAN_POINT('Ctrl Pts',(-4.51031127718423,5.9775227064379,-2.50880241775846));
#68297=CARTESIAN_POINT('Ctrl Pts',(-4.41115739721079,6.44960678792389,0.653788619124958));
#68298=CARTESIAN_POINT('Ctrl Pts',(-4.31200351723735,5.35247157449903,3.65730984762178));
#68299=CARTESIAN_POINT('Ctrl Pts',(-4.21284963726392,2.9530551606307,5.77099059916091));
#68300=CARTESIAN_POINT('Ctrl Pts',(-4.11369575729048,-0.164853293042968,
6.48056252721199));
#68301=CARTESIAN_POINT('Ctrl Pts',(-4.01454187731705,-3.24265217464831,
5.61338348517005));
#68302=CARTESIAN_POINT('Ctrl Pts',(-3.91538799734361,-5.53149871753584,
3.3804421626809));
#68303=CARTESIAN_POINT('Ctrl Pts',(-3.81623411737017,-6.47450592435959,
0.325023557244591));
#68304=CARTESIAN_POINT('Ctrl Pts',(-3.71708023739674,-5.84223576070193,
-2.80947478965496));
#68305=CARTESIAN_POINT('Ctrl Pts',(-3.6179263574233,-3.78852249476445,-5.26041486804939));
#68306=CARTESIAN_POINT('Ctrl Pts',(-3.51877247744987,-0.813044105235338,
-6.43147157035411));
#68307=CARTESIAN_POINT('Ctrl Pts',(-3.41961859747643,2.36025169231589,-6.03772136043487));
#68308=CARTESIAN_POINT('Ctrl Pts',(-3.32046471750299,4.95928728793312,-4.17496549363898));
#68309=CARTESIAN_POINT('Ctrl Pts',(-3.22131083752956,6.35170524667332,-1.29642112629886));
#68310=CARTESIAN_POINT('Ctrl Pts',(-3.12215695755612,6.19872381031724,1.89754852394804));
#68311=CARTESIAN_POINT('Ctrl Pts',(-3.02300307758268,4.53756407304736,4.62983580273871));
#68312=CARTESIAN_POINT('Ctrl Pts',(-2.92384919760925,1.77239391631247,6.23566252155694));
#68313=CARTESIAN_POINT('Ctrl Pts',(-2.82469531763581,-1.42400791440103,
6.32432357940788));
#68314=CARTESIAN_POINT('Ctrl Pts',(-2.72554143766238,-4.27394200392325,
4.87424732901725));
#68315=CARTESIAN_POINT('Ctrl Pts',(-2.62638755768894,-6.08400614812665,
2.23824405883015));
#68316=CARTESIAN_POINT('Ctrl Pts',(-2.5272336777155,-6.41380333157943,-0.942334389244107));
#68317=CARTESIAN_POINT('Ctrl Pts',(-2.42807979774207,-5.18309236738467,
-3.8936385025436));
#68318=CARTESIAN_POINT('Ctrl Pts',(-2.32892591776863,-2.69131095073478,
-5.89760227921367));
#68319=CARTESIAN_POINT('Ctrl Pts',(-2.2297720377952,0.455278923448612,-6.46665202242975));
#68320=CARTESIAN_POINT('Ctrl Pts',(-2.13061815782176,3.49109732043444,-5.4623352859914));
#68321=CARTESIAN_POINT('Ctrl Pts',(-2.03146427784832,5.67751552051297,-3.12900699770163));
#68322=CARTESIAN_POINT('Ctrl Pts',(-1.93231039787489,6.48256781800243,-0.0343767702148776));
#68323=CARTESIAN_POINT('Ctrl Pts',(-1.83315651790145,5.71038124883349,3.06861748517184));
#68324=CARTESIAN_POINT('Ctrl Pts',(-1.73400263792802,3.54883239268839,5.42500285031601));
#68325=CARTESIAN_POINT('Ctrl Pts',(-1.63484875795458,0.523836128332554,
6.46145981864663));
#68326=CARTESIAN_POINT('Ctrl Pts',(-1.53569487798115,-2.62861189967033,
5.92581359462503));
#68327=CARTESIAN_POINT('Ctrl Pts',(-1.43654099800771,-5.14150644054926,
3.94838939304646));
#68328=CARTESIAN_POINT('Ctrl Pts',(-1.33738711803427,-6.40344857817083,
1.01030370881892));
#68329=CARTESIAN_POINT('Ctrl Pts',(-1.23823323806084,-6.10740192775504,
-2.17359356140592));
#68330=CARTESIAN_POINT('Ctrl Pts',(-1.1390793580874,-4.32539601471359,-4.82864542011847));
#68331=CARTESIAN_POINT('Ctrl Pts',(-1.03992547811397,-1.49100115648436,
-6.30886541532577));
#68332=CARTESIAN_POINT('Ctrl Pts',(-0.940771598140529,1.70616120997042,
-6.25410914542779));
#68333=CARTESIAN_POINT('Ctrl Pts',(-0.841617718167091,4.48820662760173,
-4.67769906527593));
#68334=CARTESIAN_POINT('Ctrl Pts',(-0.742463838193658,6.17825052154845,
-1.96318307101446));
#68335=CARTESIAN_POINT('Ctrl Pts',(-0.643309958220219,6.36509736085303,
1.22898448492769));
#68336=CARTESIAN_POINT('Ctrl Pts',(-0.544156078246782,5.00328644146473,
4.12213440610403));
#68337=CARTESIAN_POINT('Ctrl Pts',(-0.445002198273347,2.42415268673505,
6.01234987577457));
#68338=CARTESIAN_POINT('Ctrl Pts',(-0.34584831829991,-0.744788678740318,
6.43973268865655));
#68339=CARTESIAN_POINT('Ctrl Pts',(-0.246694438326474,-3.73251949855906,
5.3002986208522));
#68340=CARTESIAN_POINT('Ctrl Pts',(-0.14754055835304,-5.81211098394011,
2.87127727461039));
#68341=CARTESIAN_POINT('Ctrl Pts',(-0.0483866783796017,-6.47758886518034,
-0.256339171846516));
#68342=CARTESIAN_POINT('Ctrl Pts',(0.0507672015938321,-5.56703928211486,
-3.32158710689955));
#68343=CARTESIAN_POINT('Ctrl Pts',(0.149921081567268,-3.30200317851016,
-5.5786774675043));
#68344=CARTESIAN_POINT('Ctrl Pts',(0.249074961540705,-0.233574361216745,
-6.47844968299619));
#68345=CARTESIAN_POINT('Ctrl Pts',(0.348228841514139,2.89168418329416,-5.8019849932086));
#68346=CARTESIAN_POINT('Ctrl Pts',(0.447382721487577,5.31338253190132,-3.71387039986819));
#68347=CARTESIAN_POINT('Ctrl Pts',(0.546536601461015,6.44231022572788,-0.722153884441094));
#68348=CARTESIAN_POINT('Ctrl Pts',(0.645690481434449,6.00379391212401,2.44526602603354));
#68349=CARTESIAN_POINT('Ctrl Pts',(0.744844361407886,4.10452664743683,5.01774135222336));
#68350=CARTESIAN_POINT('Ctrl Pts',(0.843998241381322,1.20660898072922,6.36937689613002));
#68351=CARTESIAN_POINT('Ctrl Pts',(0.943152121354761,-1.9848822566212,6.17131345052912));
#68352=CARTESIAN_POINT('Ctrl Pts',(1.04230600132819,-4.69344241962331,4.47174077189317));
#68353=CARTESIAN_POINT('Ctrl Pts',(1.14145988130163,-6.26006623726308,1.68417278876314));
#68354=CARTESIAN_POINT('Ctrl Pts',(1.24061376127507,-6.30358685653012,-1.51316225815738));
#68355=CARTESIAN_POINT('Ctrl Pts',(1.3397676412485,-4.81341550856989,-4.34233789785988));
#68356=CARTESIAN_POINT('Ctrl Pts',(1.43892152122194,-2.15211780533888,-6.11500255349699));
#68357=CARTESIAN_POINT('Ctrl Pts',(1.53807540119537,1.03280015818185,-6.39985867895463));
#68358=CARTESIAN_POINT('Ctrl Pts',(1.63722928116881,3.96643304506188,-5.12759945553204));
#68359=CARTESIAN_POINT('Ctrl Pts',(1.73638316114225,5.93501434493084,-2.60777146291548));
#68360=CARTESIAN_POINT('Ctrl Pts',(1.83553704111568,6.45957908194884,0.546539441742633));
#68361=CARTESIAN_POINT('Ctrl Pts',(1.93469092108912,5.41249821859067,3.56787476112659));
#68362=CARTESIAN_POINT('Ctrl Pts',(2.03384480106256,3.0485313934114,5.72112957559227));
#68363=CARTESIAN_POINT('Ctrl Pts',(2.13299868103599,-0.0571572825696857,
6.48240698524711));
#68364=CARTESIAN_POINT('Ctrl Pts',(2.23215256100943,-3.14893932616178,5.66648465960009));
#68365=CARTESIAN_POINT('Ctrl Pts',(2.33130644098286,-5.47456980244149,3.471880291071));
#68366=CARTESIAN_POINT('Ctrl Pts',(2.4304603209563,-6.46821201217862,0.432551318156661));
#68367=CARTESIAN_POINT('Ctrl Pts',(2.52961420092973,-5.8881081895082,-2.71201940000037));
#68368=CARTESIAN_POINT('Ctrl Pts',(2.62876808090318,-3.87540028951621,-5.19674319871096));
#68369=CARTESIAN_POINT('Ctrl Pts',(2.7279219608766,-0.919789494855471,-6.41707523428578));
#68370=CARTESIAN_POINT('Ctrl Pts',(2.82707584085005,2.25961035703773,-6.07610305308455));
#68371=CARTESIAN_POINT('Ctrl Pts',(2.92622972082348,4.88923651142507,-4.25678677087163));
#68372=CARTESIAN_POINT('Ctrl Pts',(3.02538360079692,6.32928870830338,-1.40177449124226));
#68373=CARTESIAN_POINT('Ctrl Pts',(3.12453748077035,6.22939555800606,1.79429603443556));
#68374=CARTESIAN_POINT('Ctrl Pts',(3.22369136074379,4.61386152810167,4.55380599903706));
#68375=CARTESIAN_POINT('Ctrl Pts',(3.32284524071722,1.87575355343092,6.20535380813579));
#68376=CARTESIAN_POINT('Ctrl Pts',(3.42199912069066,-1.31873397506443,6.34711020702708));
#68377=CARTESIAN_POINT('Ctrl Pts',(3.5211530006641,-4.19236740098541,4.94458520535987));
#68378=CARTESIAN_POINT('Ctrl Pts',(3.62030688063753,-6.04597836127066,2.33901965172245));
#68379=CARTESIAN_POINT('Ctrl Pts',(3.71946076061097,-6.42857469838133,-0.835640249567287));
#68380=CARTESIAN_POINT('Ctrl Pts',(3.8186146405844,-5.24706894496936,-3.80698499626393));
#68381=CARTESIAN_POINT('Ctrl Pts',(3.91776852055784,-2.78892694192586,-5.85207260635886));
#68382=CARTESIAN_POINT('Ctrl Pts',(4.01692240053128,0.347773945463821,-6.47332376513164));
#68383=CARTESIAN_POINT('Ctrl Pts',(4.11607628050471,3.3998598111037,-5.51958517592035));
#68384=CARTESIAN_POINT('Ctrl Pts',(4.21523016047815,5.62474399967788,-3.2229058751893));
#68385=CARTESIAN_POINT('Ctrl Pts',(4.31438404045158,6.48110182257391,-0.142078593380259));
#68386=CARTESIAN_POINT('Ctrl Pts',(4.41353792042502,5.76057749963056,2.97331705330878));
#68387=CARTESIAN_POINT('Ctrl Pts',(4.51269180039846,3.63847783642259,5.36529088040279));
#68388=CARTESIAN_POINT('Ctrl Pts',(4.6118456803719,0.631119752015993,6.45186444679596));
#68389=CARTESIAN_POINT('Ctrl Pts',(4.71099956034532,-2.5297929710906,5.96866954249621));
#68390=CARTESIAN_POINT('Ctrl Pts',(4.81015344031878,-5.07519478672013,4.03326937102785));
#68391=CARTESIAN_POINT('Ctrl Pts',(4.9093073202922,-6.3857791487184,1.1165564855737));
#68392=CARTESIAN_POINT('Ctrl Pts',(5.00846120026564,-6.14267180917851,-2.07182067402597));
#68393=CARTESIAN_POINT('Ctrl Pts',(5.10761508023907,-4.40502769148852,-4.75611250736834));
#68394=CARTESIAN_POINT('Ctrl Pts',(5.20676896021251,-1.59561249292064,-6.28322342394515));
#68395=CARTESIAN_POINT('Ctrl Pts',(5.30592284018595,1.60200834941566,-6.28159039988369));
#68396=CARTESIAN_POINT('Ctrl Pts',(5.40507672015938,4.40988078716951,-4.75162981867586));
#68397=CARTESIAN_POINT('Ctrl Pts',(5.50423060013282,6.14475515867778,-2.06555128428737));
#68398=CARTESIAN_POINT('Ctrl Pts',(5.60338448010625,6.38468584605272,1.12303831208186));
#68399=CARTESIAN_POINT('Ctrl Pts',(5.7025383600797,5.07099150144849,4.03847901383656));
#68400=CARTESIAN_POINT('Ctrl Pts',(5.80169224005312,2.52389427730921,5.97115958776782));
#68401=CARTESIAN_POINT('Ctrl Pts',(5.90084612002658,-0.638069512693321,
6.45139792173227));
#68402=CARTESIAN_POINT('Ctrl Pts',(5.96694870667552,-2.64132982999147,5.72450942764096));
#68403=CARTESIAN_POINT('Ctrl Pts',(6.,-3.49587713861109,5.14372565308808));
#68404=CARTESIAN_POINT('Ctrl Pts',(-13.8917225030894,-2.81294064672976,
5.81225999754714));
#68405=CARTESIAN_POINT('Ctrl Pts',(-13.8586712097649,-3.77855418696971,
5.34493513982917));
#68406=CARTESIAN_POINT('Ctrl Pts',(-13.792568623116,-5.47141591447493,3.92024327990461));
#68407=CARTESIAN_POINT('Ctrl Pts',(-13.6934147431425,-6.67961196425968,
0.827272824525194));
#68408=CARTESIAN_POINT('Ctrl Pts',(-13.5942608631691,-6.26254845264959,
-2.46607399211431));
#68409=CARTESIAN_POINT('Ctrl Pts',(-13.4951069831957,-4.32182024074876,
-5.15986000085787));
#68410=CARTESIAN_POINT('Ctrl Pts',(-13.3959531032222,-1.32955100376653,
-6.59799956300203));
#68411=CARTESIAN_POINT('Ctrl Pts',(-13.2967992232488,1.9861927484542,-6.43093299302389));
#68412=CARTESIAN_POINT('Ctrl Pts',(-13.1976453432754,4.81869247713522,-4.6991297293172));
#68413=CARTESIAN_POINT('Ctrl Pts',(-13.0984914633019,6.47877889280262,-1.82403777732267));
#68414=CARTESIAN_POINT('Ctrl Pts',(-12.9993375833285,6.56254987832162,1.49486725812272));
#68415=CARTESIAN_POINT('Ctrl Pts',(-12.900183703355,5.04962117780174,4.45005576963626));
#68416=CARTESIAN_POINT('Ctrl Pts',(-12.8010298233816,2.30809660492678,6.3225293635006));
#68417=CARTESIAN_POINT('Ctrl Pts',(-12.7018759434082,-0.994998811504643,
6.65669995668465));
#68418=CARTESIAN_POINT('Ctrl Pts',(-12.6027220634347,-4.05600628265989,
5.37126567829685));
#68419=CARTESIAN_POINT('Ctrl Pts',(-12.5035681834613,-6.1301686397452,2.77897691106667));
#68420=CARTESIAN_POINT('Ctrl Pts',(-12.4044143034879,-6.7128324575675,-0.489449541531061));
#68421=CARTESIAN_POINT('Ctrl Pts',(-12.3052604235144,-5.66223296757825,
-3.63879080564613));
#68422=CARTESIAN_POINT('Ctrl Pts',(-12.206106543541,-3.23398588317021,-5.90279727972304));
#68423=CARTESIAN_POINT('Ctrl Pts',(-12.1069526635675,-0.0188950131322108,
-6.73062579494758));
#68424=CARTESIAN_POINT('Ctrl Pts',(-12.0077987835941,3.20079310350503,-5.92086176342652));
#68425=CARTESIAN_POINT('Ctrl Pts',(-11.9086449036207,5.64171338680542,-3.67052456918084));
#68426=CARTESIAN_POINT('Ctrl Pts',(-11.8094910236472,6.70997859354236,-0.527131688995861));
#68427=CARTESIAN_POINT('Ctrl Pts',(-11.7103371436738,6.14567483514093,2.74451477704338));
#68428=CARTESIAN_POINT('Ctrl Pts',(-11.6111832637004,4.08609983809049,5.34840804899111));
#68429=CARTESIAN_POINT('Ctrl Pts',(-11.5120293837269,1.03235776726246,6.65100879432626));
#68430=CARTESIAN_POINT('Ctrl Pts',(-11.4128755037535,-2.27256174440011,
6.33538820133974));
#68431=CARTESIAN_POINT('Ctrl Pts',(-11.3137216237801,-5.02455642586494,
4.47833822597765));
#68432=CARTESIAN_POINT('Ctrl Pts',(-11.2145677438066,-6.55405318595761,
1.53168775500311));
#68433=CARTESIAN_POINT('Ctrl Pts',(-11.1154138638332,-6.4889183572691,-1.78762946269443));
#68434=CARTESIAN_POINT('Ctrl Pts',(-11.0162599838597,-4.84499954621256,
-4.67200812716823));
#68435=CARTESIAN_POINT('Ctrl Pts',(-10.9171061038863,-2.02226983679597,
-6.41966550922812));
#68436=CARTESIAN_POINT('Ctrl Pts',(-10.8179522239129,1.29248751892042,-6.60538844857633));
#68437=CARTESIAN_POINT('Ctrl Pts',(-10.7187983439394,4.29277665667947,-5.18398969125477));
#68438=CARTESIAN_POINT('Ctrl Pts',(-10.619644463966,6.2486132906028,-2.50130215840957));
#68439=CARTESIAN_POINT('Ctrl Pts',(-10.5204905839926,6.68413328128352,0.789963810057592));
#68440=CARTESIAN_POINT('Ctrl Pts',(-10.4213367040191,5.49337259166222,3.88902791354576));
#68441=CARTESIAN_POINT('Ctrl Pts',(-10.3221828240457,2.96604882952749,6.04187345812717));
#68442=CARTESIAN_POINT('Ctrl Pts',(-10.2230289440723,-0.282928392420811,
6.72470312117386));
#68443=CARTESIAN_POINT('Ctrl Pts',(-10.1238750640988,-3.46306782207204,
5.77138127339482));
#68444=CARTESIAN_POINT('Ctrl Pts',(-10.0247211841254,-5.8006267619862,3.41385554927162));
#68445=CARTESIAN_POINT('Ctrl Pts',(-9.92556730415195,-6.72686626231402,
0.225722910012753));
#68446=CARTESIAN_POINT('Ctrl Pts',(-9.82641342417851,-6.01642794952727,
-3.01732916190961));
#68447=CARTESIAN_POINT('Ctrl Pts',(-9.72725954420508,-3.84216476566213,
-5.52625103091307));
#68448=CARTESIAN_POINT('Ctrl Pts',(-9.62810566423164,-0.733085044486097,
-6.69061035038762));
#68449=CARTESIAN_POINT('Ctrl Pts',(-9.5289517842582,2.55435767376008,-6.22711308855605));
#68450=CARTESIAN_POINT('Ctrl Pts',(-9.42979790428477,5.22031330301457,-4.24853028252504));
#68451=CARTESIAN_POINT('Ctrl Pts',(-9.33064402431133,6.6161424532551,-1.23626032104847));
#68452=CARTESIAN_POINT('Ctrl Pts',(-9.2314901443379,6.40223340752278,2.076797519924));
#68453=CARTESIAN_POINT('Ctrl Pts',(-9.13233626436446,4.63063123041715,4.88456087596916));
#68454=CARTESIAN_POINT('Ctrl Pts',(-9.03318238439104,1.73237496208956,6.50388787833003));
#68455=CARTESIAN_POINT('Ctrl Pts',(-8.93402850441757,-1.5873761827352,6.54078874430662));
#68456=CARTESIAN_POINT('Ctrl Pts',(-8.83487462444418,-4.52091132771111,
4.98628532177378));
#68457=CARTESIAN_POINT('Ctrl Pts',(-8.7357207444707,-6.3544877435272,2.21859551530372));
#68458=CARTESIAN_POINT('Ctrl Pts',(-8.6365668644973,-6.64198776983563,-1.08888888713082));
#68459=CARTESIAN_POINT('Ctrl Pts',(-8.53741298452384,-5.31346131457574,
-4.13144156459587));
#68460=CARTESIAN_POINT('Ctrl Pts',(-8.43825910455042,-2.6921450363445,-6.16879531565515));
#68461=CARTESIAN_POINT('Ctrl Pts',(-8.33910522457696,0.584182636324011,
-6.70525250759289));
#68462=CARTESIAN_POINT('Ctrl Pts',(-8.23995134460355,3.71837595959501,-5.61029061335232));
#68463=CARTESIAN_POINT('Ctrl Pts',(-8.14079746463009,5.94787113716593,-3.15031894874656));
#68464=CARTESIAN_POINT('Ctrl Pts',(-8.04164358465668,6.73022163460534,0.0761399517559067));
#68465=CARTESIAN_POINT('Ctrl Pts',(-7.94248970468322,5.87507794126342,3.28407364826723));
#68466=CARTESIAN_POINT('Ctrl Pts',(-7.8433358247098,3.59050049053371,5.6929769690945));
#68467=CARTESIAN_POINT('Ctrl Pts',(-7.74418194473635,0.43233758980697,6.71675254506246));
#68468=CARTESIAN_POINT('Ctrl Pts',(-7.64502806476292,-2.83101505506209,
6.10631102230922));
#68469=CARTESIAN_POINT('Ctrl Pts',(-7.54587418478948,-5.40556858478126,
4.01017565929336));
#68470=CARTESIAN_POINT('Ctrl Pts',(-7.44672030481605,-6.66492216477869,
0.93834592800572));
#68471=CARTESIAN_POINT('Ctrl Pts',(-7.34756642484261,-6.30266921837014,
-2.3617877269079));
#68472=CARTESIAN_POINT('Ctrl Pts',(-7.24841254486918,-4.40694757036174,
-5.08728745553522));
#68473=CARTESIAN_POINT('Ctrl Pts',(-7.14925866489574,-1.43899510480635,
-6.57502651184819));
#68474=CARTESIAN_POINT('Ctrl Pts',(-7.05010478492231,1.879071554993,-6.46303107174794));
#68475=CARTESIAN_POINT('Ctrl Pts',(-6.95095090494887,4.73995137572269,-4.77855014611627));
#68476=CARTESIAN_POINT('Ctrl Pts',(-6.85179702497543,6.44757900600099,-1.93142576987532));
#68477=CARTESIAN_POINT('Ctrl Pts',(-6.752643145002,6.58648071013089,1.38562346914196));
#68478=CARTESIAN_POINT('Ctrl Pts',(-6.65348926502856,5.12286105819178,4.36554408082491));
#68479=CARTESIAN_POINT('Ctrl Pts',(-6.55433538505512,2.4128255111451,6.28330753631641));
#68480=CARTESIAN_POINT('Ctrl Pts',(-6.45518150508169,-0.884261692202764,
6.67231307740171));
#68481=CARTESIAN_POINT('Ctrl Pts',(-6.35602762510826,-3.9662039177586,5.43791384870334));
#68482=CARTESIAN_POINT('Ctrl Pts',(-6.25687374513481,-6.08315030404075,
2.88044491730221));
#68483=CARTESIAN_POINT('Ctrl Pts',(-6.15771986516138,-6.72003796041445,
-0.377849644371708));
#68484=CARTESIAN_POINT('Ctrl Pts',(-6.05856598518794,-5.72190916124855,
-3.54421163216635));
#68485=CARTESIAN_POINT('Ctrl Pts',(-5.95941210521451,-3.33161328045984,
-5.84825046425226));
#68486=CARTESIAN_POINT('Ctrl Pts',(-5.86025822524107,-0.130720410616282,
-6.7293827887416));
#68487=CARTESIAN_POINT('Ctrl Pts',(-5.76110434526764,3.10197734242757,-5.97322501754531));
#68488=CARTESIAN_POINT('Ctrl Pts',(-5.66195046529419,5.57994959697626,-3.76375384933284));
#68489=CARTESIAN_POINT('Ctrl Pts',(-5.56279658532076,6.70029419140152,-0.638543884031722));
#68490=CARTESIAN_POINT('Ctrl Pts',(-5.46364270534732,6.19042608101304,2.64202677478423));
#68491=CARTESIAN_POINT('Ctrl Pts',(-5.36448882537389,4.17439854579983,5.27978004503857));
#68492=CARTESIAN_POINT('Ctrl Pts',(-5.26533494540045,1.14272045108553,6.63293830167551));
#68493=CARTESIAN_POINT('Ctrl Pts',(-5.16618106542702,-2.16698683819769,
6.37227185438924));
#68494=CARTESIAN_POINT('Ctrl Pts',(-5.06702718545358,-4.94945616241849,
4.56120206080161));
#68495=CARTESIAN_POINT('Ctrl Pts',(-4.96787330548015,-6.52769980827313,
1.64037061551165));
#68496=CARTESIAN_POINT('Ctrl Pts',(-4.86871942550671,-6.51772376456351,
-1.67957062132176));
#68497=CARTESIAN_POINT('Ctrl Pts',(-4.76956554553327,-4.92195524907063,
-4.59086452308377));
#68498=CARTESIAN_POINT('Ctrl Pts',(-4.67041166555984,-2.12865215519214,
-6.38517975826516));
#68499=CARTESIAN_POINT('Ctrl Pts',(-4.5712577855864,1.18256189727929,-6.625951094165));
#68500=CARTESIAN_POINT('Ctrl Pts',(-4.47210390561296,4.20605314622856,-5.25459774618991));
#68501=CARTESIAN_POINT('Ctrl Pts',(-4.37295002563953,6.20619212433233,-2.60477635489854));
#68502=CARTESIAN_POINT('Ctrl Pts',(-4.27379614566609,6.69633572602634,0.67879922473925));
#68503=CARTESIAN_POINT('Ctrl Pts',(-4.17464226569266,5.5572297359225,3.7972197994509));
#68504=CARTESIAN_POINT('Ctrl Pts',(-4.07548838571922,3.06602393344096,5.99175915593496));
#68505=CARTESIAN_POINT('Ctrl Pts',(-3.97633450574579,-0.17115973609795,
6.72847567342724));
#68506=CARTESIAN_POINT('Ctrl Pts',(-3.87718062577234,-3.36669944667494,
5.82812280060413));
#68507=CARTESIAN_POINT('Ctrl Pts',(-3.77802674579892,-5.74310554095458,
3.5097605742586));
#68508=CARTESIAN_POINT('Ctrl Pts',(-3.67887286582547,-6.7221873759554,0.337457294645066));
#68509=CARTESIAN_POINT('Ctrl Pts',(-3.57971898585204,-6.06572979262974,
-2.91695091250557));
#68510=CARTESIAN_POINT('Ctrl Pts',(-3.4805651058786,-3.9334519707537,-5.46165141115185));
#68511=CARTESIAN_POINT('Ctrl Pts',(-3.38141122590517,-0.844147010468397,
-6.67750674787232));
#68512=CARTESIAN_POINT('Ctrl Pts',(-3.28225734593173,2.45054283917926,-6.26869367065504));
#68513=CARTESIAN_POINT('Ctrl Pts',(-3.1831034659583,5.1490042313889,-4.33467830043965));
#68514=CARTESIAN_POINT('Ctrl Pts',(-3.08394958598486,6.59468897299686,-1.34601556179596));
#68515=CARTESIAN_POINT('Ctrl Pts',(-2.98479570601143,6.43585525004679,1.97013901631542));
#68516=CARTESIAN_POINT('Ctrl Pts',(-2.88564182603798,4.71114804523789,4.80694961893865));
#68517=CARTESIAN_POINT('Ctrl Pts',(-2.78648794606455,1.84019663409828,6.47420704727741));
#68518=CARTESIAN_POINT('Ctrl Pts',(-2.68733406609112,-1.47848316725324,
6.56625982331739));
#68519=CARTESIAN_POINT('Ctrl Pts',(-2.58818018611768,-4.4374411453149,5.06071107899172));
#68520=CARTESIAN_POINT('Ctrl Pts',(-2.48902630614425,-6.31674907737723,
2.32386781823257));
#68521=CARTESIAN_POINT('Ctrl Pts',(-2.3898724261708,-6.65916261273149,-0.978383278864916));
#68522=CARTESIAN_POINT('Ctrl Pts',(-2.29071854619737,-5.38137094745038,
-4.04258917886792));
#68523=CARTESIAN_POINT('Ctrl Pts',(-2.19156466622393,-2.79426673002688,
-6.12321435070079));
#68524=CARTESIAN_POINT('Ctrl Pts',(-2.0924107862505,0.472695564341056,-6.71403302394436));
#68525=CARTESIAN_POINT('Ctrl Pts',(-1.99325690627706,3.62464883186855,-5.67129627058904));
#68526=CARTESIAN_POINT('Ctrl Pts',(-1.89410302630363,5.89470819930681,-3.24870678704439));
#68527=CARTESIAN_POINT('Ctrl Pts',(-1.79494914633019,6.73055767637759,-0.0356918494576151));
#68528=CARTESIAN_POINT('Ctrl Pts',(-1.69579526635676,5.92883120214271,3.18600708091843));
#68529=CARTESIAN_POINT('Ctrl Pts',(-1.59664138638331,3.68459255242263,5.63253568704139));
#68530=CARTESIAN_POINT('Ctrl Pts',(-1.49748750640989,0.543875416917607,
6.70864219302505));
#68531=CARTESIAN_POINT('Ctrl Pts',(-1.39833362643644,-2.7291691342452,6.15250488661704));
#68532=CARTESIAN_POINT('Ctrl Pts',(-1.29917974646301,-5.33819415594591,
4.09943455815411));
#68533=CARTESIAN_POINT('Ctrl Pts',(-1.20002586648957,-6.64841173946677,
1.04895275664998));
#68534=CARTESIAN_POINT('Ctrl Pts',(-1.10087198651614,-6.34103985976374,
-2.25674412374346));
#68535=CARTESIAN_POINT('Ctrl Pts',(-1.0017181065427,-4.49086352314854,-5.01336467450923));
#68536=CARTESIAN_POINT('Ctrl Pts',(-0.902564226569266,-1.54803922781885,
-6.55021030901278));
#68537=CARTESIAN_POINT('Ctrl Pts',(-0.80341034659583,1.771430203478,-6.49335934454339));
#68538=CARTESIAN_POINT('Ctrl Pts',(-0.704256466622392,4.65990243660605,
-4.8566438848732));
#68539=CARTESIAN_POINT('Ctrl Pts',(-0.605102586648959,6.41459875805902,
-2.03828440514837));
#68540=CARTESIAN_POINT('Ctrl Pts',(-0.50594870667552,6.60859340090657,1.27599913975567));
#68541=CARTESIAN_POINT('Ctrl Pts',(-0.406794826702084,5.19468656728889,
4.27982616595484));
#68542=CARTESIAN_POINT('Ctrl Pts',(-0.307640946728648,2.51688835851528,
6.24235160287639));
#68543=CARTESIAN_POINT('Ctrl Pts',(-0.208487066755212,-0.773280480777033,
6.68608389426968));
#68544=CARTESIAN_POINT('Ctrl Pts',(-0.109333186781774,-3.87530658661073,
5.50306091215922));
#68545=CARTESIAN_POINT('Ctrl Pts',(-0.0101793068083413,-6.03445259612738,
2.9811176441487));
#68546=CARTESIAN_POINT('Ctrl Pts',(0.0889745731650972,-6.72538825430939,
-0.26614539627899));
#68547=CARTESIAN_POINT('Ctrl Pts',(0.188128453138531,-5.78000570559087,
-3.44865402534091));
#68548=CARTESIAN_POINT('Ctrl Pts',(0.287282333111967,-3.42832091610777,
-5.79208910837369));
#68549=CARTESIAN_POINT('Ctrl Pts',(0.386436213085404,-0.242509720534929,
-6.72628200260807));
#68550=CARTESIAN_POINT('Ctrl Pts',(0.485590093058838,3.00230521668917,-6.02393923682869));
#68551=CARTESIAN_POINT('Ctrl Pts',(0.584743973032275,5.51664534666433,-3.85594406887471));
#68552=CARTESIAN_POINT('Ctrl Pts',(0.683897853005714,6.68876003471413,-0.749779795122723));
#68553=CARTESIAN_POINT('Ctrl Pts',(0.783051732979147,6.2334683318573,2.53880938608934));
#68554=CARTESIAN_POINT('Ctrl Pts',(0.882205612952585,4.26154482458082,5.20969444893381));
#68555=CARTESIAN_POINT('Ctrl Pts',(0.981359492926021,1.25276766331399,6.61303664929493));
#68556=CARTESIAN_POINT('Ctrl Pts',(1.08051337289946,-2.0608136905113,6.4073963102156));
#68557=CARTESIAN_POINT('Ctrl Pts',(1.17966725287289,-4.87298949936261,4.6428066815521));
#68558=CARTESIAN_POINT('Ctrl Pts',(1.27882113284633,-6.49954432421604,1.74860061784114));
#68559=CARTESIAN_POINT('Ctrl Pts',(1.37797501281977,-6.54472981958023,-1.57104809979206));
#68560=CARTESIAN_POINT('Ctrl Pts',(1.4771288927932,-4.99755214451164,-4.50845351601304));
#68561=CARTESIAN_POINT('Ctrl Pts',(1.57628277276664,-2.2344468151906,-6.34893124653652));
#68562=CARTESIAN_POINT('Ctrl Pts',(1.67543665274007,1.07230980499896,-6.64468450908441));
#68563=CARTESIAN_POINT('Ctrl Pts',(1.77459053271351,4.11816846792437,-5.32375516087627));
#68564=CARTESIAN_POINT('Ctrl Pts',(1.87374441268695,6.16205761052794,-2.70753144906902));
#68565=CARTESIAN_POINT('Ctrl Pts',(1.97289829266038,6.70668950896931,0.567447242873178));
#68566=CARTESIAN_POINT('Ctrl Pts',(2.07205217263382,5.61955269212147,3.70436338439326));
#68567=CARTESIAN_POINT('Ctrl Pts',(2.17120605260726,3.16515259811441,5.93999070485913));
#68568=CARTESIAN_POINT('Ctrl Pts',(2.27035993258069,-0.0593438275943384,
6.7303906909844));
#68569=CARTESIAN_POINT('Ctrl Pts',(2.36951381255413,-3.26940162435141,5.88325535412594));
#68570=CARTESIAN_POINT('Ctrl Pts',(2.46866769252756,-5.68399881700607,3.60469665733983));
#68571=CARTESIAN_POINT('Ctrl Pts',(2.567821572501,-6.71565269091494,0.449098517220573));
#68572=CARTESIAN_POINT('Ctrl Pts',(2.66697545247443,-6.11335706572648,-2.81576737854816));
#68573=CARTESIAN_POINT('Ctrl Pts',(2.76612933244788,-4.0236532651774,-5.39554398970022));
#68574=CARTESIAN_POINT('Ctrl Pts',(2.8652832124213,-0.954975932231545,-6.66255968168546));
#68575=CARTESIAN_POINT('Ctrl Pts',(2.96443709239475,2.3460514816286,-6.30854365037732));
#68576=CARTESIAN_POINT('Ctrl Pts',(3.06359097236817,5.07627367078402,-4.41962964086989));
#68577=CARTESIAN_POINT('Ctrl Pts',(3.16274485234162,6.57141489262633,-1.45539920714448));
#68578=CARTESIAN_POINT('Ctrl Pts',(3.26189873231505,6.46770034178368,1.86293661513677));
#68579=CARTESIAN_POINT('Ctrl Pts',(3.36105261228849,4.79036425033147,4.72801130416831));
#68580=CARTESIAN_POINT('Ctrl Pts',(3.46020649226192,1.94751028180179,6.44273887764077));
#68581=CARTESIAN_POINT('Ctrl Pts',(3.55936037223536,-1.36918198592865,6.58991815065725));
#68582=CARTESIAN_POINT('Ctrl Pts',(3.6585142522088,-4.35274591567518,5.13373972240108));
#68583=CARTESIAN_POINT('Ctrl Pts',(3.75766813218223,-6.27726654207255,2.42849856940638));
#68584=CARTESIAN_POINT('Ctrl Pts',(3.85682201215567,-6.67449905640789,-0.867607567605545));
#68585=CARTESIAN_POINT('Ctrl Pts',(3.9559758921291,-5.44779494137685,-3.95262075304505));
#68586=CARTESIAN_POINT('Ctrl Pts',(4.05512977210254,-2.89561700931341,-6.07594294564353));
#68587=CARTESIAN_POINT('Ctrl Pts',(4.15428365207598,0.361077996250999,-6.72095999336724));
#68588=CARTESIAN_POINT('Ctrl Pts',(4.25343753204941,3.52992104250486,-5.73073624822614));
#68589=CARTESIAN_POINT('Ctrl Pts',(4.35259141202285,5.83991791023889,-3.3461977548863));
#68590=CARTESIAN_POINT('Ctrl Pts',(4.45174529199628,6.72903559946889,-0.147513793017169));
#68591=CARTESIAN_POINT('Ctrl Pts',(4.55089917196972,5.98094770452458,3.08706094240574));
#68592=CARTESIAN_POINT('Ctrl Pts',(4.65005305194315,3.77766737191036,5.57053944284399));
#68593=CARTESIAN_POINT('Ctrl Pts',(4.7492069319166,0.655263162823926,6.69867975136916));
#68594=CARTESIAN_POINT('Ctrl Pts',(4.84836081189002,-2.62656989934376,6.19700028366044));
#68595=CARTESIAN_POINT('Ctrl Pts',(4.94751469186348,-5.26934575771189,4.18756160956527));
#68596=CARTESIAN_POINT('Ctrl Pts',(5.0466685718369,-6.63006636809895,1.15927022070139));
#68597=CARTESIAN_POINT('Ctrl Pts',(5.14582245181034,-6.37765898629265,-2.15107792670036));
#68598=CARTESIAN_POINT('Ctrl Pts',(5.24497633178377,-4.5735415002168,-4.93805702383651));
#68599=CARTESIAN_POINT('Ctrl Pts',(5.34413021175721,-1.65665245844824,-6.52358738631149));
#68600=CARTESIAN_POINT('Ctrl Pts',(5.44328409173065,1.66329298767028,-6.52189189110945));
#68601=CARTESIAN_POINT('Ctrl Pts',(5.54243797170408,4.57858025049396,-4.93340285042299));
#68602=CARTESIAN_POINT('Ctrl Pts',(5.64159185167752,6.37982203407842,-2.14456870220543));
#68603=CARTESIAN_POINT('Ctrl Pts',(5.74074573165094,6.62893124127026,1.16600000870917));
#68604=CARTESIAN_POINT('Ctrl Pts',(5.8398996116244,5.26498167626374,4.19297054663797));
#68605=CARTESIAN_POINT('Ctrl Pts',(5.93905349159781,2.62044555173564,6.19958558531679));
#68606=CARTESIAN_POINT('Ctrl Pts',(6.03820737157128,-0.662478785766676,
6.69819537944482));
#68607=CARTESIAN_POINT('Ctrl Pts',(6.10430995822022,-2.74237358747327,5.94349985274467));
#68608=CARTESIAN_POINT('Ctrl Pts',(6.1373612515447,-3.62961150141922,5.34049826419562));
#68609=CARTESIAN_POINT('Ctrl Pts',(-13.7543612515447,-2.91658447331021,
6.02641484220292));
#68610=CARTESIAN_POINT('Ctrl Pts',(-13.7213099582202,-3.91777639748254,
5.54187122924162));
#68611=CARTESIAN_POINT('Ctrl Pts',(-13.6552073715713,-5.67301223427239,
4.06468607685024));
#68612=CARTESIAN_POINT('Ctrl Pts',(-13.5560534915978,-6.92572470924536,
0.85775399420773));
#68613=CARTESIAN_POINT('Ctrl Pts',(-13.4568996116244,-6.49329434006559,
-2.55693738998599));
#68614=CARTESIAN_POINT('Ctrl Pts',(-13.357745731651,-4.48105928763902,-5.34997692910876));
#68615=CARTESIAN_POINT('Ctrl Pts',(-13.2585918516775,-1.37853879660337,
-6.84110526922471));
#68616=CARTESIAN_POINT('Ctrl Pts',(-13.1594379717041,2.05937474645172,-6.66788307039378));
#68617=CARTESIAN_POINT('Ctrl Pts',(-13.0602840917306,4.99623896323877,-4.87227088226356));
#68618=CARTESIAN_POINT('Ctrl Pts',(-12.9611302117572,6.71749186984302,-1.89124511612268));
#68619=CARTESIAN_POINT('Ctrl Pts',(-12.8619763317837,6.80434942795133,1.54994618879328));
#68620=CARTESIAN_POINT('Ctrl Pts',(-12.7628224518104,5.23567631631225,4.61401970147312));
#68621=CARTESIAN_POINT('Ctrl Pts',(-12.6636685718369,2.39313926820875,6.55548526950676));
#68622=CARTESIAN_POINT('Ctrl Pts',(-12.5645146918635,-1.03165990650043,
6.90196850037429));
#68623=CARTESIAN_POINT('Ctrl Pts',(-12.46536081189,-4.20545131707893,5.56917192602596));
#68624=CARTESIAN_POINT('Ctrl Pts',(-12.3662069319166,-6.35603694455473,
2.88136933138902));
#68625=CARTESIAN_POINT('Ctrl Pts',(-12.2670530519432,-6.96016922377503,
-0.507483488838575));
#68626=CARTESIAN_POINT('Ctrl Pts',(-12.1678991719697,-5.87086001146276,
-3.77286338327458));
#68627=CARTESIAN_POINT('Ctrl Pts',(-12.0687452919963,-3.35314327542756,
-6.12028800364231));
#68628=CARTESIAN_POINT('Ctrl Pts',(-11.9695914120228,-0.0195912067993729,
-6.97861816317637));
#68629=CARTESIAN_POINT('Ctrl Pts',(-11.8704375320494,3.31872749565981,-6.1390180798525));
#68630=CARTESIAN_POINT('Ctrl Pts',(-11.771283652076,5.84958437923409,-3.80576638892909));
#68631=CARTESIAN_POINT('Ctrl Pts',(-11.6721297721025,6.95721020808646,-0.546554048803889));
#68632=CARTESIAN_POINT('Ctrl Pts',(-11.5729758921291,6.37211447138913,2.84563742743775));
#68633=CARTESIAN_POINT('Ctrl Pts',(-11.4738220121557,4.23665368056203,5.54547209901134));
#68634=CARTESIAN_POINT('Ctrl Pts',(-11.3746681321822,1.07039536664217,6.89606764505803));
#68635=CARTESIAN_POINT('Ctrl Pts',(-11.2755142522088,-2.35629511275388,
6.56881789592747));
#68636=CARTESIAN_POINT('Ctrl Pts',(-11.1763603722354,-5.20968804442629,
4.64334423525892));
#68637=CARTESIAN_POINT('Ctrl Pts',(-11.0772064922619,-6.79553967185065,
1.58812335034336));
#68638=CARTESIAN_POINT('Ctrl Pts',(-10.9780526122885,-6.7280049265849,-1.85349532383051));
#68639=CARTESIAN_POINT('Ctrl Pts',(-10.8788987323151,-5.02351532589454,
-4.84414997476734));
#68640=CARTESIAN_POINT('Ctrl Pts',(-10.7797448523416,-2.09678110830378,
-6.656200432038));
#68641=CARTESIAN_POINT('Ctrl Pts',(-10.6805909723682,1.34010969410712,-6.84876640098948));
#68642=CARTESIAN_POINT('Ctrl Pts',(-10.5814370923947,4.45094558209592,-5.37499568677053));
#68643=CARTESIAN_POINT('Ctrl Pts',(-10.4822832124213,6.47884573187826,-2.59346355094835));
#68644=CARTESIAN_POINT('Ctrl Pts',(-10.3831293324479,6.93041261584803,0.819070315461309));
#68645=CARTESIAN_POINT('Ctrl Pts',(-10.2839754524744,5.69577791325833,4.03232056890508));
#68646=CARTESIAN_POINT('Ctrl Pts',(-10.184821572501,3.07533398308171,6.26448849468798));
#68647=CARTESIAN_POINT('Ctrl Pts',(-10.0856676925276,-0.293352992482243,
6.97247726632205));
#68648=CARTESIAN_POINT('Ctrl Pts',(-9.98651381255412,-3.59066582212385,
5.98402992651335));
#68649=CARTESIAN_POINT('Ctrl Pts',(-9.8873599325807,-6.01435297582444,3.53964030513942));
#68650=CARTESIAN_POINT('Ctrl Pts',(-9.78820605260725,-6.97472010918838,
0.234039753159747));
#68651=CARTESIAN_POINT('Ctrl Pts',(-9.68905217263381,-6.23810543702052,
-3.12850375805924));
#68652=CARTESIAN_POINT('Ctrl Pts',(-9.58989829266039,-3.98373073120386,
-5.72986777062419));
#68653=CARTESIAN_POINT('Ctrl Pts',(-9.49074441268694,-0.760095830976685,
-6.93712833493136));
#68654=CARTESIAN_POINT('Ctrl Pts',(-9.39159053271351,2.64847391615979,-6.45655334702634));
#68655=CARTESIAN_POINT('Ctrl Pts',(-9.29243665274007,5.41265765528602,-4.40506893410868));
#68656=CARTESIAN_POINT('Ctrl Pts',(-9.19328277276664,6.85991664090245,-1.28181078457213));
#68657=CARTESIAN_POINT('Ctrl Pts',(-9.0941288927932,6.6381260381719,2.15331788385273));
#68658=CARTESIAN_POINT('Ctrl Pts',(-8.99497501281976,4.8012485311275,5.06453430731019));
#68659=CARTESIAN_POINT('Ctrl Pts',(-8.89582113284634,1.79620495094906,6.74352600512238));
#68660=CARTESIAN_POINT('Ctrl Pts',(-8.79666725287289,-1.64586363855569,
6.78178649699738));
#68661=CARTESIAN_POINT('Ctrl Pts',(-8.69751337289946,-4.68748595849105,
5.17000682751243));
#68662=CARTESIAN_POINT('Ctrl Pts',(-8.59835949292602,-6.58862116772988,
2.30034047821565));
#68663=CARTESIAN_POINT('Ctrl Pts',(-8.49920561295258,-6.88671423762183,
-1.12900939629063));
#68664=CARTESIAN_POINT('Ctrl Pts',(-8.40005173297915,-5.50923773938943,
-4.28366603955806));
#68665=CARTESIAN_POINT('Ctrl Pts',(-8.30089785300571,-2.79133810449572,
-6.39608683446105));
#68666=CARTESIAN_POINT('Ctrl Pts',(-8.20174397303227,0.605707059144963,
-6.95230998777225));
#68667=CARTESIAN_POINT('Ctrl Pts',(-8.10259009305884,3.85538088131818,-5.81700382220452));
#68668=CARTESIAN_POINT('Ctrl Pts',(-8.0034362130854,6.16702262384234,-3.26639360221523));
#68669=CARTESIAN_POINT('Ctrl Pts',(-7.90428233311197,6.97819911139855,0.0789453561161987));
#68670=CARTESIAN_POINT('Ctrl Pts',(-7.80512845313852,6.09154733602257,3.40507654254235));
#68671=CARTESIAN_POINT('Ctrl Pts',(-7.7059745731651,3.72279379384625,5.90273678695532));
#68672=CARTESIAN_POINT('Ctrl Pts',(-7.60682069319165,0.448267226372286,
6.96423374832697));
#68673=CARTESIAN_POINT('Ctrl Pts',(-7.50766681321823,-2.9353248398258,6.33130028448165));
#68674=CARTESIAN_POINT('Ctrl Pts',(-7.40851293324478,-5.60473873564142,
4.15793204763815));
#68675=CARTESIAN_POINT('Ctrl Pts',(-7.30935905327135,-6.91049365873169,
0.972919626795923));
#68676=CARTESIAN_POINT('Ctrl Pts',(-7.21020517329792,-6.53489337006783,
-2.44880865920948));
#68677=CARTESIAN_POINT('Ctrl Pts',(-7.11105129332448,-4.56932316483537,
-5.27473042182012));
#68678=CARTESIAN_POINT('Ctrl Pts',(-7.01189741335104,-1.49201540556034,
-6.81728576760183));
#68679=CARTESIAN_POINT('Ctrl Pts',(-6.9127435333776,1.94830663345238,-6.70116381456395));
#68680=CARTESIAN_POINT('Ctrl Pts',(-6.81358965340418,4.91459661715582,-4.95461757335684));
#68681=CARTESIAN_POINT('Ctrl Pts',(-6.71443577343073,6.68514241180503,-2.00258985852354));
#68682=CARTESIAN_POINT('Ctrl Pts',(-6.6152818934573,6.82916200000809,1.43667727246641));
#68683=CARTESIAN_POINT('Ctrl Pts',(-6.51612801348386,5.31161474687281,4.52639414858881));
#68684=CARTESIAN_POINT('Ctrl Pts',(-6.41697413351043,2.50172694926709,6.51481829975991));
#68685=CARTESIAN_POINT('Ctrl Pts',(-6.31782025353699,-0.916842637550795,
6.91815689223255));
#68686=CARTESIAN_POINT('Ctrl Pts',(-6.21866637356355,-4.11234015120979,
5.63827577263862));
#68687=CARTESIAN_POINT('Ctrl Pts',(-6.11951249359012,-6.30728620108067,
2.98657596341246));
#68688=CARTESIAN_POINT('Ctrl Pts',(-6.02035861361668,-6.9676402160088,-0.391771652665847));
#68689=CARTESIAN_POINT('Ctrl Pts',(-5.92120473364325,-5.93273499630734,
-3.67479940556843));
#68690=CARTESIAN_POINT('Ctrl Pts',(-5.82205085366981,-3.4543677898643,-6.06373139081241));
#68691=CARTESIAN_POINT('Ctrl Pts',(-5.72289697369637,-0.135536851938726,
-6.97732935795225));
#68692=CARTESIAN_POINT('Ctrl Pts',(-5.62374309372294,3.21627083173698,-6.19331067721406));
#68693=CARTESIAN_POINT('Ctrl Pts',(-5.5245892137495,5.78554487998695,-3.90243073599426));
#68694=CARTESIAN_POINT('Ctrl Pts',(-5.42543533377606,6.94716898060797,-0.662071266899751));
#68695=CARTESIAN_POINT('Ctrl Pts',(-5.32628145380263,6.4185145932771,2.73937321726426));
#68696=CARTESIAN_POINT('Ctrl Pts',(-5.22712757382919,4.3282057864402,5.4743154711618));
#68697=CARTESIAN_POINT('Ctrl Pts',(-5.12797369385576,1.18482440390089,6.87733133849872));
#68698=CARTESIAN_POINT('Ctrl Pts',(-5.02881981388231,-2.24683026053273,
6.60706054065878));
#68699=CARTESIAN_POINT('Ctrl Pts',(-4.92966593390888,-5.13182068431539,
4.72926121837316));
#68700=CARTESIAN_POINT('Ctrl Pts',(-4.83051205393545,-6.76821529433023,
1.70081067058338));
#68701=CARTESIAN_POINT('Ctrl Pts',(-4.73135817396201,-6.75787167964274,
-1.7414550149396));
#68702=CARTESIAN_POINT('Ctrl Pts',(-4.63220429398857,-5.10330648976053,
-4.76001660492311));
#68703=CARTESIAN_POINT('Ctrl Pts',(-4.53305041401514,-2.20708312211616,
-6.62044404097231));
#68704=CARTESIAN_POINT('Ctrl Pts',(-4.43389653404171,1.22613382274623,-6.87008668477287));
#68705=CARTESIAN_POINT('Ctrl Pts',(-4.33474265406826,4.36102671219507,-5.44820532130507));
#68706=CARTESIAN_POINT('Ctrl Pts',(-4.23558877409484,6.43486154222677,-2.70075029203863));
#68707=CARTESIAN_POINT('Ctrl Pts',(-4.13643489412139,6.94306466412877,0.703809830353542));
#68708=CARTESIAN_POINT('Ctrl Pts',(-4.03728101414796,5.76198789734599,3.93712975128002));
#68709=CARTESIAN_POINT('Ctrl Pts',(-3.93812713417452,3.1789927062512,6.21252771270901));
#68710=CARTESIAN_POINT('Ctrl Pts',(-3.83897325420109,-0.177466179152926,
6.97638881964248));
#68711=CARTESIAN_POINT('Ctrl Pts',(-3.73981937422764,-3.49074671870157,
6.04286211603823));
#68712=CARTESIAN_POINT('Ctrl Pts',(-3.64066549425422,-5.95471236437332,
3.63907898583629));
#68713=CARTESIAN_POINT('Ctrl Pts',(-3.54151161428077,-6.9698688275512,0.349891032045548));
#68714=CARTESIAN_POINT('Ctrl Pts',(-3.44235773430735,-6.28922382455756,
-3.02442703535618));
#68715=CARTESIAN_POINT('Ctrl Pts',(-3.3432038543339,-4.07838144674295,-5.66288795425431));
#68716=CARTESIAN_POINT('Ctrl Pts',(-3.24404997436047,-0.875249915701455,
-6.92354192539052));
#68717=CARTESIAN_POINT('Ctrl Pts',(-3.14489609438703,2.54083398604264,-6.49966598087521));
#68718=CARTESIAN_POINT('Ctrl Pts',(-3.0457422144136,5.33872117484468,-4.49439110724032));
#68719=CARTESIAN_POINT('Ctrl Pts',(-2.94658833444016,6.83767269932039,-1.39560999729307));
#68720=CARTESIAN_POINT('Ctrl Pts',(-2.84743445446673,6.67298668977635,2.04272950868281));
#68721=CARTESIAN_POINT('Ctrl Pts',(-2.74828057449329,4.88473201742842,4.9840634351386));
#68722=CARTESIAN_POINT('Ctrl Pts',(-2.64912669451986,1.90799935188411,6.71275157299788));
#68723=CARTESIAN_POINT('Ctrl Pts',(-2.54997281454641,-1.53295842010545,
6.80819606722689));
#68724=CARTESIAN_POINT('Ctrl Pts',(-2.45081893457298,-4.60094028670655,
5.2471748289662));
#68725=CARTESIAN_POINT('Ctrl Pts',(-2.35166505459954,-6.54949200662783,
2.40949157763498));
#68726=CARTESIAN_POINT('Ctrl Pts',(-2.25251117462611,-6.90452189388355,
-1.01443216848572));
#68727=CARTESIAN_POINT('Ctrl Pts',(-2.15335729465267,-5.57964952751609,
-4.19153985519224));
#68728=CARTESIAN_POINT('Ctrl Pts',(-2.05420341467924,-2.89722250931899,
-6.3488264221879));
#68729=CARTESIAN_POINT('Ctrl Pts',(-1.9550495347058,0.490112205233504,-6.96141402545897));
#68730=CARTESIAN_POINT('Ctrl Pts',(-1.85589565473236,3.75820034330266,-5.88025725518668));
#68731=CARTESIAN_POINT('Ctrl Pts',(-1.75674177475893,6.11190087810066,-3.36840657638715));
#68732=CARTESIAN_POINT('Ctrl Pts',(-1.65758789478549,6.97854753475277,-0.0370069287003618));
#68733=CARTESIAN_POINT('Ctrl Pts',(-1.55843401481206,6.14728115545192,3.30339667666503));
#68734=CARTESIAN_POINT('Ctrl Pts',(-1.45928013483862,3.82035271215688,5.84006852376676));
#68735=CARTESIAN_POINT('Ctrl Pts',(-1.36012625486519,0.563914705502657,
6.95582456740348));
#68736=CARTESIAN_POINT('Ctrl Pts',(-1.26097237489175,-2.82972636882007,
6.37919617860903));
#68737=CARTESIAN_POINT('Ctrl Pts',(-1.16181849491831,-5.53488187134256,
4.25047972326176));
#68738=CARTESIAN_POINT('Ctrl Pts',(-1.06266461494487,-6.8933749007627,1.08760180448103));
#68739=CARTESIAN_POINT('Ctrl Pts',(-0.96351073497144,-6.57467779177244,
-2.33989468608098));
#68740=CARTESIAN_POINT('Ctrl Pts',(-0.864356854998002,-4.65633103158349,
-5.1980839289));
#68741=CARTESIAN_POINT('Ctrl Pts',(-0.765202975024568,-1.60507729915334,
-6.79155520269978));
#68742=CARTESIAN_POINT('Ctrl Pts',(-0.666049095051131,1.83669919698557,
-6.73260954365901));
#68743=CARTESIAN_POINT('Ctrl Pts',(-0.566895215077694,4.83159824561038,
-5.03558870447046));
#68744=CARTESIAN_POINT('Ctrl Pts',(-0.46774133510426,6.65094699456959,-2.11338573928228));
#68745=CARTESIAN_POINT('Ctrl Pts',(-0.368587455130822,6.85208944096011,
1.32301379458366));
#68746=CARTESIAN_POINT('Ctrl Pts',(-0.269433575157385,5.38608669311305,
4.43751792580564));
#68747=CARTESIAN_POINT('Ctrl Pts',(-0.17027969518395,2.6096240302955,6.47235332997821));
#68748=CARTESIAN_POINT('Ctrl Pts',(-0.0711258152105136,-0.801772282813753,
6.93243509988283));
#68749=CARTESIAN_POINT('Ctrl Pts',(0.0280280647629242,-4.01809367466241,
5.70582320346624));
#68750=CARTESIAN_POINT('Ctrl Pts',(0.127181944736357,-6.25679420831466,
3.09095801368702));
#68751=CARTESIAN_POINT('Ctrl Pts',(0.226335824709796,-6.97318764343842,
-0.275951620711471));
#68752=CARTESIAN_POINT('Ctrl Pts',(0.325489704683229,-5.9929721290669,-3.57572094378226));
#68753=CARTESIAN_POINT('Ctrl Pts',(0.424643584656666,-3.55463865370539,
-6.00550074924309));
#68754=CARTESIAN_POINT('Ctrl Pts',(0.523797464630102,-0.251445079853116,
-6.97411432221995));
#68755=CARTESIAN_POINT('Ctrl Pts',(0.622951344603537,3.11292625008419,-6.24589348044878));
#68756=CARTESIAN_POINT('Ctrl Pts',(0.722105224576973,5.71990816142732,-3.99801773788122));
#68757=CARTESIAN_POINT('Ctrl Pts',(0.821259104550414,6.93520984370039,-0.777405705804355));
#68758=CARTESIAN_POINT('Ctrl Pts',(0.920412984523845,6.46314275159058,2.63235274614514));
#68759=CARTESIAN_POINT('Ctrl Pts',(1.01956686449728,4.41856300172481,5.40164754564424));
#68760=CARTESIAN_POINT('Ctrl Pts',(1.11872074447072,1.29892634589875,6.85669640245985));
#68761=CARTESIAN_POINT('Ctrl Pts',(1.21787462444416,-2.1367451244014,6.64347916990207));
#68762=CARTESIAN_POINT('Ctrl Pts',(1.31702850441759,-5.05253657910191,4.81387259121105));
#68763=CARTESIAN_POINT('Ctrl Pts',(1.41618238439103,-6.73902241116898,1.81302844691914));
#68764=CARTESIAN_POINT('Ctrl Pts',(1.51533626436446,-6.78587278263037,-1.62893394142675));
#68765=CARTESIAN_POINT('Ctrl Pts',(1.6144901443379,-5.18168878045337,-4.6745691341662));
#68766=CARTESIAN_POINT('Ctrl Pts',(1.71364402431134,-2.31677582504233,-6.58285993957605));
#68767=CARTESIAN_POINT('Ctrl Pts',(1.81279790428477,1.11181945181607,-6.88951033921419));
#68768=CARTESIAN_POINT('Ctrl Pts',(1.91195178425821,4.26990389078685,-5.5199108662205));
#68769=CARTESIAN_POINT('Ctrl Pts',(2.01110566423164,6.38910087612505,-2.80729143522257));
#68770=CARTESIAN_POINT('Ctrl Pts',(2.11025954420508,6.95379993598976,0.588355044003722));
#68771=CARTESIAN_POINT('Ctrl Pts',(2.20941342417852,5.82660716565228,3.84085200765993));
#68772=CARTESIAN_POINT('Ctrl Pts',(2.30856730415196,3.28177380281742,6.158851834126));
#68773=CARTESIAN_POINT('Ctrl Pts',(2.40772118412539,-0.0615303726189893,
6.97837439672171));
#68774=CARTESIAN_POINT('Ctrl Pts',(2.50687506409883,-3.38986392254105,6.10002604865179));
#68775=CARTESIAN_POINT('Ctrl Pts',(2.60602894407226,-5.89342783157066,3.73751302360866));
#68776=CARTESIAN_POINT('Ctrl Pts',(2.7051828240457,-6.96309336965125,0.465645716284481));
#68777=CARTESIAN_POINT('Ctrl Pts',(2.80433670401913,-6.33860594194476,-2.91951535709594));
#68778=CARTESIAN_POINT('Ctrl Pts',(2.90349058399257,-4.17190624083858,-5.59434478068947));
#68779=CARTESIAN_POINT('Ctrl Pts',(3.002644463966,-0.990162369607622,-6.90804412908513));
#68780=CARTESIAN_POINT('Ctrl Pts',(3.10179834393944,2.43249260621947,-6.54098424767011));
#68781=CARTESIAN_POINT('Ctrl Pts',(3.20095222391288,5.26331083014297,-4.58247251086813));
#68782=CARTESIAN_POINT('Ctrl Pts',(3.30010610388631,6.81354107694928,-1.5090239230467));
#68783=CARTESIAN_POINT('Ctrl Pts',(3.39925998385975,6.70600512556131,1.93157719583798));
#68784=CARTESIAN_POINT('Ctrl Pts',(3.49841386383318,4.96686697256125,4.90221660929955));
#68785=CARTESIAN_POINT('Ctrl Pts',(3.59756774380662,2.01926701017267,6.68012394714576));
#68786=CARTESIAN_POINT('Ctrl Pts',(3.69672162378006,-1.41962999679287,6.83272609428742));
#68787=CARTESIAN_POINT('Ctrl Pts',(3.7958755037535,-4.51312443036494,5.3228942394423));
#68788=CARTESIAN_POINT('Ctrl Pts',(3.89502938372693,-6.50855472287447,2.5179774870903));
#68789=CARTESIAN_POINT('Ctrl Pts',(3.99418326370037,-6.92042341443442,-0.899574885643797));
#68790=CARTESIAN_POINT('Ctrl Pts',(4.0933371436738,-5.64852093778436,-4.09825650982619));
#68791=CARTESIAN_POINT('Ctrl Pts',(4.19249102364723,-3.00230707670095,-6.29981328492818));
#68792=CARTESIAN_POINT('Ctrl Pts',(4.29164490362068,0.374382047038171,-6.96859622160285));
#68793=CARTESIAN_POINT('Ctrl Pts',(4.39079878359411,3.65998227390602,-5.94188732053192));
#68794=CARTESIAN_POINT('Ctrl Pts',(4.48995266356754,6.05509182079991,-3.4694896345833));
#68795=CARTESIAN_POINT('Ctrl Pts',(4.58910654354098,6.97696937636385,-0.152948992654073));
#68796=CARTESIAN_POINT('Ctrl Pts',(4.68826042351442,6.2013179094186,3.2008048315027));
#68797=CARTESIAN_POINT('Ctrl Pts',(4.78741430348786,3.91685690739814,5.77578800528519));
#68798=CARTESIAN_POINT('Ctrl Pts',(4.8865681834613,0.67940657363186,6.94549505594236));
#68799=CARTESIAN_POINT('Ctrl Pts',(4.98572206343472,-2.72334682759693,6.42533102482466));
#68800=CARTESIAN_POINT('Ctrl Pts',(5.08487594340817,-5.46349672870364,4.34185384810268));
#68801=CARTESIAN_POINT('Ctrl Pts',(5.1840298233816,-6.87435358747951,1.20198395582908));
#68802=CARTESIAN_POINT('Ctrl Pts',(5.28318370335504,-6.61264616340679,-2.23033517937476));
#68803=CARTESIAN_POINT('Ctrl Pts',(5.38233758332847,-4.74205530894508,-5.12000154030467));
#68804=CARTESIAN_POINT('Ctrl Pts',(5.48149146330192,-1.71769242397583,-6.76395134867786));
#68805=CARTESIAN_POINT('Ctrl Pts',(5.58064534327534,1.7245776259249,-6.76219338233518));
#68806=CARTESIAN_POINT('Ctrl Pts',(5.67979922324879,4.74727971381842,-5.11517588217014));
#68807=CARTESIAN_POINT('Ctrl Pts',(5.77895310322222,6.61488890947906,-2.22358612012347));
#68808=CARTESIAN_POINT('Ctrl Pts',(5.87810698319565,6.8731766364878,1.20896170533647));
#68809=CARTESIAN_POINT('Ctrl Pts',(5.9772608631691,5.45897185107899,4.34746207943939));
#68810=CARTESIAN_POINT('Ctrl Pts',(6.07641474314252,2.71699682616207,6.42801158286575));
#68811=CARTESIAN_POINT('Ctrl Pts',(6.17556862311597,-0.686888058840034,
6.94499283715739));
#68812=CARTESIAN_POINT('Ctrl Pts',(6.24167120976492,-2.84341734495507,6.16249027784839));
#68813=CARTESIAN_POINT('Ctrl Pts',(6.2747225030894,-3.76334586422734,5.53727087530317));
#68814=CARTESIAN_POINT('Ctrl Pts',(-13.617,-3.02022829989065,6.2405696868587));
#68815=CARTESIAN_POINT('Ctrl Pts',(-13.5839487066755,-4.05699860799537,
5.73880731865407));
#68816=CARTESIAN_POINT('Ctrl Pts',(-13.5178461200266,-5.87460855406983,
4.20912887379586));
#68817=CARTESIAN_POINT('Ctrl Pts',(-13.4186922400531,-7.17183745423105,
0.88823516389027));
#68818=CARTESIAN_POINT('Ctrl Pts',(-13.3195383600797,-6.72404022748158,
-2.64780078785767));
#68819=CARTESIAN_POINT('Ctrl Pts',(-13.2203844801063,-4.64029833452928,
-5.54009385735964));
#68820=CARTESIAN_POINT('Ctrl Pts',(-13.1212306001328,-1.4275265894402,-7.08421097544739));
#68821=CARTESIAN_POINT('Ctrl Pts',(-13.0220767201594,2.13255674444923,-6.90483314776367));
#68822=CARTESIAN_POINT('Ctrl Pts',(-12.922922840186,5.17378544934233,-5.04541203520993));
#68823=CARTESIAN_POINT('Ctrl Pts',(-12.8237689602125,6.95620484688339,-1.95845245492269));
#68824=CARTESIAN_POINT('Ctrl Pts',(-12.7246150802391,7.04614897758106,1.60502511946383));
#68825=CARTESIAN_POINT('Ctrl Pts',(-12.6254612002656,5.42173145482275,4.77798363330997));
#68826=CARTESIAN_POINT('Ctrl Pts',(-12.5263073202922,2.47818193149074,6.78844117551293));
#68827=CARTESIAN_POINT('Ctrl Pts',(-12.4271534403188,-1.06832100149623,
7.14723704406392));
#68828=CARTESIAN_POINT('Ctrl Pts',(-12.3279995603453,-4.35489635149795,
5.76707817375509));
#68829=CARTESIAN_POINT('Ctrl Pts',(-12.2288456803719,-6.58190524936427,
2.98376175171135));
#68830=CARTESIAN_POINT('Ctrl Pts',(-12.1296918003985,-7.20750598998253,
-0.52551743614608));
#68831=CARTESIAN_POINT('Ctrl Pts',(-12.030537920425,-6.07948705534731,-3.90693596090304));
#68832=CARTESIAN_POINT('Ctrl Pts',(-11.9313840404516,-3.47230066768488,
-6.33777872756158));
#68833=CARTESIAN_POINT('Ctrl Pts',(-11.8322301604781,-0.0202874004665461,
-7.22661053140516));
#68834=CARTESIAN_POINT('Ctrl Pts',(-11.7330762805047,3.4366618878146,-6.35717439627847));
#68835=CARTESIAN_POINT('Ctrl Pts',(-11.6339224005313,6.05745537166277,-3.94100820867734));
#68836=CARTESIAN_POINT('Ctrl Pts',(-11.5347685205578,7.20444182263055,-0.565976408611909));
#68837=CARTESIAN_POINT('Ctrl Pts',(-11.4356146405844,6.59855410763732,2.9467600778321));
#68838=CARTESIAN_POINT('Ctrl Pts',(-11.3364607606109,4.38720752303357,5.7425361490316));
#68839=CARTESIAN_POINT('Ctrl Pts',(-11.2373068806376,1.10843296602187,7.14112649578979));
#68840=CARTESIAN_POINT('Ctrl Pts',(-11.1381530006641,-2.44002848110766,
6.80224759051522));
#68841=CARTESIAN_POINT('Ctrl Pts',(-11.0389991206907,-5.39481966298761,
4.80835024454017));
#68842=CARTESIAN_POINT('Ctrl Pts',(-10.9398452407172,-7.03702615774369,
1.64455894568363));
#68843=CARTESIAN_POINT('Ctrl Pts',(-10.8406913607438,-6.9670914959007,-1.91936118496661));
#68844=CARTESIAN_POINT('Ctrl Pts',(-10.7415374807704,-5.20203110557652,
-5.01629182236644));
#68845=CARTESIAN_POINT('Ctrl Pts',(-10.6423836007969,-2.17129237981159,
-6.89273535484788));
#68846=CARTESIAN_POINT('Ctrl Pts',(-10.5432297208235,1.38773186929381,-7.09214435340263));
#68847=CARTESIAN_POINT('Ctrl Pts',(-10.4440758408501,4.60911450751237,-5.56600168228627));
#68848=CARTESIAN_POINT('Ctrl Pts',(-10.3449219608766,6.70907817315371,-2.68562494348715));
#68849=CARTESIAN_POINT('Ctrl Pts',(-10.2457680809032,7.17669195041253,0.848176820865036));
#68850=CARTESIAN_POINT('Ctrl Pts',(-10.1466142009297,5.89818323485443,4.17561322426439));
#68851=CARTESIAN_POINT('Ctrl Pts',(-10.0474603209563,3.18461913663593,6.48710353124882));
#68852=CARTESIAN_POINT('Ctrl Pts',(-9.94830644098287,-0.303777592543674,
7.22025141147022));
#68853=CARTESIAN_POINT('Ctrl Pts',(-9.84915256100942,-3.71826382217565,
6.19667857963189));
#68854=CARTESIAN_POINT('Ctrl Pts',(-9.749998681036,-6.22807918966268,3.66542506100721));
#68855=CARTESIAN_POINT('Ctrl Pts',(-9.65084480106256,-7.22257395606273,
0.242356596306747));
#68856=CARTESIAN_POINT('Ctrl Pts',(-9.55169092108911,-6.45978292451376,
-3.23967835420889));
#68857=CARTESIAN_POINT('Ctrl Pts',(-9.45253704111569,-4.12529669674559,
-5.9334845103353));
#68858=CARTESIAN_POINT('Ctrl Pts',(-9.35338316114224,-0.787106617467268,
-7.18364631947511));
#68859=CARTESIAN_POINT('Ctrl Pts',(-9.25422928116881,2.7425901585595,-6.68599360549662));
#68860=CARTESIAN_POINT('Ctrl Pts',(-9.15507540119538,5.60500200755747,-4.56160758569233));
#68861=CARTESIAN_POINT('Ctrl Pts',(-9.05592152122194,7.1036908285498,-1.3273612480958));
#68862=CARTESIAN_POINT('Ctrl Pts',(-8.9567676412485,6.87401866882103,2.22983824778147));
#68863=CARTESIAN_POINT('Ctrl Pts',(-8.85761376127506,4.97186583183785,5.24450773865122));
#68864=CARTESIAN_POINT('Ctrl Pts',(-8.75845988130163,1.86003493980857,6.98316413191473));
#68865=CARTESIAN_POINT('Ctrl Pts',(-8.65930600132819,-1.7043510943762,7.02278424968813));
#68866=CARTESIAN_POINT('Ctrl Pts',(-8.56015212135476,-4.85406058927098,
5.35372833325108));
#68867=CARTESIAN_POINT('Ctrl Pts',(-8.46099824138132,-6.82275459193258,
2.38208544112758));
#68868=CARTESIAN_POINT('Ctrl Pts',(-8.36184436140789,-7.13144070540802,
-1.16912990545044));
#68869=CARTESIAN_POINT('Ctrl Pts',(-8.26269048143445,-5.70501416420314,
-4.43589051452024));
#68870=CARTESIAN_POINT('Ctrl Pts',(-8.16353660146102,-2.89053117264693,
-6.62337835326697));
#68871=CARTESIAN_POINT('Ctrl Pts',(-8.06438272148757,0.627231481965904,
-7.19936746795161));
#68872=CARTESIAN_POINT('Ctrl Pts',(-7.96522884151415,3.99238580304136,-6.02371703105673));
#68873=CARTESIAN_POINT('Ctrl Pts',(-7.8660749615407,6.38617411051875,-3.38246825568388));
#68874=CARTESIAN_POINT('Ctrl Pts',(-7.76692108156728,7.22617658819175,0.0817507604764866));
#68875=CARTESIAN_POINT('Ctrl Pts',(-7.66776720159382,6.30801673078173,3.52607943681746));
#68876=CARTESIAN_POINT('Ctrl Pts',(-7.56861332162041,3.85508709715878,6.11249660481615));
#68877=CARTESIAN_POINT('Ctrl Pts',(-7.46945944164694,0.46419686293761,7.21171495159147));
#68878=CARTESIAN_POINT('Ctrl Pts',(-7.37030556167353,-3.03963462458951,
6.55628954665409));
#68879=CARTESIAN_POINT('Ctrl Pts',(-7.27115168170008,-5.80390888650157,
4.30568843598292));
#68880=CARTESIAN_POINT('Ctrl Pts',(-7.17199780172666,-7.15606515268471,
1.00749332558613));
#68881=CARTESIAN_POINT('Ctrl Pts',(-7.07284392175321,-6.76711752176552,
-2.53582959151107));
#68882=CARTESIAN_POINT('Ctrl Pts',(-6.97369004177979,-4.731698759309,-5.46217338810503));
#68883=CARTESIAN_POINT('Ctrl Pts',(-6.87453616180633,-1.54503570631433,
-7.05954502335547));
#68884=CARTESIAN_POINT('Ctrl Pts',(-6.77538228183291,2.01754171191176,-6.93929655737995));
#68885=CARTESIAN_POINT('Ctrl Pts',(-6.67622840185947,5.08924185858894,-5.13068500059742));
#68886=CARTESIAN_POINT('Ctrl Pts',(-6.57707452188604,6.92270581760909,-2.07375394717175));
#68887=CARTESIAN_POINT('Ctrl Pts',(-6.47792064191259,7.07184328988527,1.48773107579087));
#68888=CARTESIAN_POINT('Ctrl Pts',(-6.37876676193917,5.50036843555384,4.68724421635273));
#68889=CARTESIAN_POINT('Ctrl Pts',(-6.27961288196572,2.59062838738908,6.74632906320341));
#68890=CARTESIAN_POINT('Ctrl Pts',(-6.18045900199229,-0.949423582898823,
7.16400070706338));
#68891=CARTESIAN_POINT('Ctrl Pts',(-6.08130512201885,-4.25847638466099,
5.83863769657389));
#68892=CARTESIAN_POINT('Ctrl Pts',(-5.98215124204542,-6.53142209812059,
3.09270700952272));
#68893=CARTESIAN_POINT('Ctrl Pts',(-5.88299736207198,-7.21524247160315,
-0.405693660959992));
#68894=CARTESIAN_POINT('Ctrl Pts',(-5.78384348209854,-6.14356083136612,
-3.80538717897051));
#68895=CARTESIAN_POINT('Ctrl Pts',(-5.68468960212512,-3.57712229926877,
-6.27921231737256));
#68896=CARTESIAN_POINT('Ctrl Pts',(-5.58553572215167,-0.140353293261173,
-7.22527592716291));
#68897=CARTESIAN_POINT('Ctrl Pts',(-5.48638184217824,3.3305643210464,-6.4133963368828));
#68898=CARTESIAN_POINT('Ctrl Pts',(-5.3872279622048,5.99114016299764,-4.04110762265567));
#68899=CARTESIAN_POINT('Ctrl Pts',(-5.28807408223137,7.19404376981442,-0.685598649767781));
#68900=CARTESIAN_POINT('Ctrl Pts',(-5.18892020225793,6.64660310554116,2.83671965974429));
#68901=CARTESIAN_POINT('Ctrl Pts',(-5.08976632228449,4.48201302708057,5.66885089728502));
#68902=CARTESIAN_POINT('Ctrl Pts',(-4.99061244231105,1.22692835671624,7.12172437532194));
#68903=CARTESIAN_POINT('Ctrl Pts',(-4.89145856233762,-2.32667368286776,
6.84184922692832));
#68904=CARTESIAN_POINT('Ctrl Pts',(-4.79230468236418,-5.31418520621231,
4.89732037594473));
#68905=CARTESIAN_POINT('Ctrl Pts',(-4.69315080239075,-7.0087307803873,1.7612507256551));
#68906=CARTESIAN_POINT('Ctrl Pts',(-4.5939969224173,-6.99801959472198,-1.80333940855744));
#68907=CARTESIAN_POINT('Ctrl Pts',(-4.49484304244388,-5.28465773045043,
-4.92916868676245));
#68908=CARTESIAN_POINT('Ctrl Pts',(-4.39568916247043,-2.28551408904019,
-6.85570832367946));
#68909=CARTESIAN_POINT('Ctrl Pts',(-4.29653528249701,1.26970574821316,-7.11422227538074));
#68910=CARTESIAN_POINT('Ctrl Pts',(-4.19738140252356,4.51600027816159,-5.64181289642023));
#68911=CARTESIAN_POINT('Ctrl Pts',(-4.09822752255013,6.6635309601212,-2.79672422917872));
#68912=CARTESIAN_POINT('Ctrl Pts',(-3.9990736425767,7.1897936022312,0.728820435967838));
#68913=CARTESIAN_POINT('Ctrl Pts',(-3.89991976260326,5.96674605876947,4.07703970310913));
#68914=CARTESIAN_POINT('Ctrl Pts',(-3.80076588262982,3.29196147906146,6.43329626948305));
#68915=CARTESIAN_POINT('Ctrl Pts',(-3.70161200265639,-0.183772622207902,
7.22430196585773));
#68916=CARTESIAN_POINT('Ctrl Pts',(-3.60245812268295,-3.61479399072821,
6.25760143147231));
#68917=CARTESIAN_POINT('Ctrl Pts',(-3.50330424270951,-6.16631918779205,
3.768397397414));
#68918=CARTESIAN_POINT('Ctrl Pts',(-3.40415036273608,-7.21755027914701,
0.362324769446019));
#68919=CARTESIAN_POINT('Ctrl Pts',(-3.30499648276264,-6.51271785648537,
-3.13190315820678));
#68920=CARTESIAN_POINT('Ctrl Pts',(-3.20584260278921,-4.22331092273221,
-5.86412449735678));
#68921=CARTESIAN_POINT('Ctrl Pts',(-3.10668872281577,-0.906352820934512,
-7.16957710290872));
#68922=CARTESIAN_POINT('Ctrl Pts',(-3.00753484284234,2.63112513290601,-6.73063829109539));
#68923=CARTESIAN_POINT('Ctrl Pts',(-2.9083809628689,5.52843811830046,-4.65410391404099));
#68924=CARTESIAN_POINT('Ctrl Pts',(-2.80922708289546,7.08065642564394,-1.44520443279018));
#68925=CARTESIAN_POINT('Ctrl Pts',(-2.71007320292203,6.9101181295059,2.11532000105019));
#68926=CARTESIAN_POINT('Ctrl Pts',(-2.61091932294859,5.05831598961895,5.16117725133854));
#68927=CARTESIAN_POINT('Ctrl Pts',(-2.51176544297515,1.97580206966993,6.95129609871836));
#68928=CARTESIAN_POINT('Ctrl Pts',(-2.41261156300172,-1.58743367295767,
7.05013231113639));
#68929=CARTESIAN_POINT('Ctrl Pts',(-2.31345768302828,-4.76443942809818,
5.43363857894068));
#68930=CARTESIAN_POINT('Ctrl Pts',(-2.21430380305484,-6.78223493587843,
2.4951153370374));
#68931=CARTESIAN_POINT('Ctrl Pts',(-2.11514992308141,-7.1498811750356,-1.05048105810653));
#68932=CARTESIAN_POINT('Ctrl Pts',(-2.01599604310797,-5.77792810758181,
-4.34049053151657));
#68933=CARTESIAN_POINT('Ctrl Pts',(-1.91684216313454,-3.00017828861109,
-6.57443849367501));
#68934=CARTESIAN_POINT('Ctrl Pts',(-1.8176882831611,0.50752884612595,-7.20879502697359));
#68935=CARTESIAN_POINT('Ctrl Pts',(-1.71853440318767,3.89175185473677,-6.08921823978432));
#68936=CARTESIAN_POINT('Ctrl Pts',(-1.61938052321423,6.32909355689451,-3.48810636572991));
#68937=CARTESIAN_POINT('Ctrl Pts',(-1.52022664324079,7.22653739312793,-0.0383220079431006));
#68938=CARTESIAN_POINT('Ctrl Pts',(-1.42107276326736,6.36573110876114,3.42078627241163));
#68939=CARTESIAN_POINT('Ctrl Pts',(-1.32191888329392,3.95611287189113,6.04760136049213));
#68940=CARTESIAN_POINT('Ctrl Pts',(-1.22276500332049,0.58395399408771,7.2030069417819));
#68941=CARTESIAN_POINT('Ctrl Pts',(-1.12361112334705,-2.93028360339495,
6.60588747060103));
#68942=CARTESIAN_POINT('Ctrl Pts',(-1.02445724337361,-5.7315695867392,4.40152488836941));
#68943=CARTESIAN_POINT('Ctrl Pts',(-0.925303363400176,-7.13833806205865,
1.12625085231209));
#68944=CARTESIAN_POINT('Ctrl Pts',(-0.826149483426741,-6.80831572378113,
-2.42304524841852));
#68945=CARTESIAN_POINT('Ctrl Pts',(-0.726995603453303,-4.82179854001844,
-5.38280318329076));
#68946=CARTESIAN_POINT('Ctrl Pts',(-0.627841723479869,-1.66211537048783,
-7.03290009638678));
#68947=CARTESIAN_POINT('Ctrl Pts',(-0.528687843506433,1.90196819049315,
-6.97185974277461));
#68948=CARTESIAN_POINT('Ctrl Pts',(-0.429533963532995,5.0032940546147,-5.21453352406773));
#68949=CARTESIAN_POINT('Ctrl Pts',(-0.330380083559562,6.88729523108016,
-2.18848707341619));
#68950=CARTESIAN_POINT('Ctrl Pts',(-0.231226203586123,7.09558548101365,
1.37002844941164));
#68951=CARTESIAN_POINT('Ctrl Pts',(-0.132072323612686,5.57748681893721,
4.59520968565645));
#68952=CARTESIAN_POINT('Ctrl Pts',(-0.0329184436392514,2.70235970207573,
6.70235505708003));
#68953=CARTESIAN_POINT('Ctrl Pts',(0.0662354363341854,-0.830264084850464,
7.17878630549598));
#68954=CARTESIAN_POINT('Ctrl Pts',(0.165389316307623,-4.16088076271409,
5.90858549477325));
#68955=CARTESIAN_POINT('Ctrl Pts',(0.264543196281057,-6.47913582050193,
3.20079838322534));
#68956=CARTESIAN_POINT('Ctrl Pts',(0.363697076254494,-7.22098703256748,
-0.285757845143952));
#68957=CARTESIAN_POINT('Ctrl Pts',(0.462850956227929,-6.20593855254291,
-3.70278786222361));
#68958=CARTESIAN_POINT('Ctrl Pts',(0.562004836201364,-3.68095639130301,
-6.21891239011249));
#68959=CARTESIAN_POINT('Ctrl Pts',(0.661158716174802,-0.260380439171297,
-7.22194664183183));
#68960=CARTESIAN_POINT('Ctrl Pts',(0.760312596148235,3.22354728347921,-6.46784772406888));
#68961=CARTESIAN_POINT('Ctrl Pts',(0.859466476121674,5.92317097619031,-4.14009140688773));
#68962=CARTESIAN_POINT('Ctrl Pts',(0.95862035609511,7.18165965268664,-0.805031616485985));
#68963=CARTESIAN_POINT('Ctrl Pts',(1.05777423606855,6.69281717132386,2.72589610620094));
#68964=CARTESIAN_POINT('Ctrl Pts',(1.15692811604198,4.5755811788688,5.59360064235469));
#68965=CARTESIAN_POINT('Ctrl Pts',(1.25608199601542,1.34508502848351,7.10035615562477));
#68966=CARTESIAN_POINT('Ctrl Pts',(1.35523587598886,-2.2126765582915,6.87956202958854));
#68967=CARTESIAN_POINT('Ctrl Pts',(1.45438975596229,-5.2320836588412,4.98493850086998));
#68968=CARTESIAN_POINT('Ctrl Pts',(1.55354363593573,-6.97850049812194,1.87745627599714));
#68969=CARTESIAN_POINT('Ctrl Pts',(1.65269751590916,-7.02701574568049,-1.68681978306143));
#68970=CARTESIAN_POINT('Ctrl Pts',(1.7518513958826,-5.36582541639512,-4.84068475231937));
#68971=CARTESIAN_POINT('Ctrl Pts',(1.85100527585604,-2.39910483489405,-6.81678863261558));
#68972=CARTESIAN_POINT('Ctrl Pts',(1.95015915582947,1.15132909863318,-7.13433616934397));
#68973=CARTESIAN_POINT('Ctrl Pts',(2.04931303580291,4.42163931364934,-5.71606657156472));
#68974=CARTESIAN_POINT('Ctrl Pts',(2.14846691577634,6.61614414172214,-2.90705142137611));
#68975=CARTESIAN_POINT('Ctrl Pts',(2.24762079574978,7.20091036301022,0.609262845134264));
#68976=CARTESIAN_POINT('Ctrl Pts',(2.34677467572321,6.03366163918308,3.97734063092661));
#68977=CARTESIAN_POINT('Ctrl Pts',(2.44592855569666,3.39839500752044,6.37771296339286));
#68978=CARTESIAN_POINT('Ctrl Pts',(2.54508243567008,-0.0637169176436377,
7.22635810245902));
#68979=CARTESIAN_POINT('Ctrl Pts',(2.64423631564353,-3.51032622073068,6.31679674317765));
#68980=CARTESIAN_POINT('Ctrl Pts',(2.74339019561696,-6.10285684613524,3.87032938987749));
#68981=CARTESIAN_POINT('Ctrl Pts',(2.8425440755904,-7.21053404838757,0.482192915348399));
#68982=CARTESIAN_POINT('Ctrl Pts',(2.94169795556383,-6.56385481816304,-3.02326333564373));
#68983=CARTESIAN_POINT('Ctrl Pts',(3.04085183553727,-4.32015921649977,-5.79314557167872));
#68984=CARTESIAN_POINT('Ctrl Pts',(3.14000571551071,-1.02534880698369,-7.15352857648482));
#68985=CARTESIAN_POINT('Ctrl Pts',(3.23915959548414,2.51893373081034,-6.77342484496287));
#68986=CARTESIAN_POINT('Ctrl Pts',(3.33831347545758,5.45034798950191,-4.7453153808664));
#68987=CARTESIAN_POINT('Ctrl Pts',(3.43746735543101,7.05566726127222,-1.56264863894891));
#68988=CARTESIAN_POINT('Ctrl Pts',(3.53662123540445,6.94430990933893,2.00021777653919));
#68989=CARTESIAN_POINT('Ctrl Pts',(3.63577511537789,5.14336969479104,5.07642191443079));
#68990=CARTESIAN_POINT('Ctrl Pts',(3.73492899535132,2.09102373854355,6.91750901665076));
#68991=CARTESIAN_POINT('Ctrl Pts',(3.83408287532475,-1.47007800765708,7.07553403791758));
#68992=CARTESIAN_POINT('Ctrl Pts',(3.9332367552982,-4.67350294505472,5.51204875648353));
#68993=CARTESIAN_POINT('Ctrl Pts',(4.03239063527163,-6.73984290367638,2.60745640477422));
#68994=CARTESIAN_POINT('Ctrl Pts',(4.13154451524507,-7.16634777246096,-0.93154220368205));
#68995=CARTESIAN_POINT('Ctrl Pts',(4.2306983952185,-5.84924693419187,-4.24389226660731));
#68996=CARTESIAN_POINT('Ctrl Pts',(4.32985227519194,-3.10899714408849,-6.52368362421285));
#68997=CARTESIAN_POINT('Ctrl Pts',(4.42900615516538,0.387686097825344,-7.21623244983844));
#68998=CARTESIAN_POINT('Ctrl Pts',(4.52816003513881,3.79004350530718,-6.15303839283771));
#68999=CARTESIAN_POINT('Ctrl Pts',(4.62731391511224,6.27026573136093,-3.59278151428031));
#69000=CARTESIAN_POINT('Ctrl Pts',(4.72646779508569,7.22490315325883,-0.158384192290982));
#69001=CARTESIAN_POINT('Ctrl Pts',(4.82562167505912,6.42168811431263,3.31454872059966));
#69002=CARTESIAN_POINT('Ctrl Pts',(4.92477555503256,4.0560464428859,5.98103656772639));
#69003=CARTESIAN_POINT('Ctrl Pts',(5.023929435006,0.703549984439801,7.19231036051555));
#69004=CARTESIAN_POINT('Ctrl Pts',(5.12308331497942,-2.8201237558501,6.65366176598889));
#69005=CARTESIAN_POINT('Ctrl Pts',(5.22223719495288,-5.65764769969538,4.49614608664009));
#69006=CARTESIAN_POINT('Ctrl Pts',(5.3213910749263,-7.11864080686008,1.24469769095677));
#69007=CARTESIAN_POINT('Ctrl Pts',(5.42054495489974,-6.84763334052093,-2.30959243204915));
#69008=CARTESIAN_POINT('Ctrl Pts',(5.51969883487318,-4.91056911767337,-5.30194605677284));
#69009=CARTESIAN_POINT('Ctrl Pts',(5.61885271484661,-1.77873238950342,-7.0043153110442));
#69010=CARTESIAN_POINT('Ctrl Pts',(5.71800659482005,1.78586226417951,-7.00249487356092));
#69011=CARTESIAN_POINT('Ctrl Pts',(5.81716047479348,4.91597917714289,-5.29694891391728));
#69012=CARTESIAN_POINT('Ctrl Pts',(5.91631435476692,6.84995578487968,-2.30260353804152));
#69013=CARTESIAN_POINT('Ctrl Pts',(6.01546823474035,7.11742203170536,1.25192340196377));
#69014=CARTESIAN_POINT('Ctrl Pts',(6.11462211471379,5.65296202589422,4.5019536122408));
#69015=CARTESIAN_POINT('Ctrl Pts',(6.21377599468722,2.81354810058851,6.65643758041471));
#69016=CARTESIAN_POINT('Ctrl Pts',(6.31292987466067,-0.711297331913398,
7.19179029486994));
#69017=CARTESIAN_POINT('Ctrl Pts',(6.37903246130962,-2.94446110243687,6.38148070295211));
#69018=CARTESIAN_POINT('Ctrl Pts',(6.4120837546341,-3.89708022703547,5.73404348641072));
#69019=CARTESIAN_POINT('',(6.,6.90110124345015,0.667252526942056));
#69020=CARTESIAN_POINT('Ctrl Pts',(6.,6.90110124345015,0.667252526942055));
#69021=CARTESIAN_POINT('Ctrl Pts',(6.,6.87512084914595,0.845079749951139));
#69022=CARTESIAN_POINT('Ctrl Pts',(6.,6.8422227909989,1.02164116641632));
#69023=CARTESIAN_POINT('Ctrl Pts',(6.,6.80237868150643,1.19653215063161));
#69024=CARTESIAN_POINT('Ctrl Pts',(6.,6.76059281023488,1.37994626744993));
#69025=CARTESIAN_POINT('Ctrl Pts',(6.,6.71116752238872,1.56152391244805));
#69026=CARTESIAN_POINT('Ctrl Pts',(6.,6.65432880950473,1.74083702432569));
#69027=CARTESIAN_POINT('Ctrl Pts',(6.,6.61860356983375,1.85354196736429));
#69028=CARTESIAN_POINT('Ctrl Pts',(6.,6.57994859237711,1.96535194631467));
#69029=CARTESIAN_POINT('Ctrl Pts',(6.,6.53841065439784,2.07615582015086));
#69030=CARTESIAN_POINT('Ctrl Pts',(6.,6.51423804398105,2.14063708728189));
#69031=CARTESIAN_POINT('Ctrl Pts',(6.,6.48908897520853,2.20477755420385));
#69032=CARTESIAN_POINT('Ctrl Pts',(6.,6.46297163102309,2.26855457840167));
#69033=CARTESIAN_POINT('Ctrl Pts',(6.,6.45029733594765,2.29950446434633));
#69034=CARTESIAN_POINT('Ctrl Pts',(6.00000000000001,6.43739500160117,2.33036875102595));
#69035=CARTESIAN_POINT('Ctrl Pts',(6.00000000000001,6.42426550165052,2.36114479888992));
#69036=CARTESIAN_POINT('Ctrl Pts',(6.00000000000001,6.41370848887882,2.38589083884451));
#69037=CARTESIAN_POINT('Ctrl Pts',(6.,6.40300509881027,2.41057855434172));
#69038=CARTESIAN_POINT('Ctrl Pts',(6.,6.3921608998279,2.43519538126747));
#69039=CARTESIAN_POINT('Ctrl Pts',(6.,6.31690021844114,2.60604056504019));
#69040=CARTESIAN_POINT('Ctrl Pts',(6.,6.23479842551277,2.77362133337677));
#69041=CARTESIAN_POINT('Ctrl Pts',(6.,6.14608035170904,2.93752067517517));
#69042=CARTESIAN_POINT('Ctrl Pts',(6.,6.05778543340776,3.10063827199919));
#69043=CARTESIAN_POINT('Ctrl Pts',(6.00000000000001,5.96293679676374,3.26011007278674));
#69044=CARTESIAN_POINT('Ctrl Pts',(6.00000000000001,5.86171344922557,3.4154964720103));
#69045=CARTESIAN_POINT('Ctrl Pts',(6.00000000000001,5.77251333828363,3.55242618621861));
#69046=CARTESIAN_POINT('Ctrl Pts',(6.,5.67836217835066,3.6861832393832));
#69047=CARTESIAN_POINT('Ctrl Pts',(6.,5.57935844247498,3.81644275297445));
#69048=CARTESIAN_POINT('Ctrl Pts',(6.,5.56179714751913,3.83954820166029));
#69049=CARTESIAN_POINT('Ctrl Pts',(6.,5.54408311980832,3.86254353976059));
#69050=CARTESIAN_POINT('Ctrl Pts',(6.,5.52621684224323,3.88542686726127));
#69051=CARTESIAN_POINT('Ctrl Pts',(6.,5.5120906212318,3.90351988862925));
#69052=CARTESIAN_POINT('Ctrl Pts',(6.,5.49787159919033,3.9215397938568));
#69053=CARTESIAN_POINT('Ctrl Pts',(6.,5.48356530754569,3.9394793139752));
#69054=CARTESIAN_POINT('Ctrl Pts',(6.,5.41395857010921,4.02676339133329));
#69055=CARTESIAN_POINT('Ctrl Pts',(6.00000000000001,5.34225042088021,4.112191032286));
#69056=CARTESIAN_POINT('Ctrl Pts',(6.00000000000001,5.26848862833751,4.19567458971719));
#69057=CARTESIAN_POINT('Ctrl Pts',(6.00000000000001,5.14726642343806,4.33287381652286));
#69058=CARTESIAN_POINT('Ctrl Pts',(6.00000000000001,5.02049957218978,4.46482444068325));
#69059=CARTESIAN_POINT('Ctrl Pts',(6.,4.88860267407126,4.59129948324502));
#69060=CARTESIAN_POINT('Ctrl Pts',(6.,4.75596452769754,4.71848530373989));
#69061=CARTESIAN_POINT('Ctrl Pts',(6.00000000000001,4.61813790255797,4.84013424195775));
#69062=CARTESIAN_POINT('Ctrl Pts',(6.00000000000001,4.47551055286989,4.95597518165141));
#69063=CARTESIAN_POINT('Ctrl Pts',(6.,4.33223183470951,5.07234515828002));
#69064=CARTESIAN_POINT('Ctrl Pts',(6.,4.18410782009949,5.18285439570423));
#69065=CARTESIAN_POINT('Ctrl Pts',(6.,4.03150680793832,5.28718112877869));
#69066=CARTESIAN_POINT('Ctrl Pts',(6.,3.91705604881744,5.36542617858453));
#69067=CARTESIAN_POINT('Ctrl Pts',(6.,3.80008641070901,5.44019264427881));
#69068=CARTESIAN_POINT('Ctrl Pts',(6.,3.68074738017099,5.51132537150878));
#69069=CARTESIAN_POINT('Ctrl Pts',(6.,3.64726712747172,5.53128147197407));
#69070=CARTESIAN_POINT('Ctrl Pts',(6.,3.6136003658972,5.55095146610427));
#69071=CARTESIAN_POINT('Ctrl Pts',(6.,3.57975035326996,5.57033167451751));
#69072=CARTESIAN_POINT('Ctrl Pts',(6.,3.56056135851451,5.58131798408544));
#69073=CARTESIAN_POINT('Ctrl Pts',(5.99999999999999,3.54131353286354,5.59221107875469));
#69074=CARTESIAN_POINT('Ctrl Pts',(5.99999999999999,3.52202007761294,5.60300338569058));
#69075=CARTESIAN_POINT('Ctrl Pts',(5.99999999999999,3.36376168596919,5.69152942292001));
#69076=CARTESIAN_POINT('Ctrl Pts',(5.99999999999999,3.20222425639891,5.7733994532117));
#69077=CARTESIAN_POINT('Ctrl Pts',(5.99999999999999,3.03778929826304,5.84837571003259));
#69078=CARTESIAN_POINT('Ctrl Pts',(5.99999999999999,2.87948768288287,5.9205553894904));
#69079=CARTESIAN_POINT('Ctrl Pts',(6.,2.7184999884668,5.98634601537609));
#69080=CARTESIAN_POINT('Ctrl Pts',(6.,2.55514743307005,6.0454940255894));
#69081=CARTESIAN_POINT('Ctrl Pts',(6.,2.38509059043805,6.10706957817509));
#69082=CARTESIAN_POINT('Ctrl Pts',(6.,2.21247016466867,6.16144647749524));
#69083=CARTESIAN_POINT('Ctrl Pts',(6.00000000000001,2.03775930492053,6.20856933932807));
#69084=CARTESIAN_POINT('Ctrl Pts',(6.00000000000001,1.86371390683491,6.25551271341741));
#69085=CARTESIAN_POINT('Ctrl Pts',(6.,1.68759322518328,6.29525721624741));
#69086=CARTESIAN_POINT('Ctrl Pts',(6.,1.50986401183211,6.32769663740758));
#69087=CARTESIAN_POINT('Ctrl Pts',(6.,1.42166905351582,6.34379412269477));
#69088=CARTESIAN_POINT('Ctrl Pts',(6.,1.33307805394327,6.35809195955199));
#69089=CARTESIAN_POINT('Ctrl Pts',(6.,1.24414881613908,6.37057241832403));
#69090=CARTESIAN_POINT('Ctrl Pts',(6.,1.21992034554203,6.37397267717997));
#69091=CARTESIAN_POINT('Ctrl Pts',(6.00000000000001,1.1956667730464,6.37723801904711));
#69092=CARTESIAN_POINT('Ctrl Pts',(6.00000000000001,1.17138927881511,6.38036804447858));
#69093=CARTESIAN_POINT('Ctrl Pts',(6.00000000000001,1.15206171036832,6.38285989063826));
#69094=CARTESIAN_POINT('Ctrl Pts',(6.,1.13272121299246,6.38526565950859));
#69095=CARTESIAN_POINT('Ctrl Pts',(6.,1.1133772217241,6.38758422312348));
#69096=CARTESIAN_POINT('Ctrl Pts',(6.,0.935876273983282,6.40885942084931));
#69097=CARTESIAN_POINT('Ctrl Pts',(6.,0.757869165584463,6.42282400107153));
#69098=CARTESIAN_POINT('Ctrl Pts',(6.,0.579814660575315,6.42946647010954));
#69099=CARTESIAN_POINT('Ctrl Pts',(6.,0.401928577292704,6.43610265603719));
#69100=CARTESIAN_POINT('Ctrl Pts',(6.,0.223994448325209,6.43543058097201));
#69101=CARTESIAN_POINT('Ctrl Pts',(6.,0.0464678143495036,6.42738694530138));
#69102=CARTESIAN_POINT('Ctrl Pts',(6.,-0.128897738801852,6.41944122703288));
#69103=CARTESIAN_POINT('Ctrl Pts',(6.00000000000001,-0.303866334909319,
6.40430224928206));
#69104=CARTESIAN_POINT('Ctrl Pts',(6.00000000000001,-0.477990242294203,
6.38185908387302));
#69105=CARTESIAN_POINT('Ctrl Pts',(6.00000000000001,-0.528330376469423,
6.37537064713291));
#69106=CARTESIAN_POINT('Ctrl Pts',(6.00000000000001,-0.578599818986257,
6.36827139495402));
#69107=CARTESIAN_POINT('Ctrl Pts',(6.00000000000001,-0.628787491712748,
6.36055786920434));
#69108=CARTESIAN_POINT('Ctrl Pts',(6.00000000000001,-0.758270673288377,
6.34065712862454));
#69109=CARTESIAN_POINT('Ctrl Pts',(6.00000000000001,-0.887210108491146,
6.31666852198741));
#69110=CARTESIAN_POINT('Ctrl Pts',(6.00000000000001,-1.0154256226731,6.28864626423226));
#69111=CARTESIAN_POINT('Ctrl Pts',(6.00000000000001,-1.0715199101277,6.27638652646438));
#69112=CARTESIAN_POINT('Ctrl Pts',(6.00000000000001,-1.12747553722447,6.26335455099811));
#69113=CARTESIAN_POINT('Ctrl Pts',(6.00000000000001,-1.18327691273108,6.24955409931957));
#69114=CARTESIAN_POINT('Ctrl Pts',(6.00000000000001,-1.21645335177475,6.2413491072431));
#69115=CARTESIAN_POINT('Ctrl Pts',(6.00000000000001,-1.24957525908693,6.23287246231486));
#69116=CARTESIAN_POINT('Ctrl Pts',(6.00000000000001,-1.28263929909211,6.22412487911342));
#69117=CARTESIAN_POINT('Ctrl Pts',(6.00000000000001,-1.30830712007077,6.21733407558259));
#69118=CARTESIAN_POINT('Ctrl Pts',(6.00000000000001,-1.33394273334406,6.21037917995715));
#69119=CARTESIAN_POINT('Ctrl Pts',(6.00000000000001,-1.35952145145008,6.20326713279195));
#69120=CARTESIAN_POINT('Ctrl Pts',(6.00000000000001,-1.52810164644578,6.15639417016115));
#69121=CARTESIAN_POINT('Ctrl Pts',(6.00000000000001,-1.69441995109146,6.10264583742032));
#69122=CARTESIAN_POINT('Ctrl Pts',(6.00000000000001,-1.85808244723373,6.04224631836195));
#69123=CARTESIAN_POINT('Ctrl Pts',(6.00000000000001,-2.02266743867339,5.98150635311946));
#69124=CARTESIAN_POINT('Ctrl Pts',(6.,-2.18456727282551,5.9140397073175));
#69125=CARTESIAN_POINT('Ctrl Pts',(6.,-2.34336323590439,5.84002531164617));
#69126=CARTESIAN_POINT('Ctrl Pts',(6.,-2.50120497939138,5.76645567530665));
#69127=CARTESIAN_POINT('Ctrl Pts',(6.00000000000001,-2.65598065856633,5.68641637359828));
#69128=CARTESIAN_POINT('Ctrl Pts',(6.00000000000001,-2.80725163501019,5.60003997452776));
#69129=CARTESIAN_POINT('Ctrl Pts',(6.,-2.95558268225547,5.51534228808054));
#69130=CARTESIAN_POINT('Ctrl Pts',(6.,-3.10054441261676,5.42455102216784));
#69131=CARTESIAN_POINT('Ctrl Pts',(6.,-3.24168883972874,5.32775543156938));
#69132=CARTESIAN_POINT('Ctrl Pts',(6.,-3.32787899344155,5.26864699205739));
#69133=CARTESIAN_POINT('Ctrl Pts',(6.,-3.41264498807892,5.20729889266937));
#69134=CARTESIAN_POINT('Ctrl Pts',(6.,-3.49587713861109,5.14372565308808));
#69135=CARTESIAN_POINT('Ctrl Pts',(5.35582833639373,-6.93262081645922,0.000142250729870931));
#69136=CARTESIAN_POINT('Ctrl Pts',(5.3774005425624,-6.93206096538092,-0.75173178625728));
#69137=CARTESIAN_POINT('Ctrl Pts',(5.39897274873107,-6.81015446000589,-1.50378293313638));
#69138=CARTESIAN_POINT('Ctrl Pts',(5.42054495489974,-6.56995721443619,-2.21593634900211));
#69139=CARTESIAN_POINT('Ctrl Pts',(5.45359624822422,-6.20194526623841,-3.30704364029038));
#69140=CARTESIAN_POINT('Ctrl Pts',(5.4866475415487,-5.5562571919559,-4.3044948485316));
#69141=CARTESIAN_POINT('Ctrl Pts',(5.51969883487318,-4.71144036678631,-5.08694866169745));
#69142=CARTESIAN_POINT('Ctrl Pts',(5.55275012819765,-3.86662354161672,-5.8694024748633));
#69143=CARTESIAN_POINT('Ctrl Pts',(5.58580142152213,-2.82267796556008,-6.43685889295375));
#69144=CARTESIAN_POINT('Ctrl Pts',(5.61885271484661,-1.70660606858459,-6.72028369575176));
#69145=CARTESIAN_POINT('Ctrl Pts',(5.65190400817109,-0.590534171609124,
-7.00370849854977));
#69146=CARTESIAN_POINT('Ctrl Pts',(5.68495530149557,0.597664046285246,-7.00310168605534));
#69147=CARTESIAN_POINT('Ctrl Pts',(5.71800659482005,1.71344930739295,-6.71854061986752));
#69148=CARTESIAN_POINT('Ctrl Pts',(5.75105788814453,2.82923456850066,-6.4339795536797));
#69149=CARTESIAN_POINT('Ctrl Pts',(5.784109181469,3.87260687282175,-5.8654642337985));
#69150=CARTESIAN_POINT('Ctrl Pts',(5.81716047479348,4.7166224596051,-5.08214901121195));
#69151=CARTESIAN_POINT('Ctrl Pts',(5.85021176811796,5.56063804638848,-4.29883378862537));
#69152=CARTESIAN_POINT('Ctrl Pts',(5.88326306144244,6.20529691563407,-3.30071866333345));
#69153=CARTESIAN_POINT('Ctrl Pts',(5.91631435476692,6.57220405806116,-2.20923994401993));
#69154=CARTESIAN_POINT('Ctrl Pts',(5.94420956984461,6.88187283716353,-1.28803443084786));
#69155=CARTESIAN_POINT('Ctrl Pts',(5.9721047849223,6.99369014720255,-0.300323033281158));
#69156=CARTESIAN_POINT('Ctrl Pts',(6.,6.90110124345015,0.667252526942056));
#69157=CARTESIAN_POINT('',(-13.617,-3.61129923637168,-5.06367012420432));
#69158=CARTESIAN_POINT('Ctrl Pts',(-13.617,-3.61129923637173,-5.06367012420428));
#69159=CARTESIAN_POINT('Ctrl Pts',(-13.617,-3.74821940074788,-4.9772215892196));
#69160=CARTESIAN_POINT('Ctrl Pts',(-13.617,-3.88155875406187,-4.8855130775753));
#69161=CARTESIAN_POINT('Ctrl Pts',(-13.617,-4.01098648203258,-4.78872019092777));
#69162=CARTESIAN_POINT('Ctrl Pts',(-13.617,-4.14999389329108,-4.68476311146675));
#69163=CARTESIAN_POINT('Ctrl Pts',(-13.617,-4.28449018187927,-4.57494160616014));
#69164=CARTESIAN_POINT('Ctrl Pts',(-13.617,-4.41423794256447,-4.4596577141252));
#69165=CARTESIAN_POINT('Ctrl Pts',(-13.617,-4.49638395135372,-4.38666908173302));
#69166=CARTESIAN_POINT('Ctrl Pts',(-13.617,-4.57662608008218,-4.31148992041847));
#69167=CARTESIAN_POINT('Ctrl Pts',(-13.617,-4.65489813141777,-4.23421332941955));
#69168=CARTESIAN_POINT('Ctrl Pts',(-13.617,-4.70991755617827,-4.17989363916403));
#69169=CARTESIAN_POINT('Ctrl Pts',(-13.617,-4.76396345962384,-4.12453745736493));
#69170=CARTESIAN_POINT('Ctrl Pts',(-13.617,-4.81701125140619,-4.06817532341179));
#69171=CARTESIAN_POINT('Ctrl Pts',(-13.617,-4.84235650451882,-4.04124653895131));
#69172=CARTESIAN_POINT('Ctrl Pts',(-13.617,-4.86747747607571,-4.01408402234033));
#69173=CARTESIAN_POINT('Ctrl Pts',(-13.617,-4.89235012235299,-3.9867147784119));
#69174=CARTESIAN_POINT('Ctrl Pts',(-13.617,-5.01128793420523,-3.8558385560507));
#69175=CARTESIAN_POINT('Ctrl Pts',(-13.617,-5.12463251721525,-3.72015406049308));
#69176=CARTESIAN_POINT('Ctrl Pts',(-13.617,-5.23214095883406,-3.58007840859063));
#69177=CARTESIAN_POINT('Ctrl Pts',(-13.617,-5.34000106729645,-3.43954456046075));
#69178=CARTESIAN_POINT('Ctrl Pts',(-13.617,-5.4419873053284,-3.29459024569057));
#69179=CARTESIAN_POINT('Ctrl Pts',(-13.617,-5.53782072571578,-3.14559625945889));
#69180=CARTESIAN_POINT('Ctrl Pts',(-13.617,-5.61942688539801,-3.01872165785366));
#69181=CARTESIAN_POINT('Ctrl Pts',(-13.617,-5.69657110816774,-2.88891693505272));
#69182=CARTESIAN_POINT('Ctrl Pts',(-13.617,-5.76905775679567,-2.75639865042115));
#69183=CARTESIAN_POINT('Ctrl Pts',(-13.617,-5.78080653204021,-2.73491983230224));
#69184=CARTESIAN_POINT('Ctrl Pts',(-13.617,-5.79243289965685,-2.71336969612923));
#69185=CARTESIAN_POINT('Ctrl Pts',(-13.617,-5.80393596649487,-2.69174912918771));
#69186=CARTESIAN_POINT('Ctrl Pts',(-13.617,-5.81531874733626,-2.67035464555759));
#69187=CARTESIAN_POINT('Ctrl Pts',(-13.617,-5.82657684846509,-2.64889857665108));
#69188=CARTESIAN_POINT('Ctrl Pts',(-13.617,-5.83770783831778,-2.62738549567325));
#69189=CARTESIAN_POINT('Ctrl Pts',(-13.617,-5.88472903406521,-2.53650671443489));
#69190=CARTESIAN_POINT('Ctrl Pts',(-13.617,-5.92949293450927,-2.44459071409149));
#69191=CARTESIAN_POINT('Ctrl Pts',(-13.617,-5.97195499129405,-2.3517149301572));
#69192=CARTESIAN_POINT('Ctrl Pts',(-13.617,-6.04516132784387,-2.19159324951219));
#69193=CARTESIAN_POINT('Ctrl Pts',(-13.617,-6.11152842057772,-2.02862056578686));
#69194=CARTESIAN_POINT('Ctrl Pts',(-13.617,-6.17107314357316,-1.86327271702071));
#69195=CARTESIAN_POINT('Ctrl Pts',(-13.617,-6.23139190661368,-1.69577546105483));
#69196=CARTESIAN_POINT('Ctrl Pts',(-13.617,-6.2847100279,-1.52584027291554));
#69197=CARTESIAN_POINT('Ctrl Pts',(-13.617,-6.33100000828456,-1.35393263393096));
#69198=CARTESIAN_POINT('Ctrl Pts',(-13.617,-6.37823410871505,-1.17851880534197));
#69199=CARTESIAN_POINT('Ctrl Pts',(-13.617,-6.41815081170317,-1.00105057130705));
#69200=CARTESIAN_POINT('Ctrl Pts',(-13.617,-6.45066957280197,-0.822002128173549));
#69201=CARTESIAN_POINT('Ctrl Pts',(-13.617,-6.47505864362608,-0.687715795823425));
#69202=CARTESIAN_POINT('Ctrl Pts',(-13.617,-6.4952853305009,-0.552540099903254));
#69203=CARTESIAN_POINT('Ctrl Pts',(-13.617,-6.5112955086982,-0.416671418134875));
#69204=CARTESIAN_POINT('Ctrl Pts',(-13.617,-6.51564948719698,-0.379721840698151));
#69205=CARTESIAN_POINT('Ctrl Pts',(-13.617,-6.51969152334182,-0.342721004431168));
#69206=CARTESIAN_POINT('Ctrl Pts',(-13.617,-6.52342029919769,-0.305672850016471));
#69207=CARTESIAN_POINT('Ctrl Pts',(-13.617,-6.52548275285274,-0.285180842870193));
#69208=CARTESIAN_POINT('Ctrl Pts',(-13.617,-6.52744895761689,-0.264678160216595));
#69209=CARTESIAN_POINT('Ctrl Pts',(-13.617,-6.52931811777843,-0.244173644297405));
#69210=CARTESIAN_POINT('Ctrl Pts',(-13.617,-6.54586442705464,-0.062662145744726));
#69211=CARTESIAN_POINT('Ctrl Pts',(-13.617,-6.55482935469237,0.119181209939556));
#69212=CARTESIAN_POINT('Ctrl Pts',(-13.617,-6.55620696958347,0.300870273217915));
#69213=CARTESIAN_POINT('Ctrl Pts',(-13.617,-6.55749612429352,0.470892616328059));
#69214=CARTESIAN_POINT('Ctrl Pts',(-13.617,-6.55214075841214,0.640780576326433));
#69215=CARTESIAN_POINT('Ctrl Pts',(-13.617,-6.54009687944681,0.810149061967126));
#69216=CARTESIAN_POINT('Ctrl Pts',(-13.617,-6.52728479397343,0.990320543328873));
#69217=CARTESIAN_POINT('Ctrl Pts',(-13.617,-6.5069044992998,1.16990477407658));
#69218=CARTESIAN_POINT('Ctrl Pts',(-13.617,-6.47915416231961,1.34847769329285));
#69219=CARTESIAN_POINT('Ctrl Pts',(-13.617,-6.45125503441877,1.52800807940656));
#69220=CARTESIAN_POINT('Ctrl Pts',(-13.617,-6.41590648915762,1.7065169794788));
#69221=CARTESIAN_POINT('Ctrl Pts',(-13.617,-6.37325744722561,1.88356902905038));
#69222=CARTESIAN_POINT('Ctrl Pts',(-13.617,-6.3513454550729,1.97453386542391));
#69223=CARTESIAN_POINT('Ctrl Pts',(-13.617,-6.32750555767679,2.06511400851921));
#69224=CARTESIAN_POINT('Ctrl Pts',(-13.617,-6.30175278232589,2.15524902944258));
#69225=CARTESIAN_POINT('Ctrl Pts',(-13.617,-6.29423752239852,2.1815525288351));
#69226=CARTESIAN_POINT('Ctrl Pts',(-13.617,-6.28655933789324,2.20781811305338));
#69227=CARTESIAN_POINT('Ctrl Pts',(-13.617,-6.27871854750472,2.23404425858231));
#69228=CARTESIAN_POINT('Ctrl Pts',(-13.617,-6.27182667314066,2.25709643713613));
#69229=CARTESIAN_POINT('Ctrl Pts',(-13.617,-6.26481116263825,2.2801113732589));
#69230=CARTESIAN_POINT('Ctrl Pts',(-13.617,-6.25767498527291,2.30308018036077));
#69231=CARTESIAN_POINT('Ctrl Pts',(-13.617,-6.20307361309252,2.47882250302214));
#69232=CARTESIAN_POINT('Ctrl Pts',(-13.617,-6.1413695380144,2.6520078842564));
#69233=CARTESIAN_POINT('Ctrl Pts',(-13.617,-6.07280403431614,2.82220755207323));
#69234=CARTESIAN_POINT('Ctrl Pts',(-13.617,-6.00377201206077,2.99356525562474));
#69235=CARTESIAN_POINT('Ctrl Pts',(-13.617,-5.92778472312197,3.16189718654644));
#69236=CARTESIAN_POINT('Ctrl Pts',(-13.617,-5.84503562544626,3.32676190057267));
#69237=CARTESIAN_POINT('Ctrl Pts',(-13.617,-5.76244833580976,3.49130423723336));
#69238=CARTESIAN_POINT('Ctrl Pts',(-13.617,-5.67312543976135,3.65239361081794));
#69239=CARTESIAN_POINT('Ctrl Pts',(-13.617,-5.57720973772646,3.80957671010982));
#69240=CARTESIAN_POINT('Ctrl Pts',(-13.617,-5.55089861053992,3.85269441064586));
#69241=CARTESIAN_POINT('Ctrl Pts',(-13.617,-5.52409110541491,3.89551805044802));
#69242=CARTESIAN_POINT('Ctrl Pts',(-13.617,-5.49678954957014,3.93803797214658));
#69243=CARTESIAN_POINT('Ctrl Pts',(-13.617,-5.41998906945479,4.05764838627403));
#69244=CARTESIAN_POINT('Ctrl Pts',(-13.617,-5.33928015461665,4.17485620063647));
#69245=CARTESIAN_POINT('Ctrl Pts',(-13.617,-5.25481751197263,4.2895246234203));
#69246=CARTESIAN_POINT('Ctrl Pts',(-13.617,-5.21786510581587,4.33969205838822));
#69247=CARTESIAN_POINT('Ctrl Pts',(-13.617,-5.1801940180667,4.38937329875199));
#69248=CARTESIAN_POINT('Ctrl Pts',(-13.617,-5.14181633873687,4.43855619232835));
#69249=CARTESIAN_POINT('Ctrl Pts',(-13.617,-5.12064999833221,4.46568190408848));
#69250=CARTESIAN_POINT('Ctrl Pts',(-13.617,-5.09926871628423,4.49265601958829));
#69251=CARTESIAN_POINT('Ctrl Pts',(-13.617,-5.07767445742497,4.51947643921585));
#69252=CARTESIAN_POINT('Ctrl Pts',(-13.617,-5.0623536077347,4.53850518293992));
#69253=CARTESIAN_POINT('Ctrl Pts',(-13.617,-5.04692457910768,4.55745765964485));
#69254=CARTESIAN_POINT('Ctrl Pts',(-13.617,-5.03139997187395,4.57631887404553));
#69255=CARTESIAN_POINT('Ctrl Pts',(-13.617,-4.91417163799297,4.71874236379161));
#69256=CARTESIAN_POINT('Ctrl Pts',(-13.617,-4.79135007651547,4.85614873648681));
#69257=CARTESIAN_POINT('Ctrl Pts',(-13.617,-4.66335466830376,4.98829842572615));
#69258=CARTESIAN_POINT('Ctrl Pts',(-13.617,-4.5330631770047,5.12281872083878));
#69259=CARTESIAN_POINT('Ctrl Pts',(-13.617,-4.39741019028498,5.25189260637322));
#69260=CARTESIAN_POINT('Ctrl Pts',(-13.617,-4.25678987213029,5.37524320479101));
#69261=CARTESIAN_POINT('Ctrl Pts',(-13.617,-4.11589880764864,5.49883129891275));
#69262=CARTESIAN_POINT('Ctrl Pts',(-13.617,-3.97002076950435,5.61667457298439));
#69263=CARTESIAN_POINT('Ctrl Pts',(-13.617,-3.81951090759404,5.72846233525811));
#69264=CARTESIAN_POINT('Ctrl Pts',(-13.617,-3.67054101929963,5.83910631730177));
#69265=CARTESIAN_POINT('Ctrl Pts',(-13.617,-3.51703305935551,5.94381851790106));
#69266=CARTESIAN_POINT('Ctrl Pts',(-13.617,-3.359298849805,6.04225900678258));
#69267=CARTESIAN_POINT('Ctrl Pts',(-13.617,-3.2483339549443,6.1115111907565));
#69268=CARTESIAN_POINT('Ctrl Pts',(-13.617,-3.13527679518198,6.17765870225568));
#69269=CARTESIAN_POINT('Ctrl Pts',(-13.617,-3.02022829989065,6.2405696868587));
#69270=CARTESIAN_POINT('Ctrl Pts',(-13.617,-3.61129923637168,-5.06367012420432));
#69271=CARTESIAN_POINT('Ctrl Pts',(-13.5891047849223,-2.90091050768866,
-5.56924680684122));
#69272=CARTESIAN_POINT('Ctrl Pts',(-13.5281582765201,-1.11449490138686,
-6.34652636371273));
#69273=CARTESIAN_POINT('Ctrl Pts',(-13.4341604747935,1.91301075045669,-6.193982915654));
#69274=CARTESIAN_POINT('Ctrl Pts',(-13.33500659482,4.64114599103167,-4.52598857637084));
#69275=CARTESIAN_POINT('Ctrl Pts',(-13.2358527148466,6.24006591576224,-1.75683043852266));
#69276=CARTESIAN_POINT('Ctrl Pts',(-13.1366988348732,6.3207503286919,1.43978832745216));
#69277=CARTESIAN_POINT('Ctrl Pts',(-13.0375449548997,4.86356603929123,4.28609183779942));
#69278=CARTESIAN_POINT('Ctrl Pts',(-12.9383910749263,2.2230539416448,6.08957345749443));
#69279=CARTESIAN_POINT('Ctrl Pts',(-12.8392371949529,-0.958337716508845,
6.41143141299502));
#69280=CARTESIAN_POINT('Ctrl Pts',(-12.7400833149794,-3.90656124824087,
5.17335943056773));
#69281=CARTESIAN_POINT('Ctrl Pts',(-12.6457560560753,-5.80705422041825,
2.79812271529996));
#69282=CARTESIAN_POINT('Ctrl Pts',(-12.5844800904956,-6.21868878492818,
0.882080331722138));
#69283=CARTESIAN_POINT('Ctrl Pts',(-12.5562554182404,-6.21952031151782,
-0.000132913339471047));
#69284=CARTESIAN_POINT('Origin',(-13.617,-1.12618006296016E-15,0.));
#69285=CARTESIAN_POINT('',(-13.617,-6.933,-8.4904762584886E-16));
#69286=CARTESIAN_POINT('Origin',(-13.617,0.,0.));
#69287=CARTESIAN_POINT('Origin',(-13.617,0.,0.));
#69288=CARTESIAN_POINT('',(-13.617,3.61104546693872,-5.06353840690493));
#69289=CARTESIAN_POINT('Ctrl Pts',(-13.617,3.02048254223756,6.24076191290031));
#69290=CARTESIAN_POINT('Ctrl Pts',(-13.617,3.17824519336757,6.15468957050444));
#69291=CARTESIAN_POINT('Ctrl Pts',(-13.617,3.33242025106992,6.06256863353936));
#69292=CARTESIAN_POINT('Ctrl Pts',(-13.617,3.48261838037657,5.96451288457896));
#69293=CARTESIAN_POINT('Ctrl Pts',(-13.617,3.64013626193522,5.86167848895641));
#69294=CARTESIAN_POINT('Ctrl Pts',(-13.617,3.79328089376711,5.75231661468439));
#69295=CARTESIAN_POINT('Ctrl Pts',(-13.617,3.94172923226954,5.63678774775573));
#69296=CARTESIAN_POINT('Ctrl Pts',(-13.617,4.03503451979194,5.56417356928354));
#69297=CARTESIAN_POINT('Ctrl Pts',(-13.617,4.12648382947108,5.48912224730297));
#69298=CARTESIAN_POINT('Ctrl Pts',(-13.617,4.2159891579907,5.41171621830808));
#69299=CARTESIAN_POINT('Ctrl Pts',(-13.617,4.26807594012178,5.3666705094707));
#69300=CARTESIAN_POINT('Ctrl Pts',(-13.617,4.31950426551617,5.32082727289711));
#69301=CARTESIAN_POINT('Ctrl Pts',(-13.617,4.37025573807922,5.27420203999897));
#69302=CARTESIAN_POINT('Ctrl Pts',(-13.617,4.39488454444256,5.25157562593252));
#69303=CARTESIAN_POINT('Ctrl Pts',(-13.617,4.41935394043864,5.22876504499028));
#69304=CARTESIAN_POINT('Ctrl Pts',(-13.617,4.44366175369453,5.20577203247252));
#69305=CARTESIAN_POINT('Ctrl Pts',(-13.617,4.46320689558227,5.18728408016865));
#69306=CARTESIAN_POINT('Ctrl Pts',(-13.617,4.48264654393124,5.16867908441253));
#69307=CARTESIAN_POINT('Ctrl Pts',(-13.617,4.50197084753761,5.14996662735338));
#69308=CARTESIAN_POINT('Ctrl Pts',(-13.617,4.6360849691378,5.02009883016965));
#69309=CARTESIAN_POINT('Ctrl Pts',(-13.617,4.76476363751091,4.8849477516844));
#69310=CARTESIAN_POINT('Ctrl Pts',(-13.617,4.88769376982304,4.74486895472631));
#69311=CARTESIAN_POINT('Ctrl Pts',(-13.617,5.01003756789948,4.60545828520619));
#69312=CARTESIAN_POINT('Ctrl Pts',(-13.617,5.12668795564162,4.46116620848808));
#69313=CARTESIAN_POINT('Ctrl Pts',(-13.617,5.23729475898094,4.31231315172846));
#69314=CARTESIAN_POINT('Ctrl Pts',(-13.617,5.3347637657555,4.18114075401248));
#69315=CARTESIAN_POINT('Ctrl Pts',(-13.617,5.42753922720179,4.04642585709307));
#69316=CARTESIAN_POINT('Ctrl Pts',(-13.617,5.51535062192892,3.90837354772389));
#69317=CARTESIAN_POINT('Ctrl Pts',(-13.617,5.53092661714939,3.88388581332916));
#69318=CARTESIAN_POINT('Ctrl Pts',(-13.617,5.5463463451654,3.85929304469139));
#69319=CARTESIAN_POINT('Ctrl Pts',(-13.617,5.56160819159072,3.83459635400809));
#69320=CARTESIAN_POINT('Ctrl Pts',(-13.617,5.57367518302917,3.81506957155148));
#69321=CARTESIAN_POINT('Ctrl Pts',(-13.617,5.58564139940011,3.79548112560944));
#69322=CARTESIAN_POINT('Ctrl Pts',(-13.617,5.59750194280488,3.77583872625322));
#69323=CARTESIAN_POINT('Ctrl Pts',(-13.617,5.65520898570643,3.68026934602712));
#69324=CARTESIAN_POINT('Ctrl Pts',(-13.617,5.71044575082297,3.58337330982993));
#69325=CARTESIAN_POINT('Ctrl Pts',(-13.617,5.76314661286957,3.48522583142202));
#69326=CARTESIAN_POINT('Ctrl Pts',(-13.617,5.8497566907193,3.32392750696295));
#69327=CARTESIAN_POINT('Ctrl Pts',(-13.617,5.92952029322569,3.15925032066695));
#69328=CARTESIAN_POINT('Ctrl Pts',(-13.617,6.0023684100752,2.99166187481058));
#69329=CARTESIAN_POINT('Ctrl Pts',(-13.617,6.07562592405362,2.82313160325521));
#69330=CARTESIAN_POINT('Ctrl Pts',(-13.617,6.14189018518748,2.65165654249902));
#69331=CARTESIAN_POINT('Ctrl Pts',(-13.617,6.20104147301423,2.47769443325878));
#69332=CARTESIAN_POINT('Ctrl Pts',(-13.617,6.2604629017156,2.30293784805581));
#69333=CARTESIAN_POINT('Ctrl Pts',(-13.617,6.31270642666534,2.12567071291085));
#69334=CARTESIAN_POINT('Ctrl Pts',(-13.617,6.35759807452877,1.94635009739155));
#69335=CARTESIAN_POINT('Ctrl Pts',(-13.617,6.39126681042635,1.81185963575207));
#69336=CARTESIAN_POINT('Ctrl Pts',(-13.617,6.42079905049903,1.67621387994155));
#69337=CARTESIAN_POINT('Ctrl Pts',(-13.617,6.44610115240018,1.53960686779479));
#69338=CARTESIAN_POINT('Ctrl Pts',(-13.617,6.45319959001507,1.50128213266926));
#69339=CARTESIAN_POINT('Ctrl Pts',(-13.617,6.45996497978633,1.46288175683764));
#69340=CARTESIAN_POINT('Ctrl Pts',(-13.617,6.466395001408,1.42441007246538));
#69341=CARTESIAN_POINT('Ctrl Pts',(-13.617,6.47004007180214,1.40260112593786));
#69342=CARTESIAN_POINT('Ctrl Pts',(-13.617,6.47357730478795,1.38076934970857));
#69343=CARTESIAN_POINT('Ctrl Pts',(-13.617,6.47700417893135,1.35892975260253));
#69344=CARTESIAN_POINT('Ctrl Pts',(-13.617,6.50511378819952,1.1797861612311));
#69345=CARTESIAN_POINT('Ctrl Pts',(-13.617,6.52584313224597,0.999876921866305));
#69346=CARTESIAN_POINT('Ctrl Pts',(-13.617,6.53910160122101,0.81964234584923));
#69347=CARTESIAN_POINT('Ctrl Pts',(-13.617,6.55186553820663,0.646130398486221));
#69348=CARTESIAN_POINT('Ctrl Pts',(-13.617,6.5577053299578,0.472316286598931));
#69349=CARTESIAN_POINT('Ctrl Pts',(-13.617,6.55649463142021,0.298589257555608));
#69350=CARTESIAN_POINT('Ctrl Pts',(-13.617,6.55523424373395,0.117732172676484));
#69351=CARTESIAN_POINT('Ctrl Pts',(-13.617,6.54633292198605,-0.0630312575838317));
#69352=CARTESIAN_POINT('Ctrl Pts',(-13.617,6.52990290843545,-0.243238067897483));
#69353=CARTESIAN_POINT('Ctrl Pts',(-13.617,6.51353547205042,-0.422758522635574));
#69354=CARTESIAN_POINT('Ctrl Pts',(-13.617,6.48969633624267,-0.601727290924061));
#69355=CARTESIAN_POINT('Ctrl Pts',(-13.617,6.45844785533837,-0.779669770145348));
#69356=CARTESIAN_POINT('Ctrl Pts',(-13.617,6.44294135723537,-0.867970533466823));
#69357=CARTESIAN_POINT('Ctrl Pts',(-13.617,6.42560960552124,-0.956018249370113));
#69358=CARTESIAN_POINT('Ctrl Pts',(-13.617,6.40645603012195,-1.0437525546006));
#69359=CARTESIAN_POINT('Ctrl Pts',(-13.617,6.40123761064567,-1.06765589366958));
#69360=CARTESIAN_POINT('Ctrl Pts',(-13.617,6.39588394211369,-1.09153595774107));
#69361=CARTESIAN_POINT('Ctrl Pts',(-13.617,6.3903950594231,-1.11539150131513));
#69362=CARTESIAN_POINT('Ctrl Pts',(-13.617,6.38602531807229,-1.13438308140121));
#69363=CARTESIAN_POINT('Ctrl Pts',(-13.617,6.38157035926579,-1.15335691703556));
#69364=CARTESIAN_POINT('Ctrl Pts',(-13.617,6.37703239899045,-1.17230376852458));
#69365=CARTESIAN_POINT('Ctrl Pts',(-13.617,6.33539254634327,-1.34615811194329));
#69366=CARTESIAN_POINT('Ctrl Pts',(-13.617,6.2867206860848,-1.51795037154905));
#69367=CARTESIAN_POINT('Ctrl Pts',(-13.617,6.23116523195699,-1.68724630323634));
#69368=CARTESIAN_POINT('Ctrl Pts',(-13.617,6.17566231906677,-1.85638212431142));
#69369=CARTESIAN_POINT('Ctrl Pts',(-13.617,6.1132885745343,-2.02302703146196));
#69370=CARTESIAN_POINT('Ctrl Pts',(-13.617,6.0441427066901,-2.18673182669575));
#69371=CARTESIAN_POINT('Ctrl Pts',(-13.617,5.97583855230202,-2.3484438415469));
#69372=CARTESIAN_POINT('Ctrl Pts',(-13.617,5.90092583665929,-2.50728749672662));
#69373=CARTESIAN_POINT('Ctrl Pts',(-13.617,5.81945588920982,-2.66280439039303));
#69374=CARTESIAN_POINT('Ctrl Pts',(-13.617,5.79590290227599,-2.70776437231505));
#69375=CARTESIAN_POINT('Ctrl Pts',(-13.617,5.77180160189991,-2.75244611117256));
#69376=CARTESIAN_POINT('Ctrl Pts',(-13.617,5.74715258895802,-2.79683801784677));
#69377=CARTESIAN_POINT('Ctrl Pts',(-13.617,5.6835575761326,-2.91137014458735));
#69378=CARTESIAN_POINT('Ctrl Pts',(-13.617,5.61631738202126,-3.02397382199317));
#69379=CARTESIAN_POINT('Ctrl Pts',(-13.617,5.54554537288572,-3.13449888198446));
#69380=CARTESIAN_POINT('Ctrl Pts',(-13.617,5.51458261888893,-3.18285359573065));
#69381=CARTESIAN_POINT('Ctrl Pts',(-13.617,5.48294372620547,-3.23081029824356));
#69382=CARTESIAN_POINT('Ctrl Pts',(-13.617,5.45063763270645,-3.27835567218871));
#69383=CARTESIAN_POINT('Ctrl Pts',(-13.617,5.4314302006912,-3.30662354486477));
#69384=CARTESIAN_POINT('Ctrl Pts',(-13.617,5.41198691778349,-3.33474601054841));
#69385=CARTESIAN_POINT('Ctrl Pts',(-13.617,5.39230961159509,-3.36272018885805));
#69386=CARTESIAN_POINT('Ctrl Pts',(-13.617,5.37703399546923,-3.38443671881408));
#69387=CARTESIAN_POINT('Ctrl Pts',(-13.617,5.36161565934957,-3.40606610228615));
#69388=CARTESIAN_POINT('Ctrl Pts',(-13.617,5.34606967910636,-3.42758759414123));
#69389=CARTESIAN_POINT('Ctrl Pts',(-13.617,5.24361164791509,-3.56942809884234));
#69390=CARTESIAN_POINT('Ctrl Pts',(-13.617,5.13549032829701,-3.70676149773043));
#69391=CARTESIAN_POINT('Ctrl Pts',(-13.617,5.0220526626288,-3.83929613750716));
#69392=CARTESIAN_POINT('Ctrl Pts',(-13.617,4.90797564391624,-3.9725777639653));
#69393=CARTESIAN_POINT('Ctrl Pts',(-13.617,4.78852166418632,-4.10100691347751));
#69394=CARTESIAN_POINT('Ctrl Pts',(-13.617,4.66400382821274,-4.22425297526121));
#69395=CARTESIAN_POINT('Ctrl Pts',(-13.617,4.54023426066734,-4.34675841112407));
#69396=CARTESIAN_POINT('Ctrl Pts',(-13.617,4.41146095294851,-4.46414331471841));
#69397=CARTESIAN_POINT('Ctrl Pts',(-13.617,4.27796044161972,-4.57604230105919));
#69398=CARTESIAN_POINT('Ctrl Pts',(-13.617,4.14705452965938,-4.6857665164092));
#69399=CARTESIAN_POINT('Ctrl Pts',(-13.617,4.01160282440768,-4.79021629205608));
#69400=CARTESIAN_POINT('Ctrl Pts',(-13.617,3.87184448414395,-4.88900244664526));
#69401=CARTESIAN_POINT('Ctrl Pts',(-13.617,3.78650057188512,-4.94932655248207));
#69402=CARTESIAN_POINT('Ctrl Pts',(-13.617,3.69955034012038,-5.00753781673398));
#69403=CARTESIAN_POINT('Ctrl Pts',(-13.617,3.61104546693877,-5.0635384069049));
#69404=CARTESIAN_POINT('Origin',(-13.617,0.,0.));
#69405=CARTESIAN_POINT('Origin',(-15.9277445817596,0.,0.));
#69406=CARTESIAN_POINT('Ctrl Pts',(-13.617,3.61104546693871,-5.06353840690493));
#69407=CARTESIAN_POINT('Ctrl Pts',(-13.5839487066755,4.45227095397745,-4.46362126645189));
#69408=CARTESIAN_POINT('Ctrl Pts',(-13.5178461200266,5.82912718297219,-2.83706456600194));
#69409=CARTESIAN_POINT('Ctrl Pts',(-13.4186922400531,6.47593427309586,0.295071888562534));
#69410=CARTESIAN_POINT('Ctrl Pts',(-13.3195383600797,5.54718661553207,3.35454744289073));
#69411=CARTESIAN_POINT('Ctrl Pts',(-13.2203844801062,3.26875126278153,5.59827586641925));
#69412=CARTESIAN_POINT('Ctrl Pts',(-13.1212306001328,0.195029276623322,
6.47969774398204));
#69413=CARTESIAN_POINT('Ctrl Pts',(-13.0220767201594,-2.92615231197546,
5.78469244453168));
#69414=CARTESIAN_POINT('Ctrl Pts',(-12.9229228401859,-5.33538328621662,
3.6821860861499));
#69415=CARTESIAN_POINT('Ctrl Pts',(-12.849812127386,-6.15465544744627,1.47135071718486));
#69416=CARTESIAN_POINT('Ctrl Pts',(-12.8097527079106,-6.21953641508352,
0.219232564831544));
#69417=CARTESIAN_POINT('Ctrl Pts',(-12.8027445817596,-6.21931067987726,
0.000159553896288585));
#69418=CARTESIAN_POINT('Ctrl Pts',(-14.0290837546341,4.02546580733783,-5.64465357962329));
#69419=CARTESIAN_POINT('Ctrl Pts',(-13.9960324613096,4.96323423627052,-4.9758871632932));
#69420=CARTESIAN_POINT('Ctrl Pts',(-13.9299298746607,6.49810487752479,-3.16265926536026));
#69421=CARTESIAN_POINT('Ctrl Pts',(-13.8307759946872,7.2191425518147,0.328935708229076));
#69422=CARTESIAN_POINT('Ctrl Pts',(-13.7316221147138,6.18380750178624,3.7395308793763));
#69423=CARTESIAN_POINT('Ctrl Pts',(-13.6324682347404,3.64388833136868,6.24075999226346));
#69424=CARTESIAN_POINT('Ctrl Pts',(-13.5333143547669,0.217411741742154,
7.22333793608995));
#69425=CARTESIAN_POINT('Ctrl Pts',(-13.4341604747935,-3.26197113461037,
6.44857060223313));
#69426=CARTESIAN_POINT('Ctrl Pts',(-13.33500659482,-5.94769663919919,4.1047708542473));
#69427=CARTESIAN_POINT('Ctrl Pts',(-13.2358527148466,-7.1863223146633,0.76229495696539));
#69428=CARTESIAN_POINT('Ctrl Pts',(-13.1366988348732,-6.67648114875678,
-2.76566822514195));
#69429=CARTESIAN_POINT('Ctrl Pts',(-13.0375449548997,-4.54222174007392,
-5.62072250746908));
#69430=CARTESIAN_POINT('Ctrl Pts',(-12.9383910749263,-1.3028183504887,-7.10823352255506));
#69431=CARTESIAN_POINT('Ctrl Pts',(-12.8392371949529,2.2535666263224,-6.86627590756217));
#69432=CARTESIAN_POINT('Ctrl Pts',(-12.7400833149794,5.26164846117041,-4.95372269926303));
#69433=CARTESIAN_POINT('Ctrl Pts',(-12.640929435006,6.98954673567817,-1.83590510727142));
#69434=CARTESIAN_POINT('Ctrl Pts',(-12.5417755550326,7.0168558409393,1.72859639764328));
#69435=CARTESIAN_POINT('Ctrl Pts',(-12.4426216750591,5.33693130930571,4.87252253811412));
#69436=CARTESIAN_POINT('Ctrl Pts',(-12.3434677950857,2.35850660217995,6.83094122079118));
#69437=CARTESIAN_POINT('Ctrl Pts',(-12.2443139151123,-1.19375372156009,
7.1273602146869));
#69438=CARTESIAN_POINT('Ctrl Pts',(-12.1451600351388,-4.45556821727479,
5.68965933289867));
#69439=CARTESIAN_POINT('Ctrl Pts',(-12.0460061551654,-6.63332226702549,
2.86763791460573));
#69440=CARTESIAN_POINT('Ctrl Pts',(-11.9468522751919,-7.19715819185692,
-0.652093136928579));
#69441=CARTESIAN_POINT('Ctrl Pts',(-11.8476983952185,-6.00989209247491,
-4.01316689555907));
#69442=CARTESIAN_POINT('Ctrl Pts',(-11.7485445152451,-3.36039132628151,
-6.39781850589597));
#69443=CARTESIAN_POINT('Ctrl Pts',(-11.6493906352716,0.106708261150547,
-7.22585115007998));
#69444=CARTESIAN_POINT('Ctrl Pts',(-11.5502367552982,3.54784523293374,-6.29580064022737));
#69445=CARTESIAN_POINT('Ctrl Pts',(-11.4510828753247,6.1257749770444,-3.8339525855188));
#69446=CARTESIAN_POINT('Ctrl Pts',(-11.3519289953513,7.21327521028865,-0.439286055197895));
#69447=CARTESIAN_POINT('Ctrl Pts',(-11.2527751153779,6.54575207362621,3.06226081323672));
#69448=CARTESIAN_POINT('Ctrl Pts',(-11.1536212354045,4.28561704737463,5.81874539921091));
#69449=CARTESIAN_POINT('Ctrl Pts',(-11.054467355431,0.982771483491727,7.15950219700309));
#69450=CARTESIAN_POINT('Ctrl Pts',(-10.9553134754576,-2.5591869480573,6.75831884883418));
#69451=CARTESIAN_POINT('Ctrl Pts',(-10.8561595954841,-5.47848330574273,
4.7128051271331));
#69452=CARTESIAN_POINT('Ctrl Pts',(-10.7570057155107,-7.06483922335105,
1.52064402337556));
#69453=CARTESIAN_POINT('Ctrl Pts',(-10.6578518355373,-6.93228693627894,
-2.04149683583503));
#69454=CARTESIAN_POINT('Ctrl Pts',(-10.5586979555638,-5.11307703177873,
-5.1069320305567));
#69455=CARTESIAN_POINT('Ctrl Pts',(-10.4595440755904,-2.04983173125164,
-6.92982693659675));
#69456=CARTESIAN_POINT('Ctrl Pts',(-10.360390195617,1.51214715254185,-7.06666275456019));
#69457=CARTESIAN_POINT('Ctrl Pts',(-10.2612363156435,4.70621360902953,-5.48414669422815));
#69458=CARTESIAN_POINT('Ctrl Pts',(-10.1620824356701,6.75523643044027,-2.5673122650899));
#69459=CARTESIAN_POINT('Ctrl Pts',(-10.0629285556967,7.16067884503,0.974161165294735));
#69460=CARTESIAN_POINT('Ctrl Pts',(-9.96377467572322,5.82389482973557,4.27861665843151));
#69461=CARTESIAN_POINT('Ctrl Pts',(-9.86462079574978,3.07013014587324,6.54206484109023));
#69462=CARTESIAN_POINT('Ctrl Pts',(-9.76546691577634,-0.430611465607748,
7.21379825496357));
#69463=CARTESIAN_POINT('Ctrl Pts',(-9.6663130358029,-3.82658330698325,6.13038103973526));
#69464=CARTESIAN_POINT('Ctrl Pts',(-9.56715915582948,-6.2915296523324,3.55541363718072));
#69465=CARTESIAN_POINT('Ctrl Pts',(-9.46800527585602,-7.22571760425057,
0.115397579055486));
#69466=CARTESIAN_POINT('Ctrl Pts',(-9.36885139588261,-6.40185489401093,
-3.3526952461649));
#69467=CARTESIAN_POINT('Ctrl Pts',(-9.26969751590916,-4.02039114649391,
-6.00506174213237));
#69468=CARTESIAN_POINT('Ctrl Pts',(-9.17054363593573,-0.660747555210352,
-7.19636881808541));
#69469=CARTESIAN_POINT('Ctrl Pts',(-9.07138975596229,2.85965898593902,-6.63676592790242));
#69470=CARTESIAN_POINT('Ctrl Pts',(-8.97223587598885,5.68429721048297,-4.46240705455296));
#69471=CARTESIAN_POINT('Ctrl Pts',(-8.87308199601543,7.12591951576202,-1.20232381350058));
#69472=CARTESIAN_POINT('Ctrl Pts',(-8.77392811604198,6.83377249745176,2.35029039709997));
#69473=CARTESIAN_POINT('Ctrl Pts',(-8.67477423606854,4.87893688235586,5.33106803517046));
#69474=CARTESIAN_POINT('Ctrl Pts',(-8.57562035609512,1.73703325734962,7.01477205335211));
#69475=CARTESIAN_POINT('Ctrl Pts',(-8.47646647612167,-1.82749862903197,
6.99174944191472));
#69476=CARTESIAN_POINT('Ctrl Pts',(-8.37731259614824,-4.94739160882633,
5.26760170917879));
#69477=CARTESIAN_POINT('Ctrl Pts',(-8.27815871617481,-6.86356122573495,
2.26182200851794));
#69478=CARTESIAN_POINT('Ctrl Pts',(-8.17900483620136,-7.10979450987494,
-1.29426949472691));
#69479=CARTESIAN_POINT('Ctrl Pts',(-8.07985095622793,-5.62618175927108,
-4.53545921702244));
#69480=CARTESIAN_POINT('Ctrl Pts',(-7.98069707625449,-2.77369284867334,
-6.67315064110252));
#69481=CARTESIAN_POINT('Ctrl Pts',(-7.88154319628106,0.753648417953927,
-7.18723351225935));
#69482=CARTESIAN_POINT('Ctrl Pts',(-7.78238931630763,4.09762352321354,-5.95262907962823));
#69483=CARTESIAN_POINT('Ctrl Pts',(-7.68323543633418,6.44462778864662,-3.26972233736018));
#69484=CARTESIAN_POINT('Ctrl Pts',(-7.58408155636075,7.22362417282433,0.20872303997529));
#69485=CARTESIAN_POINT('Ctrl Pts',(-7.48492767638731,6.24507923643584,3.63638513200491));
#69486=CARTESIAN_POINT('Ctrl Pts',(-7.38577379641388,3.74707750860212,6.17929782759794));
#69487=CARTESIAN_POINT('Ctrl Pts',(-7.28661991644044,0.337394414854048,
7.21875865412148));
#69488=CARTESIAN_POINT('Ctrl Pts',(-7.18746603646701,-3.1543783074859,6.50186196338333));
#69489=CARTESIAN_POINT('Ctrl Pts',(-7.08831215649357,-5.87867613308897,
4.20303205077935));
#69490=CARTESIAN_POINT('Ctrl Pts',(-6.98915827652014,-7.17266474451676,
0.88158491388799));
#69491=CARTESIAN_POINT('Ctrl Pts',(-6.89000439654669,-6.72151070103148,
-2.65435592819569));
#69492=CARTESIAN_POINT('Ctrl Pts',(-6.79085051657327,-4.63498187737245,
-5.54447964141429));
#69493=CARTESIAN_POINT('Ctrl Pts',(-6.69169663659982,-1.42074042987509,
-7.08560569948305));
#69494=CARTESIAN_POINT('Ctrl Pts',(-6.59254275662639,2.13917376464837,-6.90277097275208));
#69495=CARTESIAN_POINT('Ctrl Pts',(-6.49338887665296,5.17861704411722,-5.0404599996436));
#69496=CARTESIAN_POINT('Ctrl Pts',(-6.39423499667951,6.95807873807318,-1.95178169178893));
#69497=CARTESIAN_POINT('Ctrl Pts',(-6.29508111670609,7.04460754940169,1.61177416921263));
#69498=CARTESIAN_POINT('Ctrl Pts',(-6.19592723673263,5.41715061631334,4.78317788690788));
#69499=CARTESIAN_POINT('Ctrl Pts',(-6.09677335675922,2.47167577142396,6.79081220315981));
#69500=CARTESIAN_POINT('Ctrl Pts',(-5.99761947678577,-1.07516927149738,
7.14621036181109));
#69501=CARTESIAN_POINT('Ctrl Pts',(-5.89846559681234,-4.36042063567106,
5.76290233976271));
#69502=CARTESIAN_POINT('Ctrl Pts',(-5.7993117168389,-6.58476140166159,2.97745340531404));
#69503=CARTESIAN_POINT('Ctrl Pts',(-5.70015783686546,-7.20699912732122,
-0.532423775220128));
#69504=CARTESIAN_POINT('Ctrl Pts',(-5.60100395689203,-6.07574048322174,
-3.91275977772325));
#69505=CARTESIAN_POINT('Ctrl Pts',(-5.50185007691859,-3.46622595304341,
-6.34110314851262));
#69506=CARTESIAN_POINT('Ctrl Pts',(-5.40269619694516,-0.0133625451907377,
-7.22662666394319));
#69507=CARTESIAN_POINT('Ctrl Pts',(-5.30354231697172,3.44275203198619,-6.35387833876942));
#69508=CARTESIAN_POINT('Ctrl Pts',(-5.20438843699829,6.0612290455365,-3.93520189509677));
#69509=CARTESIAN_POINT('Ctrl Pts',(-5.10523455702485,7.20498087321364,-0.559072548292375));
#69510=CARTESIAN_POINT('Ctrl Pts',(-5.00608067705141,6.59572738173239,2.95308174683567));
#69511=CARTESIAN_POINT('Ctrl Pts',(-4.90692679707797,4.38170277602357,5.74673753361121));
#69512=CARTESIAN_POINT('Ctrl Pts',(-4.80777291710454,1.10158952851184,7.14218538042113));
#69513=CARTESIAN_POINT('Ctrl Pts',(-4.7086190371311,-2.44654556902168,6.79990634320274));
#69514=CARTESIAN_POINT('Ctrl Pts',(-4.60946515715767,-5.39942476351695,
4.80317850186191));
#69515=CARTESIAN_POINT('Ctrl Pts',(-4.51031127718423,-7.03859882854682,
1.63781501654116));
#69516=CARTESIAN_POINT('Ctrl Pts',(-4.4111573972108,-6.96524909885898,-1.92603647122083));
#69517=CARTESIAN_POINT('Ctrl Pts',(-4.31200351723736,-5.19722190445262,
-5.02127433760656));
#69518=CARTESIAN_POINT('Ctrl Pts',(-4.21284963726393,-2.16468647557985,
-6.89481282995197));
#69519=CARTESIAN_POINT('Ctrl Pts',(-4.11369575729048,1.39452722944346,-7.09081132903485));
#69520=CARTESIAN_POINT('Ctrl Pts',(-4.01454187731705,4.61444598088623,-5.5615824894639));
#69521=CARTESIAN_POINT('Ctrl Pts',(-3.91538799734361,6.71164858751094,-2.67919479235665));
#69522=CARTESIAN_POINT('Ctrl Pts',(-3.81623411737018,7.17587591199851,0.855053444661745));
#69523=CARTESIAN_POINT('Ctrl Pts',(-3.71708023739674,5.89417928960641,4.18126320620973));
#69524=CARTESIAN_POINT('Ctrl Pts',(-3.61792635742331,3.17840146303416,6.49015220448725));
#69525=CARTESIAN_POINT('Ctrl Pts',(-3.51877247744987,-0.310696205625941,
7.21995701963925));
#69526=CARTESIAN_POINT('Ctrl Pts',(-3.41961859747644,-3.72420004403323,
6.19311274963175));
#69527=CARTESIAN_POINT('Ctrl Pts',(-3.32046471750299,-6.23158870993929,
3.65945537584293));
#69528=CARTESIAN_POINT('Ctrl Pts',(-3.22131083752956,-7.22280289217062,
0.235435508112602));
#69529=CARTESIAN_POINT('Ctrl Pts',(-3.12215695755613,-6.45667557523428,
-3.24586691252144));
#69530=CARTESIAN_POINT('Ctrl Pts',(-3.02300307758269,-4.11960909459448,
-5.93743483377822));
#69531=CARTESIAN_POINT('Ctrl Pts',(-2.92384919760925,-0.780222582471201,
-7.18439727600238));
#69532=CARTESIAN_POINT('Ctrl Pts',(-2.82469531763581,2.74899570870432,-6.68336248389639));
#69533=CARTESIAN_POINT('Ctrl Pts',(-2.72554143766238,5.60937057274208,-4.55623455007352));
#69534=CARTESIAN_POINT('Ctrl Pts',(-2.62638755768894,7.10495951656942,-1.32055358298638));
#69535=CARTESIAN_POINT('Ctrl Pts',(-2.52723367771551,6.87187880198643,2.23642420583352));
#69536=CARTESIAN_POINT('Ctrl Pts',(-2.42807979774207,4.96683804969124,5.24926959545495));
#69537=CARTESIAN_POINT('Ctrl Pts',(-2.32892591776863,1.85334252510417,6.9849433055873));
#69538=CARTESIAN_POINT('Ctrl Pts',(-2.2297720377952,-1.71107984604937,7.02114785900938));
#69539=CARTESIAN_POINT('Ctrl Pts',(-2.13061815782176,-4.85918854137058,
5.34907451967547));
#69540=CARTESIAN_POINT('Ctrl Pts',(-2.03146427784833,-6.82503408988951,
2.37554649911859));
#69541=CARTESIAN_POINT('Ctrl Pts',(-1.93231039787489,-7.13031713677931,
-1.17596302092359));
#69542=CARTESIAN_POINT('Ctrl Pts',(-1.83315651790145,-5.70076089845598,
-4.44135527471782));
#69543=CARTESIAN_POINT('Ctrl Pts',(-1.73400263792802,-2.88418304909733,
-6.62614515664486));
#69544=CARTESIAN_POINT('Ctrl Pts',(-1.63484875795458,0.634129935366402,
-7.19876313839403));
#69545=CARTESIAN_POINT('Ctrl Pts',(-1.53569487798115,3.99815616053177,-6.01988860475261));
#69546=CARTESIAN_POINT('Ctrl Pts',(-1.43654099800771,6.38941241731386,-3.37634720653903));
#69547=CARTESIAN_POINT('Ctrl Pts',(-1.33738711803427,7.22609494920389,0.0886751527681432));
#69548=CARTESIAN_POINT('Ctrl Pts',(-1.23823323806084,6.30463500915592,3.5321224354422));
#69549=CARTESIAN_POINT('Ctrl Pts',(-1.1390793580874,3.84922808147728,6.11618792013417));
#69550=CARTESIAN_POINT('Ctrl Pts',(-1.03992547811397,0.457286078935402,
7.21215646943689));
#69551=CARTESIAN_POINT('Ctrl Pts',(-0.940771598140529,-3.04591575105879,
6.55337384368391));
#69552=CARTESIAN_POINT('Ctrl Pts',(-0.841617718167091,-5.80803212818724,
4.30012491627548));
#69553=CARTESIAN_POINT('Ctrl Pts',(-0.742463838193658,-7.157027305729,1.00063561933304));
#69554=CARTESIAN_POINT('Ctrl Pts',(-0.64330995822022,-6.76468448986276,
-2.54231297251901));
#69555=CARTESIAN_POINT('Ctrl Pts',(-0.544156078246784,-4.72646251042451,
-5.46670500714828));
#69556=CARTESIAN_POINT('Ctrl Pts',(-0.445002198273351,-1.53827024412814,
-7.06102231646795));
#69557=CARTESIAN_POINT('Ctrl Pts',(-0.345848318299913,2.02419031901898,
-6.93736009228426));
#69558=CARTESIAN_POINT('Ctrl Pts',(-0.246694438326475,5.09415597362008,
-5.1258059282477));
#69559=CARTESIAN_POINT('Ctrl Pts',(-0.147540558353041,6.92468981354721,
-2.06711936853776));
#69560=CARTESIAN_POINT('Ctrl Pts',(-0.0483866783796038,7.07041445130143,
1.49450693690473));
#69561=CARTESIAN_POINT('Ctrl Pts',(0.0507672015938331,5.49587440551356,
4.69251276145835));
#69562=CARTESIAN_POINT('Ctrl Pts',(0.149921081567267,2.58416258427939,6.74880843080014));
#69563=CARTESIAN_POINT('Ctrl Pts',(0.249074961540705,-0.95628799914268,
7.16308765549634));
#69564=CARTESIAN_POINT('Ctrl Pts',(0.348228841514144,-4.26406926967639,
5.83455437553118));
#69565=CARTESIAN_POINT('Ctrl Pts',(0.447382721487575,-6.53438267699997,
3.08644690998419));
#69566=CARTESIAN_POINT('Ctrl Pts',(0.546536601461014,-7.21485042175099,
-0.412607427693591));
#69567=CARTESIAN_POINT('Ctrl Pts',(0.645690481434445,-6.13991154033284,
-3.8112724613331));
#69568=CARTESIAN_POINT('Ctrl Pts',(0.744844361407885,-3.57110365651654,
-6.28263719882365));
#69569=CARTESIAN_POINT('Ctrl Pts',(0.843998241381321,-0.133429662532856,
-7.22540711813424));
#69570=CARTESIAN_POINT('Ctrl Pts',(0.943152121354755,3.33670838822898,-6.41020191800155));
#69571=CARTESIAN_POINT('Ctrl Pts',(1.04230600132819,5.99500978654503,-4.0353648108762));
#69572=CARTESIAN_POINT('Ctrl Pts',(1.14145988130163,7.19469745234014,-0.678704697875825));
#69573=CARTESIAN_POINT('Ctrl Pts',(1.24061376127506,6.64388180304984,2.84308742122567));
#69574=CARTESIAN_POINT('Ctrl Pts',(1.3397676412485,4.47657884511091,5.67314316240424));
#69575=CARTESIAN_POINT('Ctrl Pts',(1.43892152122194,1.22010345698743,7.12289681603459));
#69576=CARTESIAN_POINT('Ctrl Pts',(1.53807540119537,-2.33322877054477,6.83961658296214));
#69577=CARTESIAN_POINT('Ctrl Pts',(1.63722928116881,-5.31887559855225,4.89222585994902));
#69578=CARTESIAN_POINT('Ctrl Pts',(1.73638316114225,-7.01041528314337,1.75453385703958));
#69579=CARTESIAN_POINT('Ctrl Pts',(1.83553704111569,-6.9962883605478,-1.81004438445359));
#69580=CARTESIAN_POINT('Ctrl Pts',(1.93469092108911,-5.27993197666347,-4.93423041815386));
#69581=CARTESIAN_POINT('Ctrl Pts',(2.03384480106256,-2.27894361349163,-6.85789526780295));
#69582=CARTESIAN_POINT('Ctrl Pts',(2.13299868103599,1.27652231829741,-7.11300233857104));
#69583=CARTESIAN_POINT('Ctrl Pts',(2.23215256100943,4.5214044396118,-5.63748289497069));
#69584=CARTESIAN_POINT('Ctrl Pts',(2.33130644098286,6.66620785535008,-2.79033767255823));
#69585=CARTESIAN_POINT('Ctrl Pts',(2.4304603209563,7.18909193019322,0.73570966886304));
#69586=CARTESIAN_POINT('Ctrl Pts',(2.52961420092973,5.96283653953145,4.08275542990979));
#69587=CARTESIAN_POINT('Ctrl Pts',(2.62876808090317,3.28579531681644,6.43644782730468));
#69588=CARTESIAN_POINT('Ctrl Pts',(2.72792196087661,-0.190695171538537,
7.22412256604076));
#69589=CARTESIAN_POINT('Ctrl Pts',(2.82707584085004,-3.62078863873284,6.25413472282594));
#69590=CARTESIAN_POINT('Ctrl Pts',(2.92622972082349,-6.16992740875923,3.76248684625687));
#69591=CARTESIAN_POINT('Ctrl Pts',(3.02538360079691,-7.21789417615659,0.35540844033487));
#69592=CARTESIAN_POINT('Ctrl Pts',(3.12453748077035,-6.50971375778922,-3.13814249026964));
#69593=CARTESIAN_POINT('Ctrl Pts',(3.22369136074378,-4.21768973951514,-5.86816877388985));
#69594=CARTESIAN_POINT('Ctrl Pts',(3.32284524071722,-0.899482213157528,
-7.17044233265069));
#69595=CARTESIAN_POINT('Ctrl Pts',(3.42199912069066,2.63757351439253,-6.72811395961489));
#69596=CARTESIAN_POINT('Ctrl Pts',(3.52115300066409,5.5328953524373,-4.64880420294464));
#69597=CARTESIAN_POINT('Ctrl Pts',(3.62030688063753,7.0820380464371,-1.43841878635096));
#69598=CARTESIAN_POINT('Ctrl Pts',(3.71946076061097,6.90808798262623,2.12194060341662));
#69599=CARTESIAN_POINT('Ctrl Pts',(3.81861464058441,5.05336801840377,5.16602198653642));
#69600=CARTESIAN_POINT('Ctrl Pts',(3.91776852055784,1.96914014011108,6.95318621974456));
#69601=CARTESIAN_POINT('Ctrl Pts',(4.01692240053127,-1.59418868556376,7.04860794358157));
#69602=CARTESIAN_POINT('Ctrl Pts',(4.11607628050472,-4.76964399176775,5.42907060692931));
#69603=CARTESIAN_POINT('Ctrl Pts',(4.21523016047815,-6.78462276778132,2.48861517244911));
#69604=CARTESIAN_POINT('Ctrl Pts',(4.31438404045158,-7.14887128193105,-1.05733190097141));
#69605=CARTESIAN_POINT('Ctrl Pts',(4.41353792042502,-5.77376624502238,-4.3460251992502));
#69606=CARTESIAN_POINT('Ctrl Pts',(4.51269180039845,-2.9938769721112,-6.57731039820468));
#69607=CARTESIAN_POINT('Ctrl Pts',(4.6118456803719,0.514436312362811,-7.20830537738637));
#69608=CARTESIAN_POINT('Ctrl Pts',(4.71099956034533,3.897585170993,-6.08548625378336));
#69609=CARTESIAN_POINT('Ctrl Pts',(4.81015344031876,6.33243283244007,-3.48203989073616));
#69610=CARTESIAN_POINT('Ctrl Pts',(4.9093073202922,7.22657136347239,-0.031397359545163));
#69611=CARTESIAN_POINT('Ctrl Pts',(5.00846120026564,6.36244919040953,3.42688490344027));
#69612=CARTESIAN_POINT('Ctrl Pts',(5.10761508023907,3.95031806190394,6.05138897039844));
#69613=CARTESIAN_POINT('Ctrl Pts',(5.20676896021251,0.577047496600863,7.2035642704365));
#69614=CARTESIAN_POINT('Ctrl Pts',(5.30592284018594,-2.93660455179739,6.60307449482303));
#69615=CARTESIAN_POINT('Ctrl Pts',(5.40507672015939,-5.7357997190033,4.39603458568039));
#69616=CARTESIAN_POINT('Ctrl Pts',(5.50423060013282,-7.13938491615856,1.11940244029185));
#69617=CARTESIAN_POINT('Ctrl Pts',(5.60338448010626,-6.80604716325542,-2.4295533466182));
#69618=CARTESIAN_POINT('Ctrl Pts',(5.70253836007969,-4.81652869657057,-5.38745002130588));
#69619=CARTESIAN_POINT('Ctrl Pts',(5.80169224005313,-1.65559090405508,-7.03443221887737));
#69620=CARTESIAN_POINT('Ctrl Pts',(5.90084612002656,1.90909700073592,-6.97015991709384));
#69621=CARTESIAN_POINT('Ctrl Pts',(5.96694870667552,3.97444177895362,-5.79628844103034));
#69622=CARTESIAN_POINT('Ctrl Pts',(6.,4.80478746383271,-4.99805026259201));
#69623=CARTESIAN_POINT('Ctrl Pts',(-13.8917225030894,3.88732569387146,-5.4509485220505));
#69624=CARTESIAN_POINT('Ctrl Pts',(-13.8586712097649,4.79291314217283,-4.8051318643461));
#69625=CARTESIAN_POINT('Ctrl Pts',(-13.792568623116,6.27511231267392,-3.05412769890749));
#69626=CARTESIAN_POINT('Ctrl Pts',(-13.6934147431425,6.97140645890842,0.317647768340228));
#69627=CARTESIAN_POINT('Ctrl Pts',(-13.5942608631691,5.97160053970152,3.61120306721445));
#69628=CARTESIAN_POINT('Ctrl Pts',(-13.4951069831956,3.51884264183963,6.02659861698205));
#69629=CARTESIAN_POINT('Ctrl Pts',(-13.3959531032222,0.209950920035877,
6.97545787205399));
#69630=CARTESIAN_POINT('Ctrl Pts',(-13.2967992232488,-3.1500315270654,6.22727788299931));
#69631=CARTESIAN_POINT('Ctrl Pts',(-13.1976453432753,-5.743592188205,3.9639092648815));
#69632=CARTESIAN_POINT('Ctrl Pts',(-13.0984914633019,-6.93971249918703,
0.73613562115432));
#69633=CARTESIAN_POINT('Ctrl Pts',(-12.9993375833285,-6.44736732501885,
-2.67076002303153));
#69634=CARTESIAN_POINT('Ctrl Pts',(-12.900183703355,-4.38634834390208,-5.42783868181853));
#69635=CARTESIAN_POINT('Ctrl Pts',(-12.8010298233816,-1.25811011462824,
-6.86430344530502));
#69636=CARTESIAN_POINT('Ctrl Pts',(-12.7018759434082,2.17623198621772,-6.63064898179542));
#69637=CARTESIAN_POINT('Ctrl Pts',(-12.6027220634347,5.08108681930493,-4.78372800833562));
#69638=CARTESIAN_POINT('Ctrl Pts',(-12.5035681834613,6.74968957992116,-1.77290317110548));
#69639=CARTESIAN_POINT('Ctrl Pts',(-12.4044143034878,6.77606153080561,1.66927692657171));
#69640=CARTESIAN_POINT('Ctrl Pts',(-12.3052604235144,5.15378621954096,4.70531435687567));
#69641=CARTESIAN_POINT('Ctrl Pts',(-12.206106543541,2.27757078376049,6.5965268596998));
#69642=CARTESIAN_POINT('Ctrl Pts',(-12.1069526635675,-1.15278820789294,
6.88277377527959));
#69643=CARTESIAN_POINT('Ctrl Pts',(-12.0077987835941,-4.30266847136972,
5.49440983297767));
#69644=CARTESIAN_POINT('Ctrl Pts',(-11.9086449036207,-6.40568950736929,
2.76923046417301));
#69645=CARTESIAN_POINT('Ctrl Pts',(-11.8094910236473,-6.95017652641927,
-0.629715547790527));
#69646=CARTESIAN_POINT('Ctrl Pts',(-11.7103371436738,-5.80365330786967,
-3.87544883835896));
#69647=CARTESIAN_POINT('Ctrl Pts',(-11.6111832637004,-3.24507427694579,
-6.17826742370054));
#69648=CARTESIAN_POINT('Ctrl Pts',(-11.5120293837269,0.103046401378646,
-6.9778848412012));
#69649=CARTESIAN_POINT('Ctrl Pts',(-11.4128755037535,3.4260954115478,-6.0797504595955));
#69650=CARTESIAN_POINT('Ctrl Pts',(-11.3137216237801,5.91555949121022,-3.70238454580946));
#69651=CARTESIAN_POINT('Ctrl Pts',(-11.2145677438066,6.96574046432281,-0.424211271703603));
#69652=CARTESIAN_POINT('Ctrl Pts',(-11.1154138638332,6.32112442121259,2.95717457565572));
#69653=CARTESIAN_POINT('Ctrl Pts',(-11.0162599838598,4.13854943991446,5.61906611036594));
#69654=CARTESIAN_POINT('Ctrl Pts',(-10.9171061038863,0.949046153122836,
6.91381275553423));
#69655=CARTESIAN_POINT('Ctrl Pts',(-10.8179522239129,-2.47136447177597,
6.52639663726845));
#69656=CARTESIAN_POINT('Ctrl Pts',(-10.7187983439394,-5.29048063929369,
4.55107789700226));
#69657=CARTESIAN_POINT('Ctrl Pts',(-10.619644463966,-6.82239828889908,1.46846076111849));
#69658=CARTESIAN_POINT('Ctrl Pts',(-10.5204905839926,-6.69439473950172,
-1.97143970007961));
#69659=CARTESIAN_POINT('Ctrl Pts',(-10.4213367040191,-4.93761384934533,
-4.93167972338762));
#69660=CARTESIAN_POINT('Ctrl Pts',(-10.3221828240457,-1.97948857061021,
-6.6920191585307));
#69661=CARTESIAN_POINT('Ctrl Pts',(-10.2230289440723,1.46025547360891,-6.82415924280158));
#69662=CARTESIAN_POINT('Ctrl Pts',(-10.1238750640988,4.54471257708354,-5.29594967980412));
#69663=CARTESIAN_POINT('Ctrl Pts',(-10.0247211841254,6.52341999685084,-2.47921095593041));
#69664=CARTESIAN_POINT('Ctrl Pts',(-9.92556730415195,6.91494902505595,0.940731311372487));
#69665=CARTESIAN_POINT('Ctrl Pts',(-9.82641342417852,5.62403883018155,4.13178928019433));
#69666=CARTESIAN_POINT('Ctrl Pts',(-9.72725954420508,2.96477385991635,6.31756372178987));
#69667=CARTESIAN_POINT('Ctrl Pts',(-9.62810566423165,-0.415834364132817,
6.96624555990707));
#69668=CARTESIAN_POINT('Ctrl Pts',(-9.5289517842582,-3.6952681555164,5.92000748970347));
#69669=CARTESIAN_POINT('Ctrl Pts',(-9.42979790428479,-6.0756260372859,3.43340409424414));
#69670=CARTESIAN_POINT('Ctrl Pts',(-9.33064402431132,-6.97775587820442,
0.111437531839213));
#69671=CARTESIAN_POINT('Ctrl Pts',(-9.23149014433791,-6.18216529688604,
-3.23764229977566));
#69672=CARTESIAN_POINT('Ctrl Pts',(-9.13233626436446,-3.88242517789877,
-5.79898871850399));
#69673=CARTESIAN_POINT('Ctrl Pts',(-9.03318238439104,-0.638072976262717,
-6.94941424123515));
#69674=CARTESIAN_POINT('Ctrl Pts',(-8.93402850441759,2.76152534484023,-6.40901499367288));
#69675=CARTESIAN_POINT('Ctrl Pts',(-8.83487462444415,5.48923172012373,-4.30927262332129));
#69676=CARTESIAN_POINT('Ctrl Pts',(-8.73572074447072,6.88138251617669,-1.16106420381327));
#69677=CARTESIAN_POINT('Ctrl Pts',(-8.63656686449728,6.59926097670287,2.26963653052322));
#69678=CARTESIAN_POINT('Ctrl Pts',(-8.53741298452385,4.71150858292888,5.14812415276733));
#69679=CARTESIAN_POINT('Ctrl Pts',(-8.43825910455041,1.677424262329,6.77404925162703));
#69680=CARTESIAN_POINT('Ctrl Pts',(-8.33910522457698,-1.76478517422783,
6.75181669687089));
#69681=CARTESIAN_POINT('Ctrl Pts',(-8.23995134460354,-4.77761417910377,
5.08683577235843));
#69682=CARTESIAN_POINT('Ctrl Pts',(-8.14079746463011,-6.62802745849286,
2.18420407214696));
#69683=CARTESIAN_POINT('Ctrl Pts',(-8.04164358465666,-6.86581086491974,
-1.24985462613414));
#69684=CARTESIAN_POINT('Ctrl Pts',(-7.94248970468324,-5.43311059091299,
-4.37981788733594));
#69685=CARTESIAN_POINT('Ctrl Pts',(-7.8433358247098,-2.6785092691387,-6.44415110890929));
#69686=CARTESIAN_POINT('Ctrl Pts',(-7.74418194473636,0.727785801563031,
-6.94059242762187));
#69687=CARTESIAN_POINT('Ctrl Pts',(-7.64502806476293,3.95700720561687,-5.74835536427725));
#69688=CARTESIAN_POINT('Ctrl Pts',(-7.54587418478947,6.22347037318691,-3.15751673524993));
#69689=CARTESIAN_POINT('Ctrl Pts',(-7.44672030481606,6.97573428613011,0.201560384569647));
#69690=CARTESIAN_POINT('Ctrl Pts',(-7.34756642484261,6.03076963957991,3.51159692641963));
#69691=CARTESIAN_POINT('Ctrl Pts',(-7.24841254486919,3.6184907221333,5.9672456219896));
#69692=CARTESIAN_POINT('Ctrl Pts',(-7.14925866489573,0.325816201305197,
6.97103573526099));
#69693=CARTESIAN_POINT('Ctrl Pts',(-7.05010478492232,-3.04613091496857,
6.2787404682939));
#69694=CARTESIAN_POINT('Ctrl Pts',(-6.95095090494887,-5.67694022799777,
4.05879847578804));
#69695=CARTESIAN_POINT('Ctrl Pts',(-6.85179702497544,-6.92652360977957,
0.851331957866649));
#69696=CARTESIAN_POINT('Ctrl Pts',(-6.75264314500199,-6.49085161824571,
-2.56326758049872));
#69697=CARTESIAN_POINT('Ctrl Pts',(-6.65348926502857,-4.4759252729696,-5.35421220816945));
#69698=CARTESIAN_POINT('Ctrl Pts',(-6.55433538505512,-1.37198551464726,
-6.84245213113814));
#69699=CARTESIAN_POINT('Ctrl Pts',(-6.4551815050817,2.06576469332199,-6.66589166212166));
#69700=CARTESIAN_POINT('Ctrl Pts',(-6.35602762510825,5.00090475433221,-4.86748878349157));
#69701=CARTESIAN_POINT('Ctrl Pts',(-6.25687374513482,6.71930145554519,-1.88480327059009));
#69702=CARTESIAN_POINT('Ctrl Pts',(-6.15771986516138,6.80286089627483,1.55646363441408));
#69703=CARTESIAN_POINT('Ctrl Pts',(-6.05856598518795,5.23125267639344,4.61903570618861));
#69704=CARTESIAN_POINT('Ctrl Pts',(-5.95941210521452,2.38685637713317,6.55777493165612));
#69705=CARTESIAN_POINT('Ctrl Pts',(-5.86025822524107,-1.03827316747647,
6.9009770503181));
#69706=CARTESIAN_POINT('Ctrl Pts',(-5.76110434526764,-4.21078602685766,
5.56513939226495));
#69707=CARTESIAN_POINT('Ctrl Pts',(-5.6619504652942,-6.35879508354843,2.87527746569948));
#69708=CARTESIAN_POINT('Ctrl Pts',(-5.56279658532077,-6.95967975489342,
-0.514152826157048));
#69709=CARTESIAN_POINT('Ctrl Pts',(-5.46364270534732,-5.86724200878069,
-3.77848734677226));
#69710=CARTESIAN_POINT('Ctrl Pts',(-5.3644888253739,-3.34727702405715,-6.12349834192333));
#69711=CARTESIAN_POINT('Ctrl Pts',(-5.26533494540046,-0.0129039886913769,
-6.9786337421013));
#69712=CARTESIAN_POINT('Ctrl Pts',(-5.16618106542702,3.32460864707202,-6.13583513167788));
#69713=CARTESIAN_POINT('Ctrl Pts',(-5.06702718545359,5.85322855362576,-3.8001593280202));
#69714=CARTESIAN_POINT('Ctrl Pts',(-4.96787330548015,6.95773076031128,-0.539887105177606));
#69715=CARTESIAN_POINT('Ctrl Pts',(-4.86871942550671,6.36938474897545,2.8517421585476));
#69716=CARTESIAN_POINT('Ctrl Pts',(-4.76956554553328,4.2313378374983,5.5495293065515));
#69717=CARTESIAN_POINT('Ctrl Pts',(-4.67041166555984,1.06378677232281,6.89709019241808));
#69718=CARTESIAN_POINT('Ctrl Pts',(-4.57125778558641,-2.36258855667067,
6.56655699215408));
#69719=CARTESIAN_POINT('Ctrl Pts',(-4.47210390561297,-5.21413511377609,
4.63834996896589));
#69720=CARTESIAN_POINT('Ctrl Pts',(-4.37295002563954,-6.79705837401175,
1.58161084960733));
#69721=CARTESIAN_POINT('Ctrl Pts',(-4.27379614566609,-6.72622575426015,
-1.85994153726566));
#69722=CARTESIAN_POINT('Ctrl Pts',(-4.17464226569266,-5.01887115997917,
-4.84896150725576));
#69723=CARTESIAN_POINT('Ctrl Pts',(-4.07548838571922,-2.09040189593921,
-6.65820661535616));
#69724=CARTESIAN_POINT('Ctrl Pts',(-3.97633450574579,1.34667186091541,-6.84747912142397));
#69725=CARTESIAN_POINT('Ctrl Pts',(-3.87718062577235,4.45609409767756,-5.37072814541586));
#69726=CARTESIAN_POINT('Ctrl Pts',(-3.77802674579892,6.4813279384732,-2.5872540604443));
#69727=CARTESIAN_POINT('Ctrl Pts',(-3.67887286582548,6.92962458106006,0.825710957228362));
#69728=CARTESIAN_POINT('Ctrl Pts',(-3.57971898585204,5.69191136961234,4.03777666294169));
#69729=CARTESIAN_POINT('Ctrl Pts',(-3.48056510587861,3.06932967860987,6.26743254796759));
#69730=CARTESIAN_POINT('Ctrl Pts',(-3.38141122590517,-0.300034182607279,
6.97219297700414));
#69731=CARTESIAN_POINT('Ctrl Pts',(-3.28225734593174,-3.59639833330539,
5.98058646350983));
#69732=CARTESIAN_POINT('Ctrl Pts',(-3.1831034659583,-6.01774206146008,3.53387547899653));
#69733=CARTESIAN_POINT('Ctrl Pts',(-3.08394958598486,-6.97494118899802,
0.227356172860154));
#69734=CARTESIAN_POINT('Ctrl Pts',(-2.98479570601143,-6.2351047212594,-3.13447994637828));
#69735=CARTESIAN_POINT('Ctrl Pts',(-2.88564182603799,-3.97823830795728,
-5.73368253258061));
#69736=CARTESIAN_POINT('Ctrl Pts',(-2.78648794606455,-0.753448032337097,
-6.93785352121866));
#69737=CARTESIAN_POINT('Ctrl Pts',(-2.68733406609112,2.65465964989922,-6.45401251645174));
#69738=CARTESIAN_POINT('Ctrl Pts',(-2.58818018611768,5.41687630636897,-4.39988028255512));
#69739=CARTESIAN_POINT('Ctrl Pts',(-2.48902630614424,6.86114179192153,-1.27523673506788));
#69740=CARTESIAN_POINT('Ctrl Pts',(-2.38987242617081,6.6360596041924,2.15967783452175));
#69741=CARTESIAN_POINT('Ctrl Pts',(-2.29071854619738,4.79639328513682,5.06913275359931));
#69742=CARTESIAN_POINT('Ctrl Pts',(-2.19156466622393,1.78974219685312,6.7452441236861));
#69743=CARTESIAN_POINT('Ctrl Pts',(-2.0924107862505,-1.65236148266087,6.7802062616072));
#69744=CARTESIAN_POINT('Ctrl Pts',(-1.99325690627706,-4.69243793694715,
5.1655127167802));
#69745=CARTESIAN_POINT('Ctrl Pts',(-1.89410302630363,-6.59082244117281,
2.29402593016113));
#69746=CARTESIAN_POINT('Ctrl Pts',(-1.7949491463302,-6.88562922599628,-1.13560802278984));
#69747=CARTESIAN_POINT('Ctrl Pts',(-1.69579526635675,-5.5051304310646,-4.28894326801897));
#69748=CARTESIAN_POINT('Ctrl Pts',(-1.59664138638332,-2.78520782666867,
-6.3987586906823));
#69749=CARTESIAN_POINT('Ctrl Pts',(-1.49748750640988,0.612368781399033,
-6.95172639672238));
#69750=CARTESIAN_POINT('Ctrl Pts',(-1.39833362643645,3.86095322002601,-5.81330677429719));
#69751=CARTESIAN_POINT('Ctrl Pts',(-1.29917974646301,6.17014980310849,-3.26048260638193));
#69752=CARTESIAN_POINT('Ctrl Pts',(-1.20002586648958,6.9781202739794,0.085632127128072));
#69753=CARTESIAN_POINT('Ctrl Pts',(-1.10087198651614,6.08828166342847,3.41091216628038));
#69754=CARTESIAN_POINT('Ctrl Pts',(-1.0017181065427,3.7171358393909,5.90630142905309));
#69755=CARTESIAN_POINT('Ctrl Pts',(-0.902564226569267,0.441593596660263,
6.96466011480154));
#69756=CARTESIAN_POINT('Ctrl Pts',(-0.80341034659583,-2.94139041968142,
6.32848463838897));
#69757=CARTESIAN_POINT('Ctrl Pts',(-0.704256466622392,-5.60872048188245,
4.15255944875339));
#69758=CARTESIAN_POINT('Ctrl Pts',(-0.605102586648959,-6.91142279399939,
0.966297253387595));
#69759=CARTESIAN_POINT('Ctrl Pts',(-0.505948706675522,-6.53254383143497,
-2.45506955292504));
#69760=CARTESIAN_POINT('Ctrl Pts',(-0.406794826702085,-4.5642666059668,
-5.27910653131522));
#69761=CARTESIAN_POINT('Ctrl Pts',(-0.307640946728652,-1.48548211072044,
-6.81871236510591));
#69762=CARTESIAN_POINT('Ctrl Pts',(-0.208487066755214,1.95472708327691,
-6.69929380227666));
#69763=CARTESIAN_POINT('Ctrl Pts',(-0.109333186781776,4.9193420966947,-4.94990593395533));
#69764=CARTESIAN_POINT('Ctrl Pts',(-0.0101793068083421,6.68705832384006,
-1.99618295576339));
#69765=CARTESIAN_POINT('Ctrl Pts',(0.0889745731650949,6.8277821942402,1.44322060937863));
#69766=CARTESIAN_POINT('Ctrl Pts',(0.188128453138532,5.30727493645564,4.53148189538351));
#69767=CARTESIAN_POINT('Ctrl Pts',(0.287282333111966,2.4954830302369,6.51721258400542));
#69768=CARTESIAN_POINT('Ctrl Pts',(0.386436213085403,-0.92347149068614,
6.91727517344862));
#69769=CARTESIAN_POINT('Ctrl Pts',(0.485590093058842,-4.11774110768632,
5.63433257710166));
#69770=CARTESIAN_POINT('Ctrl Pts',(0.584743973032274,-6.31014518309602,
2.98053068891579));
#69771=CARTESIAN_POINT('Ctrl Pts',(0.683897853005712,-6.96726161995643,
-0.398448162752206));
#69772=CARTESIAN_POINT('Ctrl Pts',(0.783051732979144,-5.9292109363657,-3.6804827253229));
#69773=CARTESIAN_POINT('Ctrl Pts',(0.882205612952583,-3.44855568618915,
-6.06703874213535));
#69774=CARTESIAN_POINT('Ctrl Pts',(0.981359492926021,-0.12885081635597,
-6.97745604690156));
#69775=CARTESIAN_POINT('Ctrl Pts',(1.08051337289945,3.22220405570829,-6.19022587977982));
#69776=CARTESIAN_POINT('Ctrl Pts',(1.17966725287289,5.78928171139015,-3.89688499772348));
#69777=CARTESIAN_POINT('Ctrl Pts',(1.27882113284633,6.9478002310022,-0.65541389167797));
#69778=CARTESIAN_POINT('Ctrl Pts',(1.37797501281976,6.41588667650881,2.74552245911695));
#69779=CARTESIAN_POINT('Ctrl Pts',(1.4771288927932,4.32295808686781,5.47846044053464));
#69780=CARTESIAN_POINT('Ctrl Pts',(1.57628277276664,1.17823371120998,6.87846354508673));
#69781=CARTESIAN_POINT('Ctrl Pts',(1.67543665274007,-2.25316040019159,6.6049045133391));
#69782=CARTESIAN_POINT('Ctrl Pts',(1.77459053271351,-5.13635011855482,4.72434152860911));
#69783=CARTESIAN_POINT('Ctrl Pts',(1.87374441268695,-6.76984199075704,1.69432430175027));
#69784=CARTESIAN_POINT('Ctrl Pts',(1.97289829266038,-6.75619985545904,-1.74792989917048));
#69785=CARTESIAN_POINT('Ctrl Pts',(2.07205217263382,-5.09874290755708,-4.76490463513752));
#69786=CARTESIAN_POINT('Ctrl Pts',(2.17120605260725,-2.20073812264447,-6.62255593671038));
#69787=CARTESIAN_POINT('Ctrl Pts',(2.27035993258069,1.23271647163726,-6.86890861199019));
#69788=CARTESIAN_POINT('Ctrl Pts',(2.36951381255412,4.36624542144878,-5.4440239105827));
#69789=CARTESIAN_POINT('Ctrl Pts',(2.46866769252756,6.43744657563682,-2.69458290003125));
#69790=CARTESIAN_POINT('Ctrl Pts',(2.56782157250099,6.94238707105695,0.710462648518286));
#69791=CARTESIAN_POINT('Ctrl Pts',(2.66697545247444,5.75821253933475,3.94264933403509));
#69792=CARTESIAN_POINT('Ctrl Pts',(2.76612933244787,3.17303814544387,6.21557111992748));
#69793=CARTESIAN_POINT('Ctrl Pts',(2.86528321242131,-0.184151170447852,
6.97621557620895));
#69794=CARTESIAN_POINT('Ctrl Pts',(2.96443709239474,-3.49653565104616,6.03951437288521));
#69795=CARTESIAN_POINT('Ctrl Pts',(3.06359097236818,-5.95819676363198,3.63337126442523));
#69796=CARTESIAN_POINT('Ctrl Pts',(3.16274485234161,-6.97020092320059,0.34321204751361));
#69797=CARTESIAN_POINT('Ctrl Pts',(3.26189873231505,-6.28632281617557,-3.03045225504537));
#69798=CARTESIAN_POINT('Ctrl Pts',(3.36105261228848,-4.07295316316151,-5.66679344515464));
#69799=CARTESIAN_POINT('Ctrl Pts',(3.46020649226192,-0.868615083505064,
-6.92437746342961));
#69800=CARTESIAN_POINT('Ctrl Pts',(3.55936037223536,2.54706108129972,-6.49722827575147));
#69801=CARTESIAN_POINT('Ctrl Pts',(3.6585142522088,5.34302545206699,-4.4892732639643));
#69802=CARTESIAN_POINT('Ctrl Pts',(3.75766813218223,6.83900690764945,-1.38905721085414));
#69803=CARTESIAN_POINT('Ctrl Pts',(3.85682201215567,6.67102621054105,2.04912291479273));
#69804=CARTESIAN_POINT('Ctrl Pts',(3.95597589212911,4.87995384353306,4.98874191572099));
#69805=CARTESIAN_POINT('Ctrl Pts',(4.05512977210254,1.90156603678858,6.71457683158443));
#69806=CARTESIAN_POINT('Ctrl Pts',(4.15428365207597,-1.53948162395885,6.80672401071309));
#69807=CARTESIAN_POINT('Ctrl Pts',(4.25343753204942,-4.60596624768756,5.24276361401157));
#69808=CARTESIAN_POINT('Ctrl Pts',(4.35259141202285,-6.55179789636906,2.40321447629372));
#69809=CARTESIAN_POINT('Ctrl Pts',(4.45174529199628,-6.90354665682992,-1.02104791403367));
#69810=CARTESIAN_POINT('Ctrl Pts',(4.55089917196972,-5.5756304857366,-4.19688459220349));
#69811=CARTESIAN_POINT('Ctrl Pts',(4.65005305194315,-2.89113743228502,-6.35159977285162));
#69812=CARTESIAN_POINT('Ctrl Pts',(4.74920693191659,0.496782631034447,-6.9609411789581));
#69813=CARTESIAN_POINT('Ctrl Pts',(4.84836081189003,3.76383348024845,-5.87665333808366));
#69814=CARTESIAN_POINT('Ctrl Pts',(4.94751469186346,6.1151255612177,-3.36254828190817));
#69815=CARTESIAN_POINT('Ctrl Pts',(5.0466685718369,6.97858033935209,-0.0303199103708891));
#69816=CARTESIAN_POINT('Ctrl Pts',(5.14582245181034,6.1441118612276,3.3092860236946));
#69817=CARTESIAN_POINT('Ctrl Pts',(5.24497633178377,3.81475676007768,5.8437261559544));
#69818=CARTESIAN_POINT('Ctrl Pts',(5.34413021175722,0.557245215207563,6.95636277045938));
#69819=CARTESIAN_POINT('Ctrl Pts',(5.44328409173064,-2.83583040405735,6.37647973446532));
#69820=CARTESIAN_POINT('Ctrl Pts',(5.54243797170409,-5.53896684004573,4.24517782883969));
#69821=CARTESIAN_POINT('Ctrl Pts',(5.64159185167752,-6.89438583043771,1.08098840635952));
#69822=CARTESIAN_POINT('Ctrl Pts',(5.74074573165095,-6.57248708042578,-2.34617944877944));
#69823=CARTESIAN_POINT('Ctrl Pts',(5.83989961162439,-4.65124203100119,-5.20257130344893));
#69824=CARTESIAN_POINT('Ctrl Pts',(5.93905349159782,-1.59877672992316,-6.79303474802668));
#69825=CARTESIAN_POINT('Ctrl Pts',(6.03820737157127,1.84358337102897,-6.73096805013745));
#69826=CARTESIAN_POINT('Ctrl Pts',(6.10430995822022,3.83805263429629,-5.59737979759625));
#69827=CARTESIAN_POINT('Ctrl Pts',(6.1373612515447,4.63990371690688,-4.82653440245809));
#69828=CARTESIAN_POINT('Ctrl Pts',(-13.7543612515447,3.74918558040509,-5.25724346447772));
#69829=CARTESIAN_POINT('Ctrl Pts',(-13.7213099582202,4.62259204807514,-4.634376565399));
#69830=CARTESIAN_POINT('Ctrl Pts',(-13.6552073715713,6.05211974782306,-2.94559613245471));
#69831=CARTESIAN_POINT('Ctrl Pts',(-13.5560534915978,6.72367036600214,0.306359828451381));
#69832=CARTESIAN_POINT('Ctrl Pts',(-13.4568996116244,5.7593935776168,3.48287525505259));
#69833=CARTESIAN_POINT('Ctrl Pts',(-13.357745731651,3.39379695231058,5.81243724170065));
#69834=CARTESIAN_POINT('Ctrl Pts',(-13.2585918516775,0.202490098329601,
6.72757780801801));
#69835=CARTESIAN_POINT('Ctrl Pts',(-13.1594379717041,-3.03809191952043,
6.0059851637655));
#69836=CARTESIAN_POINT('Ctrl Pts',(-13.0602840917306,-5.53948773721081,
3.8230476755157));
#69837=CARTESIAN_POINT('Ctrl Pts',(-12.9611302117572,-6.69310268371076,
0.70997628534325));
#69838=CARTESIAN_POINT('Ctrl Pts',(-12.8619763317838,-6.2182535012809,-2.57585182092111));
#69839=CARTESIAN_POINT('Ctrl Pts',(-12.7628224518103,-4.23047494773025,
-5.23495485616797));
#69840=CARTESIAN_POINT('Ctrl Pts',(-12.6636685718369,-1.21340187876777,
-6.62037336805498));
#69841=CARTESIAN_POINT('Ctrl Pts',(-12.5645146918634,2.09889734611304,-6.39502205602867));
#69842=CARTESIAN_POINT('Ctrl Pts',(-12.4653608118901,4.90052517743945,-4.61373331740821));
#69843=CARTESIAN_POINT('Ctrl Pts',(-12.3662069319166,6.50983242416413,-1.70990123493954));
#69844=CARTESIAN_POINT('Ctrl Pts',(-12.2670530519432,6.53526722067193,1.60995745550014));
#69845=CARTESIAN_POINT('Ctrl Pts',(-12.1678991719697,4.97064112977619,4.53810617563721));
#69846=CARTESIAN_POINT('Ctrl Pts',(-12.0687452919963,2.19663496534104,6.36211249860841));
#69847=CARTESIAN_POINT('Ctrl Pts',(-11.9695914120228,-1.11182269422578,
6.63818733587228));
#69848=CARTESIAN_POINT('Ctrl Pts',(-11.8704375320494,-4.14976872546465,
5.29916033305668));
#69849=CARTESIAN_POINT('Ctrl Pts',(-11.771283652076,-6.1780567477131,2.67082301374029));
#69850=CARTESIAN_POINT('Ctrl Pts',(-11.6721297721026,-6.7031948609816,-0.607337958652469));
#69851=CARTESIAN_POINT('Ctrl Pts',(-11.5729758921291,-5.59741452326445,
-3.73773078115887));
#69852=CARTESIAN_POINT('Ctrl Pts',(-11.4738220121557,-3.12975722761006,
-5.95871634150508));
#69853=CARTESIAN_POINT('Ctrl Pts',(-11.3746681321822,0.0993845416067408,
-6.72991853232244));
#69854=CARTESIAN_POINT('Ctrl Pts',(-11.2755142522088,3.30434559016186,-5.8637002789636));
#69855=CARTESIAN_POINT('Ctrl Pts',(-11.1763603722353,5.70534400537603,-3.57081650610014));
#69856=CARTESIAN_POINT('Ctrl Pts',(-11.0772064922619,6.71820571835696,-0.409136488209301));
#69857=CARTESIAN_POINT('Ctrl Pts',(-10.9780526122885,6.09649676879898,2.85208833807471));
#69858=CARTESIAN_POINT('Ctrl Pts',(-10.8788987323151,3.9914818324543,5.41938682152096));
#69859=CARTESIAN_POINT('Ctrl Pts',(-10.7797448523416,0.915320822753942,
6.66812331406536));
#69860=CARTESIAN_POINT('Ctrl Pts',(-10.6805909723682,-2.38354199549463,
6.29447442570273));
#69861=CARTESIAN_POINT('Ctrl Pts',(-10.5814370923947,-5.10247797284465,
4.3893506668714));
#69862=CARTESIAN_POINT('Ctrl Pts',(-10.4822832124213,-6.57995735444709,
1.41627749886143));
#69863=CARTESIAN_POINT('Ctrl Pts',(-10.3831293324479,-6.45650254272451,
-1.9013825643242));
#69864=CARTESIAN_POINT('Ctrl Pts',(-10.2839754524745,-4.76215066691193,
-4.75642741621855));
#69865=CARTESIAN_POINT('Ctrl Pts',(-10.184821572501,-1.90914540996877,-6.45421138046464));
#69866=CARTESIAN_POINT('Ctrl Pts',(-10.0856676925276,1.40836379467596,-6.58165573104297));
#69867=CARTESIAN_POINT('Ctrl Pts',(-9.98651381255412,4.38321154513755,-5.10775266538008));
#69868=CARTESIAN_POINT('Ctrl Pts',(-9.8873599325807,6.29160356326141,-2.39110964677092));
#69869=CARTESIAN_POINT('Ctrl Pts',(-9.78820605260725,6.6692192050819,0.907301457450251));
#69870=CARTESIAN_POINT('Ctrl Pts',(-9.68905217263382,5.42418283062754,3.98496190195714));
#69871=CARTESIAN_POINT('Ctrl Pts',(-9.58989829266038,2.85941757395946,6.09306260248953));
#69872=CARTESIAN_POINT('Ctrl Pts',(-9.49074441268695,-0.40105726265788,
6.71869286485055));
#69873=CARTESIAN_POINT('Ctrl Pts',(-9.39159053271352,-3.56395300404956,
5.70963393967168));
#69874=CARTESIAN_POINT('Ctrl Pts',(-9.29243665274007,-5.8597224222394,3.31139455130754));
#69875=CARTESIAN_POINT('Ctrl Pts',(-9.19328277276663,-6.72979415215828,
0.107477484622944));
#69876=CARTESIAN_POINT('Ctrl Pts',(-9.09412889279321,-5.96247569976116,
-3.12258935338642));
#69877=CARTESIAN_POINT('Ctrl Pts',(-8.99497501281976,-3.74445920930363,
-5.5929156948756));
#69878=CARTESIAN_POINT('Ctrl Pts',(-8.89582113284633,-0.61539839731509,
-6.7024596643849));
#69879=CARTESIAN_POINT('Ctrl Pts',(-8.79666725287289,2.66339170374145,-6.18126405944332));
#69880=CARTESIAN_POINT('Ctrl Pts',(-8.69751337289946,5.29416622976448,-4.15613819208962));
#69881=CARTESIAN_POINT('Ctrl Pts',(-8.59835949292603,6.63684551659137,-1.11980459412596));
#69882=CARTESIAN_POINT('Ctrl Pts',(-8.49920561295258,6.36474945595398,2.18898266394648));
#69883=CARTESIAN_POINT('Ctrl Pts',(-8.40005173297916,4.54408028350189,4.9651802703642));
#69884=CARTESIAN_POINT('Ctrl Pts',(-8.30089785300571,1.6178152673084,6.53332644990195));
#69885=CARTESIAN_POINT('Ctrl Pts',(-8.20174397303229,-1.7020717194237,6.51188395182705));
#69886=CARTESIAN_POINT('Ctrl Pts',(-8.10259009305884,-4.60783674938121,
4.90606983553807));
#69887=CARTESIAN_POINT('Ctrl Pts',(-8.00343621308541,-6.39249369125078,
2.10658613577598));
#69888=CARTESIAN_POINT('Ctrl Pts',(-7.90428233311196,-6.62182721996452,
-1.20543975754137));
#69889=CARTESIAN_POINT('Ctrl Pts',(-7.80512845313853,-5.2400394225549,-4.22417655764945));
#69890=CARTESIAN_POINT('Ctrl Pts',(-7.7059745731651,-2.58332568960406,-6.21515157671607));
#69891=CARTESIAN_POINT('Ctrl Pts',(-7.60682069319166,0.701923185172142,
-6.69395134298438));
#69892=CARTESIAN_POINT('Ctrl Pts',(-7.50766681321823,3.81639088802017,-5.54408164892628));
#69893=CARTESIAN_POINT('Ctrl Pts',(-7.40851293324478,6.00231295772723,-3.04531113313967));
#69894=CARTESIAN_POINT('Ctrl Pts',(-7.30935905327136,6.72784439943585,0.194397729164));
#69895=CARTESIAN_POINT('Ctrl Pts',(-7.21020517329791,5.816460042724,3.38680872083436));
#69896=CARTESIAN_POINT('Ctrl Pts',(-7.11105129332449,3.48990393566447,5.75519341638126));
#69897=CARTESIAN_POINT('Ctrl Pts',(-7.01189741335103,0.314237987756349,
6.72331281640052));
#69898=CARTESIAN_POINT('Ctrl Pts',(-6.91274353337763,-2.93788352245125,
6.05561897320447));
#69899=CARTESIAN_POINT('Ctrl Pts',(-6.81358965340416,-5.47520432290657,
3.91456490079675));
#69900=CARTESIAN_POINT('Ctrl Pts',(-6.71443577343075,-6.68038247504238,
0.8210790018453));
#69901=CARTESIAN_POINT('Ctrl Pts',(-6.61528189345729,-6.26019253545994,
-2.47217923280175));
#69902=CARTESIAN_POINT('Ctrl Pts',(-6.51612801348387,-4.31686866856674,
-5.16394477492463));
#69903=CARTESIAN_POINT('Ctrl Pts',(-6.41697413351042,-1.32323059941942,
-6.59929856279322));
#69904=CARTESIAN_POINT('Ctrl Pts',(-6.31782025353699,1.99235562199561,-6.42901235149125));
#69905=CARTESIAN_POINT('Ctrl Pts',(-6.21866637356356,4.8231924645472,-4.69451756733956));
#69906=CARTESIAN_POINT('Ctrl Pts',(-6.11951249359011,6.4805241730172,-1.81782484939125));
#69907=CARTESIAN_POINT('Ctrl Pts',(-6.02035861361669,6.56111424314798,1.50115309961553));
#69908=CARTESIAN_POINT('Ctrl Pts',(-5.92120473364324,5.04535473647355,4.45489352546932));
#69909=CARTESIAN_POINT('Ctrl Pts',(-5.82205085366982,2.30203698284238,6.32473766015244));
#69910=CARTESIAN_POINT('Ctrl Pts',(-5.72289697369637,-1.00137706345556,
6.65574373882511));
#69911=CARTESIAN_POINT('Ctrl Pts',(-5.62374309372295,-4.06115141804426,
5.36737644476719));
#69912=CARTESIAN_POINT('Ctrl Pts',(-5.5245892137495,-6.13282876543525,2.77310152608492));
#69913=CARTESIAN_POINT('Ctrl Pts',(-5.42543533377607,-6.71236038246565,
-0.495881877093973));
#69914=CARTESIAN_POINT('Ctrl Pts',(-5.32628145380263,-5.65874353433961,
-3.64421491582127));
#69915=CARTESIAN_POINT('Ctrl Pts',(-5.22712757382919,-3.2283280950709,-5.90589353533404));
#69916=CARTESIAN_POINT('Ctrl Pts',(-5.12797369385576,-0.0124454321920131,
-6.7306408202594));
#69917=CARTESIAN_POINT('Ctrl Pts',(-5.02881981388232,3.20646526215786,-5.91779192458636));
#69918=CARTESIAN_POINT('Ctrl Pts',(-4.92966593390888,5.64522806171502,-3.66511676094361));
#69919=CARTESIAN_POINT('Ctrl Pts',(-4.83051205393545,6.71048064740892,-0.520701662062845));
#69920=CARTESIAN_POINT('Ctrl Pts',(-4.73135817396201,6.1430421162185,2.75040257025954));
#69921=CARTESIAN_POINT('Ctrl Pts',(-4.63220429398858,4.08097289897303,5.3523210794918));
#69922=CARTESIAN_POINT('Ctrl Pts',(-4.53305041401514,1.02598401613378,6.65199500441502));
#69923=CARTESIAN_POINT('Ctrl Pts',(-4.43389653404171,-2.27863154431964,
6.33320764110542));
#69924=CARTESIAN_POINT('Ctrl Pts',(-4.33474265406827,-5.02884546403524,
4.47352143606987));
#69925=CARTESIAN_POINT('Ctrl Pts',(-4.23558877409483,-6.55551791947666,
1.52540668267351));
#69926=CARTESIAN_POINT('Ctrl Pts',(-4.1364348941214,-6.48720240966135,-1.7938466033105));
#69927=CARTESIAN_POINT('Ctrl Pts',(-4.03728101414796,-4.84052041550572,
-4.67664867690495));
#69928=CARTESIAN_POINT('Ctrl Pts',(-3.93812713417453,-2.01611731629858,
-6.42160040076036));
#69929=CARTESIAN_POINT('Ctrl Pts',(-3.83897325420109,1.29881649238736,-6.60414691381309));
#69930=CARTESIAN_POINT('Ctrl Pts',(-3.73981937422765,4.29774221446888,-5.17987380136782));
#69931=CARTESIAN_POINT('Ctrl Pts',(-3.64066549425422,6.25100728943547,-2.49531332853195));
#69932=CARTESIAN_POINT('Ctrl Pts',(-3.54151161428078,6.68337325012159,0.796368469794977));
#69933=CARTESIAN_POINT('Ctrl Pts',(-3.44235773430735,5.48964344961827,3.89429011967366));
#69934=CARTESIAN_POINT('Ctrl Pts',(-3.34320385433391,2.96025789418556,6.04471289144791));
#69935=CARTESIAN_POINT('Ctrl Pts',(-3.24404997436047,-0.289372159588611,
6.72442893436904));
#69936=CARTESIAN_POINT('Ctrl Pts',(-3.14489609438704,-3.46859662257756,
5.7680601773879));
#69937=CARTESIAN_POINT('Ctrl Pts',(-3.0457422144136,-5.80389541298086,3.40829558215014));
#69938=CARTESIAN_POINT('Ctrl Pts',(-2.94658833444016,-6.72707948582544,
0.219276837607698));
#69939=CARTESIAN_POINT('Ctrl Pts',(-2.84743445446673,-6.01353386728451,
-3.02309298023511));
#69940=CARTESIAN_POINT('Ctrl Pts',(-2.74828057449329,-3.83686752132008,
-5.529930231383));
#69941=CARTESIAN_POINT('Ctrl Pts',(-2.64912669451986,-0.726673482202994,
-6.69130976643494));
#69942=CARTESIAN_POINT('Ctrl Pts',(-2.54997281454642,2.56032359109411,-6.22466254900709));
#69943=CARTESIAN_POINT('Ctrl Pts',(-2.45081893457298,5.22438203999585,-4.24352601503672));
#69944=CARTESIAN_POINT('Ctrl Pts',(-2.35166505459955,6.61732406727365,-1.22991988714937));
#69945=CARTESIAN_POINT('Ctrl Pts',(-2.25251117462611,6.40024040639838,2.08293146320999));
#69946=CARTESIAN_POINT('Ctrl Pts',(-2.15335729465268,4.6259485205824,4.88899591174365));
#69947=CARTESIAN_POINT('Ctrl Pts',(-2.05420341467923,1.72614186860208,6.50554494178492));
#69948=CARTESIAN_POINT('Ctrl Pts',(-1.9550495347058,-1.59364311927237,6.53926466420501));
#69949=CARTESIAN_POINT('Ctrl Pts',(-1.85589565473237,-4.52568733252372,
4.98195091388494));
#69950=CARTESIAN_POINT('Ctrl Pts',(-1.75674177475893,-6.35661079245612,
2.21250536120366));
#69951=CARTESIAN_POINT('Ctrl Pts',(-1.65758789478549,-6.64094131521324,
-1.09525302465609));
#69952=CARTESIAN_POINT('Ctrl Pts',(-1.55843401481206,-5.30949996367323,
-4.13653126132011));
#69953=CARTESIAN_POINT('Ctrl Pts',(-1.45928013483862,-2.68623260424001,
-6.17137222471975));
#69954=CARTESIAN_POINT('Ctrl Pts',(-1.36012625486518,0.590607627431654,
-6.70468965505072));
#69955=CARTESIAN_POINT('Ctrl Pts',(-1.26097237489175,3.72375027952026,-5.60672494384176));
#69956=CARTESIAN_POINT('Ctrl Pts',(-1.16181849491831,5.95088718890311,-3.14461800622483));
#69957=CARTESIAN_POINT('Ctrl Pts',(-1.06266461494488,6.7301455987549,0.0825891014880007));
#69958=CARTESIAN_POINT('Ctrl Pts',(-0.963510734971439,5.87192831770101,
3.28970189711857));
#69959=CARTESIAN_POINT('Ctrl Pts',(-0.864356854998003,3.58504359730451,
5.696414937972));
#69960=CARTESIAN_POINT('Ctrl Pts',(-0.765202975024567,0.425901114385129,
6.71716376016619));
#69961=CARTESIAN_POINT('Ctrl Pts',(-0.666049095051132,-2.83686508830405,
6.10359543309403));
#69962=CARTESIAN_POINT('Ctrl Pts',(-0.566895215077694,-5.40940883557766,
4.0049939812313));
#69963=CARTESIAN_POINT('Ctrl Pts',(-0.46774133510426,-6.66581828226979,
0.93195888744215));
#69964=CARTESIAN_POINT('Ctrl Pts',(-0.368587455130823,-6.30040317300718,
-2.36782613333107));
#69965=CARTESIAN_POINT('Ctrl Pts',(-0.269433575157386,-4.4020707015091,
-5.09150805548215));
#69966=CARTESIAN_POINT('Ctrl Pts',(-0.170279695183953,-1.43269397731273,
-6.57640241374388));
#69967=CARTESIAN_POINT('Ctrl Pts',(-0.0711258152105153,1.88526384753484,
-6.46122751226907));
#69968=CARTESIAN_POINT('Ctrl Pts',(0.0280280647629222,4.74452821976931,
-4.77400593966295));
#69969=CARTESIAN_POINT('Ctrl Pts',(0.127181944736356,6.44942683413289,-1.92524654298902));
#69970=CARTESIAN_POINT('Ctrl Pts',(0.226335824709794,6.58514993717897,1.39193428185253));
#69971=CARTESIAN_POINT('Ctrl Pts',(0.32548970468323,5.11867546739773,4.37045102930867));
#69972=CARTESIAN_POINT('Ctrl Pts',(0.424643584656665,2.4068034761944,6.28561673721068));
#69973=CARTESIAN_POINT('Ctrl Pts',(0.523797464630102,-0.890654982229587,
6.6714626914009));
#69974=CARTESIAN_POINT('Ctrl Pts',(0.622951344603541,-3.97141294569627,
5.43411077867214));
#69975=CARTESIAN_POINT('Ctrl Pts',(0.722105224576973,-6.08590768919204,
2.8746144678474));
#69976=CARTESIAN_POINT('Ctrl Pts',(0.82125910455041,-6.7196728181619,-0.384288897810818));
#69977=CARTESIAN_POINT('Ctrl Pts',(0.920412984523844,-5.71851033239854,
-3.5496929893127));
#69978=CARTESIAN_POINT('Ctrl Pts',(1.01956686449728,-3.32600771586179,-5.85144028544703));
#69979=CARTESIAN_POINT('Ctrl Pts',(1.11872074447072,-0.124271970179066,
-6.7295049756689));
#69980=CARTESIAN_POINT('Ctrl Pts',(1.21787462444415,3.10769972318758,-5.97024984155809));
#69981=CARTESIAN_POINT('Ctrl Pts',(1.31702850441759,5.58355363623528,-3.75840518457078));
#69982=CARTESIAN_POINT('Ctrl Pts',(1.41618238439102,6.70090300966427,-0.632123085480108));
#69983=CARTESIAN_POINT('Ctrl Pts',(1.51533626436446,6.18789154996778,2.64795749700821));
#69984=CARTESIAN_POINT('Ctrl Pts',(1.6144901443379,4.16933732862471,5.28377771866504));
#69985=CARTESIAN_POINT('Ctrl Pts',(1.71364402431134,1.13636396543253,6.63403027413886));
#69986=CARTESIAN_POINT('Ctrl Pts',(1.81279790428477,-2.1730920298384,6.37019244371608));
#69987=CARTESIAN_POINT('Ctrl Pts',(1.91195178425821,-4.9538246385574,4.55645719726919));
#69988=CARTESIAN_POINT('Ctrl Pts',(2.01110566423164,-6.52926869837069,1.63411474646096));
#69989=CARTESIAN_POINT('Ctrl Pts',(2.11025954420508,-6.51611135037028,-1.68581541388737));
#69990=CARTESIAN_POINT('Ctrl Pts',(2.20941342417852,-4.91755383845069,-4.59557885212116));
#69991=CARTESIAN_POINT('Ctrl Pts',(2.30856730415195,-2.12253263179732,-6.38721660561782));
#69992=CARTESIAN_POINT('Ctrl Pts',(2.40772118412539,1.18891062497711,-6.62481488540933));
#69993=CARTESIAN_POINT('Ctrl Pts',(2.50687506409882,4.21108640328576,-5.25056492619473));
#69994=CARTESIAN_POINT('Ctrl Pts',(2.60602894407226,6.20868529592357,-2.59882812750426));
#69995=CARTESIAN_POINT('Ctrl Pts',(2.70518282404569,6.69568221192067,0.685215628173524));
#69996=CARTESIAN_POINT('Ctrl Pts',(2.80433670401913,5.55358853913808,3.8025432381604));
#69997=CARTESIAN_POINT('Ctrl Pts',(2.90349058399257,3.0602809740713,5.99469441255026));
#69998=CARTESIAN_POINT('Ctrl Pts',(3.002644463966,-0.177607169357161,6.72830858637717));
#69999=CARTESIAN_POINT('Ctrl Pts',(3.10179834393944,-3.37228266335948,5.82489402294447));
#70000=CARTESIAN_POINT('Ctrl Pts',(3.20095222391288,-5.74646611850472,3.5042556825936));
#70001=CARTESIAN_POINT('Ctrl Pts',(3.30010610388631,-6.7225076702446,0.331015654692348));
#70002=CARTESIAN_POINT('Ctrl Pts',(3.39925998385975,-6.06293187456192,-2.9227620198211));
#70003=CARTESIAN_POINT('Ctrl Pts',(3.49841386383318,-3.92821658680787,-5.46541811641943));
#70004=CARTESIAN_POINT('Ctrl Pts',(3.59756774380662,-0.837747953852602,
-6.67831259420852));
#70005=CARTESIAN_POINT('Ctrl Pts',(3.69672162378006,2.45654864820692,-6.26634259188805));
#70006=CARTESIAN_POINT('Ctrl Pts',(3.79587550375349,5.15315555169669,-4.32974232498397));
#70007=CARTESIAN_POINT('Ctrl Pts',(3.89502938372693,6.5959757688618,-1.33969563535732));
#70008=CARTESIAN_POINT('Ctrl Pts',(3.99418326370036,6.43396443845587,1.97630522616884));
#70009=CARTESIAN_POINT('Ctrl Pts',(4.09333714367381,4.70653966866234,4.81146184490557));
#70010=CARTESIAN_POINT('Ctrl Pts',(4.19249102364724,1.83399193346608,6.47596744342429));
#70011=CARTESIAN_POINT('Ctrl Pts',(4.29164490362067,-1.48477456235392,6.56484007784463));
#70012=CARTESIAN_POINT('Ctrl Pts',(4.39079878359412,-4.44228850360737,5.05645662109383));
#70013=CARTESIAN_POINT('Ctrl Pts',(4.48995266356754,-6.31897302495677,2.31781378013833));
#70014=CARTESIAN_POINT('Ctrl Pts',(4.58910654354099,-6.6582220317288,-0.984763927095942));
#70015=CARTESIAN_POINT('Ctrl Pts',(4.68826042351442,-5.37749472645081,-4.04774398515678));
#70016=CARTESIAN_POINT('Ctrl Pts',(4.78741430348785,-2.78839789245884,-6.12588914749855));
#70017=CARTESIAN_POINT('Ctrl Pts',(4.88656818346129,0.47912894970609,-6.71357698052983));
#70018=CARTESIAN_POINT('Ctrl Pts',(4.98572206343473,3.63008178950389,-5.66782042238396));
#70019=CARTESIAN_POINT('Ctrl Pts',(5.08487594340816,5.89781828999535,-3.24305667308019));
#70020=CARTESIAN_POINT('Ctrl Pts',(5.18402982338161,6.73058931523177,-0.0292424611966137));
#70021=CARTESIAN_POINT('Ctrl Pts',(5.28318370335503,5.92577453204566,3.19168714394893));
#70022=CARTESIAN_POINT('Ctrl Pts',(5.38233758332848,3.67919545825143,5.63606334151036));
#70023=CARTESIAN_POINT('Ctrl Pts',(5.4814914633019,0.537442933814262,6.70916127048226));
#70024=CARTESIAN_POINT('Ctrl Pts',(5.58064534327535,-2.73505625631732,6.1498849741076));
#70025=CARTESIAN_POINT('Ctrl Pts',(5.67979922324878,-5.34213396108817,4.09432107199899));
#70026=CARTESIAN_POINT('Ctrl Pts',(5.77895310322222,-6.64938674471686,1.04257437242718));
#70027=CARTESIAN_POINT('Ctrl Pts',(5.87810698319565,-6.33892699759613,-2.26280555094068));
#70028=CARTESIAN_POINT('Ctrl Pts',(5.97726086316909,-4.48595536543181,-5.01769258559197));
#70029=CARTESIAN_POINT('Ctrl Pts',(6.07641474314252,-1.54196255579125,-6.55163727717598));
#70030=CARTESIAN_POINT('Ctrl Pts',(6.17556862311597,1.77806974132202,-6.49177618318107));
#70031=CARTESIAN_POINT('Ctrl Pts',(6.24167120976492,3.70166348963895,-5.39847115416216));
#70032=CARTESIAN_POINT('Ctrl Pts',(6.2747225030894,4.47501996998105,-4.65501854232418));
#70033=CARTESIAN_POINT('Ctrl Pts',(-13.617,3.61104546693871,-5.06353840690493));
#70034=CARTESIAN_POINT('Ctrl Pts',(-13.5839487066755,4.45227095397745,-4.46362126645189));
#70035=CARTESIAN_POINT('Ctrl Pts',(-13.5178461200266,5.82912718297219,-2.83706456600194));
#70036=CARTESIAN_POINT('Ctrl Pts',(-13.4186922400531,6.47593427309586,0.295071888562534));
#70037=CARTESIAN_POINT('Ctrl Pts',(-13.3195383600797,5.54718661553207,3.35454744289073));
#70038=CARTESIAN_POINT('Ctrl Pts',(-13.2203844801062,3.26875126278153,5.59827586641925));
#70039=CARTESIAN_POINT('Ctrl Pts',(-13.1212306001328,0.195029276623322,
6.47969774398204));
#70040=CARTESIAN_POINT('Ctrl Pts',(-13.0220767201594,-2.92615231197546,
5.78469244453168));
#70041=CARTESIAN_POINT('Ctrl Pts',(-12.9229228401859,-5.33538328621662,
3.6821860861499));
#70042=CARTESIAN_POINT('Ctrl Pts',(-12.8237689602125,-6.44649286823449,
0.683816949532182));
#70043=CARTESIAN_POINT('Ctrl Pts',(-12.7246150802391,-5.98913967754298,
-2.48094361881069));
#70044=CARTESIAN_POINT('Ctrl Pts',(-12.6254612002656,-4.07460155155841,
-5.04207103051742));
#70045=CARTESIAN_POINT('Ctrl Pts',(-12.5263073202922,-1.16869364290732,
-6.37644329080494));
#70046=CARTESIAN_POINT('Ctrl Pts',(-12.4271534403188,2.02156270600836,-6.15939513026191));
#70047=CARTESIAN_POINT('Ctrl Pts',(-12.3279995603453,4.71996353557397,-4.4437386264808));
#70048=CARTESIAN_POINT('Ctrl Pts',(-12.2288456803719,6.26997526840712,-1.6468992987736));
#70049=CARTESIAN_POINT('Ctrl Pts',(-12.1296918003985,6.29447291053824,1.55063798442858));
#70050=CARTESIAN_POINT('Ctrl Pts',(-12.030537920425,4.78749604001144,4.37089799439875));
#70051=CARTESIAN_POINT('Ctrl Pts',(-11.9313840404516,2.11569914692158,6.12769813751704));
#70052=CARTESIAN_POINT('Ctrl Pts',(-11.8322301604782,-1.07085718055863,
6.39360089646495));
#70053=CARTESIAN_POINT('Ctrl Pts',(-11.7330762805047,-3.99686897955958,
5.10391083313569));
#70054=CARTESIAN_POINT('Ctrl Pts',(-11.6339224005313,-5.9504239880569,2.57241556330756));
#70055=CARTESIAN_POINT('Ctrl Pts',(-11.5347685205579,-6.45621319554393,
-0.584960369514416));
#70056=CARTESIAN_POINT('Ctrl Pts',(-11.4356146405844,-5.39117573865922,
-3.60001272395876));
#70057=CARTESIAN_POINT('Ctrl Pts',(-11.336460760611,-3.01444017827433,-5.73916525930964));
#70058=CARTESIAN_POINT('Ctrl Pts',(-11.2373068806375,0.0957226818348403,
-6.48195222344366));
#70059=CARTESIAN_POINT('Ctrl Pts',(-11.1381530006641,3.18259576877592,-5.64765009833173));
#70060=CARTESIAN_POINT('Ctrl Pts',(-11.0389991206906,5.49512851954185,-3.43924846639081));
#70061=CARTESIAN_POINT('Ctrl Pts',(-10.9398452407172,6.47067097239111,-0.394061704715005));
#70062=CARTESIAN_POINT('Ctrl Pts',(-10.8406913607438,5.87186911638537,2.7470021004937));
#70063=CARTESIAN_POINT('Ctrl Pts',(-10.7415374807704,3.84441422499412,5.219707532676));
#70064=CARTESIAN_POINT('Ctrl Pts',(-10.6423836007969,0.881595492385054,
6.42243387259649));
#70065=CARTESIAN_POINT('Ctrl Pts',(-10.5432297208235,-2.29571951921329,
6.062552214137));
#70066=CARTESIAN_POINT('Ctrl Pts',(-10.44407584085,-4.9144753063956,4.22762343674055));
#70067=CARTESIAN_POINT('Ctrl Pts',(-10.3449219608766,-6.33751641999512,
1.36409423660437));
#70068=CARTESIAN_POINT('Ctrl Pts',(-10.2457680809032,-6.21861034594731,
-1.83132542856878));
#70069=CARTESIAN_POINT('Ctrl Pts',(-10.1466142009297,-4.58668748447852,
-4.58117510904947));
#70070=CARTESIAN_POINT('Ctrl Pts',(-10.0474603209563,-1.83880224932734,
-6.21640360239859));
#70071=CARTESIAN_POINT('Ctrl Pts',(-9.94830644098286,1.35647211574301,-6.33915221928435));
#70072=CARTESIAN_POINT('Ctrl Pts',(-9.84915256100943,4.22171051319157,-4.91955565095604));
#70073=CARTESIAN_POINT('Ctrl Pts',(-9.749998681036,6.05978712967198,-2.30300833761142));
#70074=CARTESIAN_POINT('Ctrl Pts',(-9.65084480106255,6.42348938510785,0.873871603528));
#70075=CARTESIAN_POINT('Ctrl Pts',(-9.55169092108912,5.22432683107353,3.83813452371996));
#70076=CARTESIAN_POINT('Ctrl Pts',(-9.45253704111568,2.75406128800256,5.86856148318917));
#70077=CARTESIAN_POINT('Ctrl Pts',(-9.35338316114225,-0.386280161182942,
6.47114016979406));
#70078=CARTESIAN_POINT('Ctrl Pts',(-9.25422928116881,-3.43263785258272,
5.49926038963988));
#70079=CARTESIAN_POINT('Ctrl Pts',(-9.15507540119538,-5.6438188071929,3.18938500837096));
#70080=CARTESIAN_POINT('Ctrl Pts',(-9.05592152122194,-6.48183242611213,
0.103517437406672));
#70081=CARTESIAN_POINT('Ctrl Pts',(-8.95676764124851,-5.74278610263628,
-3.00753640699718));
#70082=CARTESIAN_POINT('Ctrl Pts',(-8.85761376127506,-3.60649324070849,
-5.38684267124721));
#70083=CARTESIAN_POINT('Ctrl Pts',(-8.75845988130164,-0.592723818367459,
-6.45550508753466));
#70084=CARTESIAN_POINT('Ctrl Pts',(-8.65930600132819,2.56525806264267,-5.95351312521376));
#70085=CARTESIAN_POINT('Ctrl Pts',(-8.56015212135476,5.09910073940523,-4.00300376085795));
#70086=CARTESIAN_POINT('Ctrl Pts',(-8.46099824138133,6.39230851700605,-1.07854498443864));
#70087=CARTESIAN_POINT('Ctrl Pts',(-8.36184436140788,6.13023793520507,2.10832879736973));
#70088=CARTESIAN_POINT('Ctrl Pts',(-8.26269048143445,4.37665198407491,4.78223638796107));
#70089=CARTESIAN_POINT('Ctrl Pts',(-8.16353660146101,1.55820627228779,6.29260364817686));
#70090=CARTESIAN_POINT('Ctrl Pts',(-8.06438272148758,-1.63935826461956,
6.27195120678321));
#70091=CARTESIAN_POINT('Ctrl Pts',(-7.96522884151414,-4.43805931965865,
4.72530389871772));
#70092=CARTESIAN_POINT('Ctrl Pts',(-7.86607496154071,-6.15695992400869,
2.028968199405));
#70093=CARTESIAN_POINT('Ctrl Pts',(-7.76692108156727,-6.37784357500933,
-1.16102488894861));
#70094=CARTESIAN_POINT('Ctrl Pts',(-7.66776720159383,-5.0469682541968,-4.06853522796294));
#70095=CARTESIAN_POINT('Ctrl Pts',(-7.5686133216204,-2.48814211006943,-5.98615204452285));
#70096=CARTESIAN_POINT('Ctrl Pts',(-7.46945944164697,0.676060568781244,
-6.44731025834689));
#70097=CARTESIAN_POINT('Ctrl Pts',(-7.37030556167352,3.6757745704235,-5.3398079335753));
#70098=CARTESIAN_POINT('Ctrl Pts',(-7.2711516817001,5.78115554226751,-2.93310553102942));
#70099=CARTESIAN_POINT('Ctrl Pts',(-7.17199780172665,6.47995451274163,0.187235073758361));
#70100=CARTESIAN_POINT('Ctrl Pts',(-7.07284392175322,5.60215044586807,3.26202051524908));
#70101=CARTESIAN_POINT('Ctrl Pts',(-6.97369004177978,3.36131714919565,5.54314121077292));
#70102=CARTESIAN_POINT('Ctrl Pts',(-6.87453616180634,0.302659774207504,
6.47558989754003));
#70103=CARTESIAN_POINT('Ctrl Pts',(-6.77538228183291,-2.82963612993394,
5.83249747811505));
#70104=CARTESIAN_POINT('Ctrl Pts',(-6.67622840185946,-5.27346841781536,
3.77033132580544));
#70105=CARTESIAN_POINT('Ctrl Pts',(-6.57707452188605,-6.4342413403052,0.79082604582396));
#70106=CARTESIAN_POINT('Ctrl Pts',(-6.47792064191259,-6.02953345267415,
-2.38109088510478));
#70107=CARTESIAN_POINT('Ctrl Pts',(-6.37876676193917,-4.1578120641639,-4.97367734167979));
#70108=CARTESIAN_POINT('Ctrl Pts',(-6.27961288196573,-1.27447568419159,
-6.3561449944483));
#70109=CARTESIAN_POINT('Ctrl Pts',(-6.18045900199229,1.91894655066922,-6.19213304086084));
#70110=CARTESIAN_POINT('Ctrl Pts',(-6.08130512201886,4.64548017476219,-4.52154635118754));
#70111=CARTESIAN_POINT('Ctrl Pts',(-5.98215124204542,6.24174689048921,-1.75084642819241));
#70112=CARTESIAN_POINT('Ctrl Pts',(-5.88299736207198,6.31936759002112,1.44584256481697));
#70113=CARTESIAN_POINT('Ctrl Pts',(-5.78384348209855,4.85945679655365,4.29075134475004));
#70114=CARTESIAN_POINT('Ctrl Pts',(-5.68468960212512,2.21721758855159,6.09170038864876));
#70115=CARTESIAN_POINT('Ctrl Pts',(-5.58553572215167,-0.964480959434654,
6.41051042733211));
#70116=CARTESIAN_POINT('Ctrl Pts',(-5.48638184217824,-3.91151680923086,
5.16961349726944));
#70117=CARTESIAN_POINT('Ctrl Pts',(-5.38722796220481,-5.90686244732208,
2.67092558647035));
#70118=CARTESIAN_POINT('Ctrl Pts',(-5.28807408223136,-6.46504101003786,
-0.477610928030889));
#70119=CARTESIAN_POINT('Ctrl Pts',(-5.18892020225794,-5.45024505989854,
-3.50994248487028));
#70120=CARTESIAN_POINT('Ctrl Pts',(-5.08976632228449,-3.10937916608465,
-5.68828872874475));
#70121=CARTESIAN_POINT('Ctrl Pts',(-4.99061244231106,-0.0119868756926444,
-6.48264789841751));
#70122=CARTESIAN_POINT('Ctrl Pts',(-4.89145856233762,3.08832187724368,-5.69974871749482));
#70123=CARTESIAN_POINT('Ctrl Pts',(-4.79230468236419,5.43722756980429,-3.53007419386704));
#70124=CARTESIAN_POINT('Ctrl Pts',(-4.69315080239075,6.46323053450655,-0.501516218948075));
#70125=CARTESIAN_POINT('Ctrl Pts',(-4.59399692241732,5.91669948346157,2.64906298197146));
#70126=CARTESIAN_POINT('Ctrl Pts',(-4.49484304244388,3.93060796044775,5.15511285243209));
#70127=CARTESIAN_POINT('Ctrl Pts',(-4.39568916247044,0.988181259944745,
6.40689981641197));
#70128=CARTESIAN_POINT('Ctrl Pts',(-4.29653528249701,-2.19467453196863,
6.09985829005677));
#70129=CARTESIAN_POINT('Ctrl Pts',(-4.19738140252357,-4.84355581429439,
4.30869290317386));
#70130=CARTESIAN_POINT('Ctrl Pts',(-4.09822752255014,-6.31397746494157,
1.46920251573968));
#70131=CARTESIAN_POINT('Ctrl Pts',(-3.9990736425767,-6.24817906506253,-1.72775166935533));
#70132=CARTESIAN_POINT('Ctrl Pts',(-3.89991976260326,-4.66216967103227,
-4.50433584655415));
#70133=CARTESIAN_POINT('Ctrl Pts',(-3.80076588262983,-1.94183273665795,
-6.18499418616455));
#70134=CARTESIAN_POINT('Ctrl Pts',(-3.70161200265638,1.25096112385931,-6.36081470620222));
#70135=CARTESIAN_POINT('Ctrl Pts',(-3.60245812268296,4.13939033126021,-4.98901945731978));
#70136=CARTESIAN_POINT('Ctrl Pts',(-3.50330424270952,6.02068664039774,-2.40337259661961));
#70137=CARTESIAN_POINT('Ctrl Pts',(-3.40415036273608,6.43712191918314,0.767025982361597));
#70138=CARTESIAN_POINT('Ctrl Pts',(-3.30499648276265,5.28737552962418,3.75080357640562));
#70139=CARTESIAN_POINT('Ctrl Pts',(-3.20584260278921,2.85118610976127,5.82199323492824));
#70140=CARTESIAN_POINT('Ctrl Pts',(-3.10668872281577,-0.278710136569954,
6.47666489173394));
#70141=CARTESIAN_POINT('Ctrl Pts',(-3.00753484284234,-3.34079491184971,
5.55553389126599));
#70142=CARTESIAN_POINT('Ctrl Pts',(-2.9083809628689,-5.59004876450166,3.28271568530374));
#70143=CARTESIAN_POINT('Ctrl Pts',(-2.80922708289547,-6.47921778265285,
0.211197502355245));
#70144=CARTESIAN_POINT('Ctrl Pts',(-2.71007320292203,-5.79196301330962,
-2.91170601409193));
#70145=CARTESIAN_POINT('Ctrl Pts',(-2.61091932294859,-3.69549673468289,
-5.3261779301854));
#70146=CARTESIAN_POINT('Ctrl Pts',(-2.51176544297515,-0.699898932068888,
-6.4447660116512));
#70147=CARTESIAN_POINT('Ctrl Pts',(-2.41261156300172,2.46598753228901,-5.99531258156246));
#70148=CARTESIAN_POINT('Ctrl Pts',(-2.31345768302828,5.03188777362273,-4.0871717475183));
#70149=CARTESIAN_POINT('Ctrl Pts',(-2.21430380305485,6.37350634262576,-1.18460303923088));
#70150=CARTESIAN_POINT('Ctrl Pts',(-2.11514992308141,6.16442120860435,2.00618509189823));
#70151=CARTESIAN_POINT('Ctrl Pts',(-2.01599604310798,4.45550375602798,4.708859069888));
#70152=CARTESIAN_POINT('Ctrl Pts',(-1.91684216313454,1.66254154035103,6.26584575988373));
#70153=CARTESIAN_POINT('Ctrl Pts',(-1.8176882831611,-1.53492475588388,6.29832306680283));
#70154=CARTESIAN_POINT('Ctrl Pts',(-1.71853440318767,-4.35893672810028,
4.79838911098967));
#70155=CARTESIAN_POINT('Ctrl Pts',(-1.61938052321423,-6.12239914373944,
2.1309847922462));
#70156=CARTESIAN_POINT('Ctrl Pts',(-1.5202266432408,-6.3962534044302,-1.05489802652235));
#70157=CARTESIAN_POINT('Ctrl Pts',(-1.42107276326736,-5.11386949628186,
-3.98411925462125));
#70158=CARTESIAN_POINT('Ctrl Pts',(-1.32191888329392,-2.58725738181136,
-5.9439857587572));
#70159=CARTESIAN_POINT('Ctrl Pts',(-1.22276500332049,0.568846473464286,
-6.45765291337906));
#70160=CARTESIAN_POINT('Ctrl Pts',(-1.12361112334705,3.58654733901449,-5.40014311338634));
#70161=CARTESIAN_POINT('Ctrl Pts',(-1.02445724337361,5.73162457469774,-3.02875340606772));
#70162=CARTESIAN_POINT('Ctrl Pts',(-0.925303363400179,6.4821709235304,0.0795460758479203));
#70163=CARTESIAN_POINT('Ctrl Pts',(-0.826149483426742,5.65557497197356,
3.16849162795677));
#70164=CARTESIAN_POINT('Ctrl Pts',(-0.726995603453303,3.45295135521813,
5.4865284468909));
#70165=CARTESIAN_POINT('Ctrl Pts',(-0.627841723479869,0.410208632109992,
6.46966740553085));
#70166=CARTESIAN_POINT('Ctrl Pts',(-0.528687843506432,-2.73233975692668,
5.87870622779908));
#70167=CARTESIAN_POINT('Ctrl Pts',(-0.429533963532995,-5.21009718927287,
3.85742851370921));
#70168=CARTESIAN_POINT('Ctrl Pts',(-0.330380083559561,-6.42021377054019,
0.897620521496703));
#70169=CARTESIAN_POINT('Ctrl Pts',(-0.231226203586124,-6.06826251457938,
-2.28058271373709));
#70170=CARTESIAN_POINT('Ctrl Pts',(-0.132072323612687,-4.2398747970514,
-4.9039095796491));
#70171=CARTESIAN_POINT('Ctrl Pts',(-0.0329184436392546,-1.37990584390503,
-6.33409246238185));
#70172=CARTESIAN_POINT('Ctrl Pts',(0.0662354363341833,1.81580061179276,
-6.22316122226147));
#70173=CARTESIAN_POINT('Ctrl Pts',(0.165389316307621,4.56971434284393,-4.59810594537058));
#70174=CARTESIAN_POINT('Ctrl Pts',(0.264543196281055,6.21179534442574,-1.85431013021464));
#70175=CARTESIAN_POINT('Ctrl Pts',(0.363697076254493,6.34251768011774,1.34064795432643));
#70176=CARTESIAN_POINT('Ctrl Pts',(0.462850956227929,4.93007599833982,4.20942016323384));
#70177=CARTESIAN_POINT('Ctrl Pts',(0.562004836201364,2.31812392215191,6.05402089041596));
#70178=CARTESIAN_POINT('Ctrl Pts',(0.6611587161748,-0.857838473773044,6.42565020935318));
#70179=CARTESIAN_POINT('Ctrl Pts',(0.76031259614824,-3.82508478370621,5.23388898024262));
#70180=CARTESIAN_POINT('Ctrl Pts',(0.859466476121671,-5.86167019528809,
2.768698246779));
#70181=CARTESIAN_POINT('Ctrl Pts',(0.95862035609511,-6.47208401636734,-0.37012963286943));
#70182=CARTESIAN_POINT('Ctrl Pts',(1.05777423606854,-5.50780972843139,-3.4189032533025));
#70183=CARTESIAN_POINT('Ctrl Pts',(1.15692811604198,-3.20345974553442,-5.63584182875872));
#70184=CARTESIAN_POINT('Ctrl Pts',(1.25608199601542,-0.119693124002174,
-6.48155390443623));
#70185=CARTESIAN_POINT('Ctrl Pts',(1.35523587598885,2.99319539066687,-5.75027380333636));
#70186=CARTESIAN_POINT('Ctrl Pts',(1.45438975596229,5.3778255610804,-3.61992537141806));
#70187=CARTESIAN_POINT('Ctrl Pts',(1.55354363593573,6.45400578832633,-0.608832279282255));
#70188=CARTESIAN_POINT('Ctrl Pts',(1.65269751590916,5.95989642342674,2.55039253489949));
#70189=CARTESIAN_POINT('Ctrl Pts',(1.7518513958826,4.01571657038161,5.08909499679543));
#70190=CARTESIAN_POINT('Ctrl Pts',(1.85100527585604,1.09449421965509,6.38959700319101));
#70191=CARTESIAN_POINT('Ctrl Pts',(1.95015915582947,-2.09302365948521,6.13548037409304));
#70192=CARTESIAN_POINT('Ctrl Pts',(2.04931303580291,-4.77129915855997,4.38857286592929));
#70193=CARTESIAN_POINT('Ctrl Pts',(2.14846691577634,-6.28869540598436,1.57390519117164));
#70194=CARTESIAN_POINT('Ctrl Pts',(2.24762079574978,-6.27602284528152,-1.62370092860426));
#70195=CARTESIAN_POINT('Ctrl Pts',(2.34677467572321,-4.7363647693443,-4.42625306910482));
#70196=CARTESIAN_POINT('Ctrl Pts',(2.44592855569665,-2.04432714095016,-6.15187727452525));
#70197=CARTESIAN_POINT('Ctrl Pts',(2.54508243567009,1.14510477831697,-6.38072115882848));
#70198=CARTESIAN_POINT('Ctrl Pts',(2.64423631564352,4.05592738512275,-5.05710594180675));
#70199=CARTESIAN_POINT('Ctrl Pts',(2.74339019561696,5.97992401621031,-2.50307335497727));
#70200=CARTESIAN_POINT('Ctrl Pts',(2.84254407559039,6.44897735278439,0.659968607828769));
#70201=CARTESIAN_POINT('Ctrl Pts',(2.94169795556383,5.3489645389414,3.6624371422857));
#70202=CARTESIAN_POINT('Ctrl Pts',(3.04085183553727,2.94752380269873,5.77381770517306));
#70203=CARTESIAN_POINT('Ctrl Pts',(3.1400057155107,-0.171063168266469,6.48040159654536));
#70204=CARTESIAN_POINT('Ctrl Pts',(3.23915959548414,-3.2480296756728,5.61027367300375));
#70205=CARTESIAN_POINT('Ctrl Pts',(3.33831347545758,-5.53473547337747,3.37514010076197));
#70206=CARTESIAN_POINT('Ctrl Pts',(3.43746735543101,-6.47481441728861,0.318819261871086));
#70207=CARTESIAN_POINT('Ctrl Pts',(3.53662123540445,-5.83954093294827,-2.81507178459683));
#70208=CARTESIAN_POINT('Ctrl Pts',(3.63577511537788,-3.78348001045424,-5.26404278768421));
#70209=CARTESIAN_POINT('Ctrl Pts',(3.73492899535132,-0.806880824200139,
-6.43224772498744));
#70210=CARTESIAN_POINT('Ctrl Pts',(3.83408287532476,2.36603621511411,-6.03545690802462));
#70211=CARTESIAN_POINT('Ctrl Pts',(3.93323675529819,4.96328565132639,-4.17021138600364));
#70212=CARTESIAN_POINT('Ctrl Pts',(4.03239063527163,6.35294463007415,-1.29033405986049));
#70213=CARTESIAN_POINT('Ctrl Pts',(4.13154451524507,6.1969026663707,1.90348753754495));
#70214=CARTESIAN_POINT('Ctrl Pts',(4.2306983952185,4.53312549379163,4.63418177409014));
#70215=CARTESIAN_POINT('Ctrl Pts',(4.32985227519194,1.76641783014358,6.23735805526417));
#70216=CARTESIAN_POINT('Ctrl Pts',(4.42900615516537,-1.430067500749,6.32295614497614));
#70217=CARTESIAN_POINT('Ctrl Pts',(4.52816003513881,-4.27861075952717,4.87014962817609));
#70218=CARTESIAN_POINT('Ctrl Pts',(4.62731391511224,-6.08614815354451,2.23241308398294));
#70219=CARTESIAN_POINT('Ctrl Pts',(4.72646779508569,-6.41289740662767,-0.948479940158207));
#70220=CARTESIAN_POINT('Ctrl Pts',(4.82562167505912,-5.17935896716503,-3.89860337811007));
#70221=CARTESIAN_POINT('Ctrl Pts',(4.92477555503255,-2.68565835263266,-5.90017852214549));
#70222=CARTESIAN_POINT('Ctrl Pts',(5.02392943500599,0.461475268377732,-6.46621278210156));
#70223=CARTESIAN_POINT('Ctrl Pts',(5.12308331497942,3.49633009875934,-5.45898750668426));
#70224=CARTESIAN_POINT('Ctrl Pts',(5.22223719495286,5.68051101877298,-3.1235650642522));
#70225=CARTESIAN_POINT('Ctrl Pts',(5.3213910749263,6.48259829111145,-0.0281650120223385));
#70226=CARTESIAN_POINT('Ctrl Pts',(5.42054495489973,5.70743720286374,3.07408826420326));
#70227=CARTESIAN_POINT('Ctrl Pts',(5.51969883487318,3.54363415642518,5.42840052706632));
#70228=CARTESIAN_POINT('Ctrl Pts',(5.6188527148466,0.51764065242096,6.46195977050514));
#70229=CARTESIAN_POINT('Ctrl Pts',(5.71800659482005,-2.63428210857727,5.92329021374989));
#70230=CARTESIAN_POINT('Ctrl Pts',(5.81716047479348,-5.14530108213061,3.94346431515829));
#70231=CARTESIAN_POINT('Ctrl Pts',(5.91631435476693,-6.40438765899599,1.00416033849484));
#70232=CARTESIAN_POINT('Ctrl Pts',(6.01546823474035,-6.1053669147665,-2.17943165310192));
#70233=CARTESIAN_POINT('Ctrl Pts',(6.11462211471379,-4.32066869986243,-4.83281386773501));
#70234=CARTESIAN_POINT('Ctrl Pts',(6.21377599468721,-1.48514838165934,-6.31023980632529));
#70235=CARTESIAN_POINT('Ctrl Pts',(6.31292987466067,1.71255611161507,-6.25258431622468));
#70236=CARTESIAN_POINT('Ctrl Pts',(6.37903246130962,3.56527434498162,-5.19956251072807));
#70237=CARTESIAN_POINT('Ctrl Pts',(6.4120837546341,4.31013622305522,-4.48350268219026));
#70238=CARTESIAN_POINT('',(6.,4.80478746383271,-4.99805026259201));
#70239=CARTESIAN_POINT('Ctrl Pts',(6.,-6.00216240205939,-1.62981090527766));
#70240=CARTESIAN_POINT('Ctrl Pts',(6.,-5.96859682269621,-1.78822123507159));
#70241=CARTESIAN_POINT('Ctrl Pts',(6.,-5.92885555292031,-1.945098465166));
#70242=CARTESIAN_POINT('Ctrl Pts',(6.,-5.88298849091183,-2.10007140217548));
#70243=CARTESIAN_POINT('Ctrl Pts',(6.,-5.83372654272929,-2.26651478133168));
#70244=CARTESIAN_POINT('Ctrl Pts',(6.,-5.7773991931668,-2.43076229796916));
#70245=CARTESIAN_POINT('Ctrl Pts',(5.99999999999999,-5.71430111965253,-2.59245179083645));
#70246=CARTESIAN_POINT('Ctrl Pts',(5.99999999999999,-5.67435241911292,-2.69482076616652));
#70247=CARTESIAN_POINT('Ctrl Pts',(5.99999999999999,-5.63168865089157,-2.79616427521172));
#70248=CARTESIAN_POINT('Ctrl Pts',(5.99999999999999,-5.58637415866202,-2.89638792850598));
#70249=CARTESIAN_POINT('Ctrl Pts',(5.99999999999999,-5.55452143940101,-2.96683770593091));
#70250=CARTESIAN_POINT('Ctrl Pts',(5.99999999999999,-5.52135881807792,-3.03673411555926));
#70251=CARTESIAN_POINT('Ctrl Pts',(5.99999999999999,-5.48690640354643,-3.10604349782801));
#70252=CARTESIAN_POINT('Ctrl Pts',(5.99999999999999,-5.47044569052808,-3.13915821174632));
#70253=CARTESIAN_POINT('Ctrl Pts',(5.99999999999999,-5.45368794282186,-3.17214368538622));
#70254=CARTESIAN_POINT('Ctrl Pts',(5.99999999999999,-5.43665014407369,-3.20496799833295));
#70255=CARTESIAN_POINT('Ctrl Pts',(5.99999999999999,-5.35517751507704,-3.36192976964539));
#70256=CARTESIAN_POINT('Ctrl Pts',(5.99999999999999,-5.26725451919283,-3.51531432515741));
#70257=CARTESIAN_POINT('Ctrl Pts',(5.99999999999999,-5.17318806361391,-3.66474910658035));
#70258=CARTESIAN_POINT('Ctrl Pts',(5.99999999999999,-5.0788139147758,-3.81467269216468));
#70259=CARTESIAN_POINT('Ctrl Pts',(5.99999999999999,-4.9782557256485,-3.96062128997224));
#70260=CARTESIAN_POINT('Ctrl Pts',(5.99999999999999,-4.87177383449923,-4.10220114978652));
#70261=CARTESIAN_POINT('Ctrl Pts',(5.99999999999999,-4.78110005633049,-4.22276231435077));
#70262=CARTESIAN_POINT('Ctrl Pts',(6.,-4.68612992217677,-4.34015554248365));
#70263=CARTESIAN_POINT('Ctrl Pts',(6.,-4.58699864840819,-4.45412220713425));
#70264=CARTESIAN_POINT('Ctrl Pts',(6.,-4.57093126098927,-4.47259414322636));
#70265=CARTESIAN_POINT('Ctrl Pts',(6.,-4.55475451123802,-4.49097602501803));
#70266=CARTESIAN_POINT('Ctrl Pts',(6.,-4.53846892138093,-4.50926670696808));
#70267=CARTESIAN_POINT('Ctrl Pts',(6.,-4.52235362822714,-4.52736612517732));
#70268=CARTESIAN_POINT('Ctrl Pts',(6.,-4.50613731235933,-4.54536998089995));
#70269=CARTESIAN_POINT('Ctrl Pts',(6.,-4.4898234190663,-4.56327440675413));
#70270=CARTESIAN_POINT('Ctrl Pts',(6.,-4.42090782396902,-4.6389089680727));
#70271=CARTESIAN_POINT('Ctrl Pts',(5.99999999999999,-4.3502361725157,-4.7127864089364));
#70272=CARTESIAN_POINT('Ctrl Pts',(5.99999999999999,-4.27786563021268,-4.7848380789645));
#70273=CARTESIAN_POINT('Ctrl Pts',(5.99999999999999,-4.15309584140503,-4.90905811886697));
#70274=CARTESIAN_POINT('Ctrl Pts',(6.,-4.02327896890847,-5.0278531787929));
#70275=CARTESIAN_POINT('Ctrl Pts',(6.,-3.88886714141271,-5.14107396648211));
#70276=CARTESIAN_POINT('Ctrl Pts',(6.,-3.7527080452692,-5.25576655271977));
#70277=CARTESIAN_POINT('Ctrl Pts',(6.,-3.61183326584496,-5.36473945133278));
#70278=CARTESIAN_POINT('Ctrl Pts',(6.,-3.46666982118827,-5.46780534772134));
#70279=CARTESIAN_POINT('Ctrl Pts',(6.,-3.3185456493242,-5.57297335738167));
#70280=CARTESIAN_POINT('Ctrl Pts',(6.,-3.16595557716371,-5.67199151916148));
#70281=CARTESIAN_POINT('Ctrl Pts',(6.,-3.00931638963617,-5.76461974490931));
#70282=CARTESIAN_POINT('Ctrl Pts',(6.,-2.89183699899052,-5.83409091422019));
#70283=CARTESIAN_POINT('Ctrl Pts',(5.99999999999999,-2.77207915436557,-5.89996693969506));
#70284=CARTESIAN_POINT('Ctrl Pts',(5.99999999999999,-2.65020825097159,-5.96212891564935));
#70285=CARTESIAN_POINT('Ctrl Pts',(5.99999999999999,-2.61706538543952,-5.9790339024254));
#70286=CARTESIAN_POINT('Ctrl Pts',(5.99999999999999,-2.58376620188423,-5.99566411633581));
#70287=CARTESIAN_POINT('Ctrl Pts',(5.99999999999999,-2.55031393882262,-6.01201695390139));
#70288=CARTESIAN_POINT('Ctrl Pts',(5.99999999999999,-2.53181089617986,-6.02106199968047));
#70289=CARTESIAN_POINT('Ctrl Pts',(5.99999999999999,-2.51326444296905,-6.03002048154811));
#70290=CARTESIAN_POINT('Ctrl Pts',(5.99999999999999,-2.49468259592518,-6.03888858495449));
#70291=CARTESIAN_POINT('Ctrl Pts',(5.99999999999999,-2.33019094700295,-6.11739148882));
#70292=CARTESIAN_POINT('Ctrl Pts',(5.99999999999999,-2.16275731640371,-6.18889923399487));
#70293=CARTESIAN_POINT('Ctrl Pts',(5.99999999999999,-1.99283559035297,-6.25323756185287));
#70294=CARTESIAN_POINT('Ctrl Pts',(5.99999999999999,-1.83382494091869,-6.31344457324564));
#70295=CARTESIAN_POINT('Ctrl Pts',(5.99999999999999,-1.6726346722028,-6.3673732853798));
#70296=CARTESIAN_POINT('Ctrl Pts',(5.99999999999999,-1.50961068395816,-6.4148488107241));
#70297=CARTESIAN_POINT('Ctrl Pts',(5.99999999999999,-1.33618843229499,-6.46535249789769));
#70298=CARTESIAN_POINT('Ctrl Pts',(6.,-1.16069077253835,-6.50855444745417));
#70299=CARTESIAN_POINT('Ctrl Pts',(6.,-0.983584177924514,-6.54449336584105));
#70300=CARTESIAN_POINT('Ctrl Pts',(6.,-0.805527961020956,-6.58062498398619));
#70301=CARTESIAN_POINT('Ctrl Pts',(5.99999999999999,-0.625844808076049,
-6.60941559586448));
#70302=CARTESIAN_POINT('Ctrl Pts',(5.99999999999999,-0.444994705161226,
-6.63085379932921));
#70303=CARTESIAN_POINT('Ctrl Pts',(5.99999999999999,-0.352078520882111,
-6.64186820314562));
#70304=CARTESIAN_POINT('Ctrl Pts',(6.,-0.25885414203866,-6.65094100308522));
#70305=CARTESIAN_POINT('Ctrl Pts',(6.,-0.165383456909019,-6.65806532413613));
#70306=CARTESIAN_POINT('Ctrl Pts',(6.,-0.138106596290388,-6.66014436220072));
#70307=CARTESIAN_POINT('Ctrl Pts',(5.99999999999999,-0.110808760073336,
-6.66205744319297));
#70308=CARTESIAN_POINT('Ctrl Pts',(5.99999999999999,-0.0834914876766973,
-6.6638043373535));
#70309=CARTESIAN_POINT('Ctrl Pts',(5.99999999999999,-0.0594801003657474,
-6.66533982565814));
#70310=CARTESIAN_POINT('Ctrl Pts',(5.99999999999999,-0.0354607393562745,
-6.66674643599058));
#70311=CARTESIAN_POINT('Ctrl Pts',(5.99999999999999,-0.0114427696453575,
-6.66802386946623));
#70312=CARTESIAN_POINT('Ctrl Pts',(5.99999999999999,0.17232643902647,-6.67779792371714));
#70313=CARTESIAN_POINT('Ctrl Pts',(5.99999999999999,0.356162228661273,-6.68002334405103));
#70314=CARTESIAN_POINT('Ctrl Pts',(5.99999999999999,0.539578749421798,-6.67477763109705));
#70315=CARTESIAN_POINT('Ctrl Pts',(5.99999999999999,0.724243247873377,-6.66949622597797));
#70316=CARTESIAN_POINT('Ctrl Pts',(6.,0.908483469211453,-6.65664177842282));
#70317=CARTESIAN_POINT('Ctrl Pts',(6.,1.09181827093861,-6.63624254656122));
#70318=CARTESIAN_POINT('Ctrl Pts',(6.,1.27479461914379,-6.61588319897929));
#70319=CARTESIAN_POINT('Ctrl Pts',(6.,1.45686982323424,-6.58800858408027));
#70320=CARTESIAN_POINT('Ctrl Pts',(6.,1.63756918901508,-6.55259533222835));
#70321=CARTESIAN_POINT('Ctrl Pts',(6.,1.68713774842448,-6.54288094352135));
#70322=CARTESIAN_POINT('Ctrl Pts',(5.99999999999999,1.73660276294476,-6.53259898060699));
#70323=CARTESIAN_POINT('Ctrl Pts',(5.99999999999999,1.78595436777605,-6.52174827503316));
#70324=CARTESIAN_POINT('Ctrl Pts',(5.99999999999999,1.92478260633383,-6.49122476223002));
#70325=CARTESIAN_POINT('Ctrl Pts',(6.,2.06271376773678,-6.4562019664384));
#70326=CARTESIAN_POINT('Ctrl Pts',(6.,2.19956587504128,-6.41677751371926));
#70327=CARTESIAN_POINT('Ctrl Pts',(6.,2.25943867198699,-6.39952931565464));
#70328=CARTESIAN_POINT('Ctrl Pts',(6.,2.31910486823453,-6.38143838211038));
#70329=CARTESIAN_POINT('Ctrl Pts',(6.,2.37854887132776,-6.36251183496192));
#70330=CARTESIAN_POINT('Ctrl Pts',(6.,2.41133386438944,-6.35207332670784));
#70331=CARTESIAN_POINT('Ctrl Pts',(6.,2.44405126586026,-6.34138062840303));
#70332=CARTESIAN_POINT('Ctrl Pts',(6.,2.47669842477198,-6.33043485420982));
#70333=CARTESIAN_POINT('Ctrl Pts',(6.,2.49986116879962,-6.32266896663266));
#70334=CARTESIAN_POINT('Ctrl Pts',(6.,2.52298992297603,-6.31477515716261));
#70335=CARTESIAN_POINT('Ctrl Pts',(6.,2.54606625141156,-6.30676003981754));
#70336=CARTESIAN_POINT('Ctrl Pts',(6.,2.72031866926523,-6.24623682527488));
#70337=CARTESIAN_POINT('Ctrl Pts',(6.,2.89180656871482,-6.17872697332531));
#70338=CARTESIAN_POINT('Ctrl Pts',(6.,3.06015974003863,-6.10454067443522));
#70339=CARTESIAN_POINT('Ctrl Pts',(6.,3.23153292294491,-6.02902358100085));
#70340=CARTESIAN_POINT('Ctrl Pts',(6.,3.3996585561246,-5.94658821955142));
#70341=CARTESIAN_POINT('Ctrl Pts',(6.,3.56414018751553,-5.85750818319925));
#70342=CARTESIAN_POINT('Ctrl Pts',(6.,3.72893847172068,-5.76825665387267));
#70343=CARTESIAN_POINT('Ctrl Pts',(6.,3.89007937659884,-5.67233455879464));
#70344=CARTESIAN_POINT('Ctrl Pts',(6.,4.04714827512776,-5.56996716740956));
#70345=CARTESIAN_POINT('Ctrl Pts',(5.99999999999999,4.20261003215418,-5.46864720734118));
#70346=CARTESIAN_POINT('Ctrl Pts',(6.,4.35408329610926,-5.36101281708549));
#70347=CARTESIAN_POINT('Ctrl Pts',(6.,4.5011410535457,-5.24723848450609));
#70348=CARTESIAN_POINT('Ctrl Pts',(6.,4.6045951656092,-5.16719903090768));
#70349=CARTESIAN_POINT('Ctrl Pts',(6.,4.70586353074338,-5.08411998909903));
#70350=CARTESIAN_POINT('Ctrl Pts',(6.,4.80478746383271,-4.99805026259201));
#70351=CARTESIAN_POINT('Ctrl Pts',(6.,4.80478746383271,-4.99805026259201));
#70352=CARTESIAN_POINT('Ctrl Pts',(5.96694870667552,3.97444177895361,-5.79628844103034));
#70353=CARTESIAN_POINT('Ctrl Pts',(5.93389741335104,2.94176938984478,-6.38322417906209));
#70354=CARTESIAN_POINT('Ctrl Pts',(5.90084612002656,1.83131854449184,-6.68740409837522));
#70355=CARTESIAN_POINT('Ctrl Pts',(5.86779482670209,0.720867699138943,-6.99158401768835));
#70356=CARTESIAN_POINT('Ctrl Pts',(5.83474353337761,-0.467361602457999,
-7.01300811828287));
#70357=CARTESIAN_POINT('Ctrl Pts',(5.80169224005313,-1.58829921867574,-6.74922313565156));
#70358=CARTESIAN_POINT('Ctrl Pts',(5.76864094672865,-2.7092368348935,-6.48543815302024));
#70359=CARTESIAN_POINT('Ctrl Pts',(5.73558965340417,-3.76288276573208,-5.93644408716305));
#70360=CARTESIAN_POINT('Ctrl Pts',(5.70253836007969,-4.62129214226549,-5.16896427511983));
#70361=CARTESIAN_POINT('Ctrl Pts',(5.66948706675521,-5.47970151879887,-4.40148446307664));
#70362=CARTESIAN_POINT('Ctrl Pts',(5.63643577343074,-6.14287434102713,-3.41551890484744));
#70363=CARTESIAN_POINT('Ctrl Pts',(5.60338448010626,-6.53001704429179,-2.33104349458117));
#70364=CARTESIAN_POINT('Ctrl Pts',(5.58064687460627,-6.79635149518946,-1.58497967762262));
#70365=CARTESIAN_POINT('Ctrl Pts',(5.55790926910627,-6.93204810038981,-0.792293720665733));
#70366=CARTESIAN_POINT('Ctrl Pts',(5.53517166360628,-6.93272540515737,0.000163154062267218));
#70367=CARTESIAN_POINT('Origin',(10.5,5.,0.));
#70368=CARTESIAN_POINT('Origin',(10.5,5.,0.));
#70369=CARTESIAN_POINT('Origin',(-13.9,0.,0.));
#70370=CARTESIAN_POINT('',(-13.9,-6.65,-8.1439012143299E-16));
#70371=CARTESIAN_POINT('Origin',(-3.775,0.,0.));
#70372=CARTESIAN_POINT('Origin',(6.,0.,0.));
#70373=CARTESIAN_POINT('Origin',(6.,11.5,0.));
#70374=CARTESIAN_POINT('',(6.,-11.5,-1.40834381901946E-15));
#70375=CARTESIAN_POINT('Origin',(6.,0.,0.));
#70376=CARTESIAN_POINT('Origin',(6.25,0.,0.));
#70377=CARTESIAN_POINT('',(6.25,-11.75,-1.43895998899814E-15));
#70378=CARTESIAN_POINT('Origin',(14.75,0.,0.));
#70379=CARTESIAN_POINT('',(15.,-11.5,-1.40834381901946E-15));
#70380=CARTESIAN_POINT('Origin',(15.,0.,0.));
#70381=CARTESIAN_POINT('',(14.75,-11.75,-1.43895998899814E-15));
#70382=CARTESIAN_POINT('Origin',(15.,8.,0.));
#70383=CARTESIAN_POINT('',(15.,-8.,-9.79717439317883E-16));
#70384=CARTESIAN_POINT('Origin',(15.,0.,0.));
#70385=CARTESIAN_POINT('Origin',(15.8,0.,0.));
#70386=CARTESIAN_POINT('',(16.6,-8.,-9.79717439317883E-16));
#70387=CARTESIAN_POINT('Origin',(16.6,0.,0.));
#70388=CARTESIAN_POINT('',(15.8,-8.,-9.79717439317883E-16));
#70389=CARTESIAN_POINT('Origin',(16.8,0.,0.));
#70390=CARTESIAN_POINT('',(16.8,-7.8,-9.55224503334935E-16));
#82359=UNCERTAINTY_MEASURE_WITH_UNIT(LENGTH_MEASURE(0.01),#82385,
'DISTANCE_ACCURACY_VALUE',
'Maximum model space distance between geometric entities at asserted c
onnectivities');
#82363=UNCERTAINTY_MEASURE_WITH_UNIT(LENGTH_MEASURE(0.01),#82385,
'DISTANCE_ACCURACY_VALUE',
'Maximum model space distance between geometric entities at asserted c
onnectivities');
#82380=(
GEOMETRIC_REPRESENTATION_CONTEXT(3)
GLOBAL_UNCERTAINTY_ASSIGNED_CONTEXT((#82359))
GLOBAL_UNIT_ASSIGNED_CONTEXT((#82385,#82387,#82388))
REPRESENTATION_CONTEXT('','3D')
);
#82384=(
GEOMETRIC_REPRESENTATION_CONTEXT(3)
GLOBAL_UNCERTAINTY_ASSIGNED_CONTEXT((#82363))
GLOBAL_UNIT_ASSIGNED_CONTEXT((#82385,#82387,#82388))
REPRESENTATION_CONTEXT('','3D')
);
#82385=(
LENGTH_UNIT()
NAMED_UNIT(*)
SI_UNIT(.MILLI.,.METRE.)
);
#82387=(
NAMED_UNIT(*)
PLANE_ANGLE_UNIT()
SI_UNIT($,.RADIAN.)
);
#82388=(
NAMED_UNIT(*)
SI_UNIT($,.STERADIAN.)
SOLID_ANGLE_UNIT()
);
#82405=SHAPE_DEFINITION_REPRESENTATION(#82425,#82481);
#82425=PRODUCT_DEFINITION_SHAPE('',$,#82502);
#82481=SHAPE_REPRESENTATION('',(#32907),#82380);
#82485=PRODUCT_DEFINITION_CONTEXT('part definition',#82547,'design');
#82502=PRODUCT_DEFINITION('2026-10-20-12-38-17-430',
'07_AJS_Bushing_M14x1.25_Brass',#82522,#82485);
#82522=PRODUCT_DEFINITION_FORMATION('',$,#82565);
#82547=APPLICATION_CONTEXT(
'Core Data for Automotive Mechanical Design Process');
#82548=PRODUCT_CONTEXT('part definition',#82547,'mechanical');
#82565=PRODUCT('2026-10-20-12-38-17-430',
'07_AJS_Bushing_M14x1.25_Brass',$,(#82548));
#82639=COLOUR_RGB('Off White',0.89,0.88,0.83);
#82640=FILL_AREA_STYLE_COLOUR('',#82639);
#82641=FILL_AREA_STYLE('',(#82640));
#82642=SURFACE_STYLE_FILL_AREA(#82641);
#82643=SURFACE_SIDE_STYLE('',(#82642));
#82644=SURFACE_STYLE_USAGE(.BOTH.,#82643);
#82645=PRESENTATION_STYLE_ASSIGNMENT((#82644));
ENDSEC;
END-ISO-10303-21;
